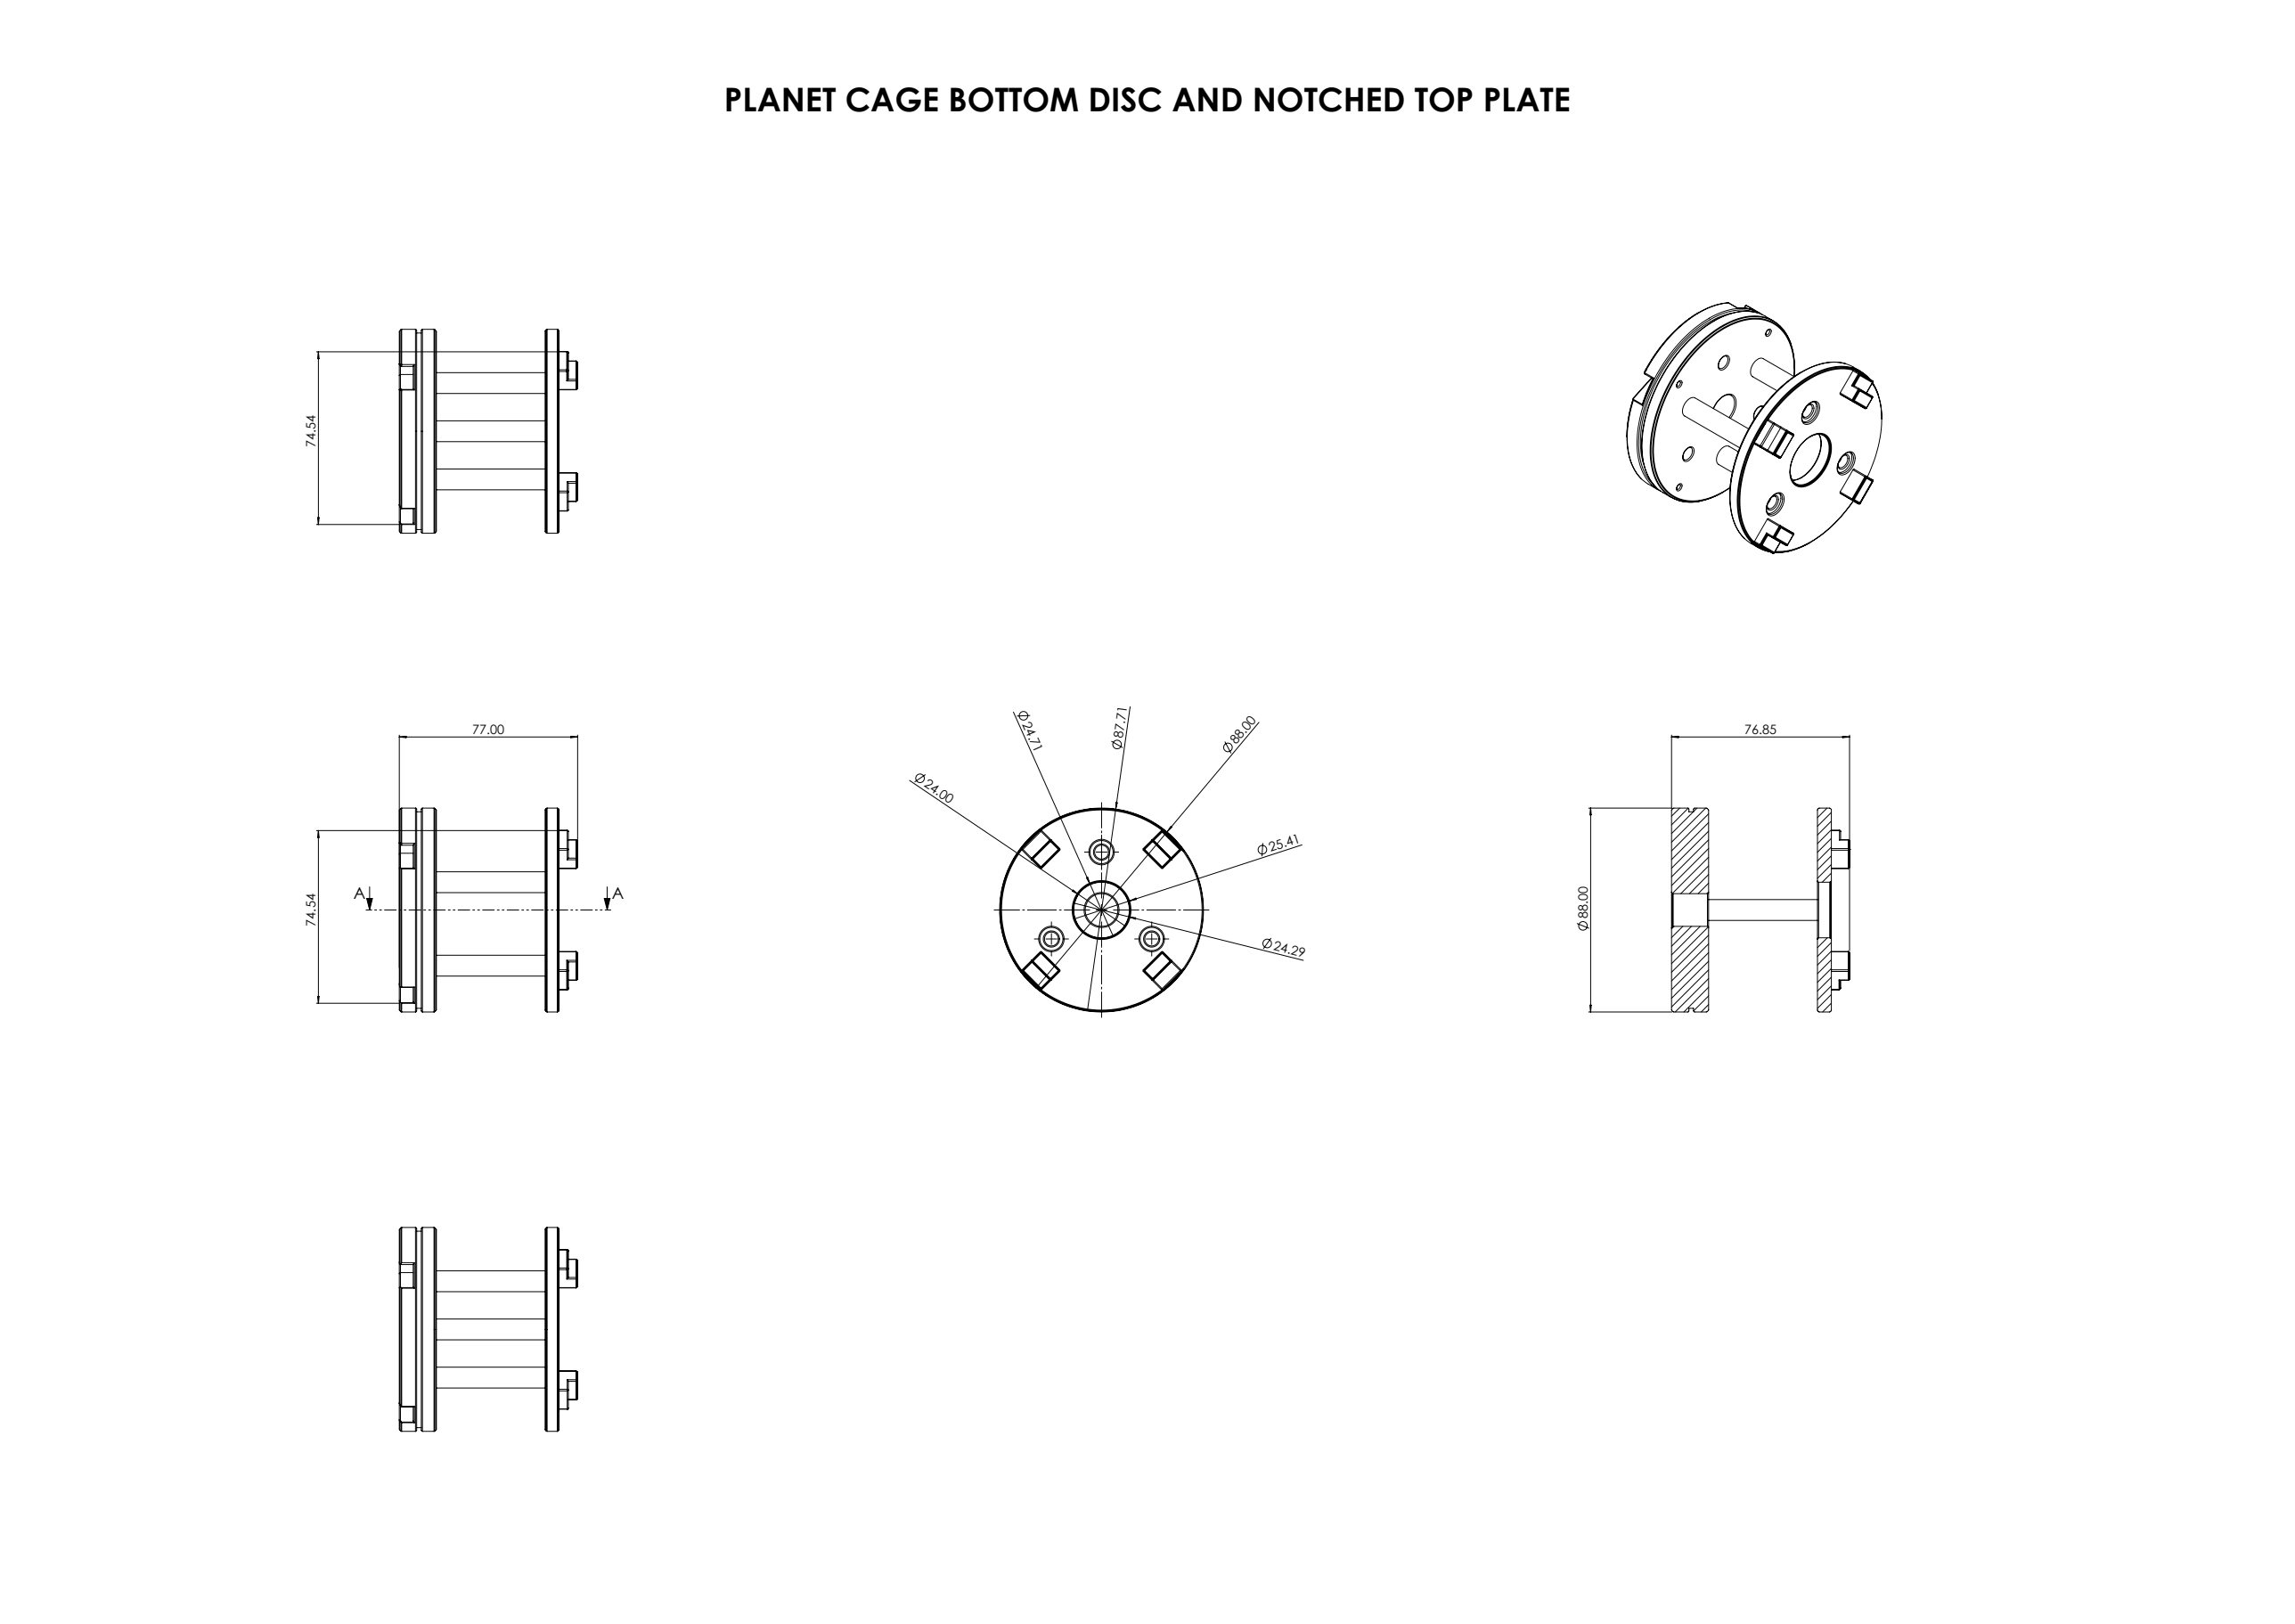
ISO-10303-21;
HEADER;
/* Generated by software containing ST-Developer
 * from STEP Tools, Inc. (www.steptools.com) 
 */

FILE_DESCRIPTION(
/* description */ (''),
/* implementation_level */ '2;1');

FILE_NAME(
/* name */ '02_Planet_Cage_Bottom_Disc_and_Notched_Top_Plate.step',
/* time_stamp */ '2026-10-11T13:00:10-07:00',
/* author */ (''),
/* organization */ (''),
/* preprocessor_version */ 'ST-DEVELOPER v20.2',
/* originating_system */ 'Autodesk Translation Framework v15.15.0.0',
/* authorisation */ '');

FILE_SCHEMA (('AUTOMOTIVE_DESIGN { 1 0 10303 214 3 1 1 }'));
ENDSEC;

DATA;
#10=MECHANICAL_DESIGN_GEOMETRIC_PRESENTATION_REPRESENTATION('',(#359),#65563);
#95=TOROIDAL_SURFACE('',#20843,43.5,0.5);
#96=TOROIDAL_SURFACE('',#20862,3.5,0.5);
#97=TOROIDAL_SURFACE('',#20886,42.9928932188135,0.5);
#98=TOROIDAL_SURFACE('',#20891,43.5,0.5);
#99=TOROIDAL_SURFACE('',#20897,3.5,0.5);
#100=TOROIDAL_SURFACE('',#20902,42.9928932188135,0.5);
#101=TOROIDAL_SURFACE('',#20905,42.9928932188135,0.5);
#102=TOROIDAL_SURFACE('',#20926,43.5,0.5);
#103=TOROIDAL_SURFACE('',#20929,43.5,0.5);
#104=TOROIDAL_SURFACE('',#20951,43.5,0.5);
#105=TOROIDAL_SURFACE('',#20956,43.5,0.5);
#106=TOROIDAL_SURFACE('',#20967,42.9928932188135,0.5);
#107=TOROIDAL_SURFACE('',#20971,3.5,0.5);
#108=TOROIDAL_SURFACE('',#20981,3.5,0.5);
#109=TOROIDAL_SURFACE('',#20985,1.75,0.5);
#110=TOROIDAL_SURFACE('',#21020,43.5,0.5);
#111=TOROIDAL_SURFACE('',#21025,1.75,0.5);
#112=TOROIDAL_SURFACE('',#21059,43.5,0.5);
#113=TOROIDAL_SURFACE('',#21069,43.5,0.5);
#114=TOROIDAL_SURFACE('',#21076,43.5,0.5);
#115=TOROIDAL_SURFACE('',#21081,43.5,0.5);
#116=TOROIDAL_SURFACE('',#21097,1.75,0.5);
#117=TOROIDAL_SURFACE('',#21103,1.75,0.5);
#118=TOROIDAL_SURFACE('',#21109,3.5,0.5);
#119=TOROIDAL_SURFACE('',#21128,3.5,0.5);
#120=TOROIDAL_SURFACE('',#21134,42.9928932188134,0.5);
#121=TOROIDAL_SURFACE('',#21136,1.75,0.5);
#122=TOROIDAL_SURFACE('',#21138,1.75,0.5);
#123=TOROIDAL_SURFACE('',#21140,3.5,0.5);
#124=TOROIDAL_SURFACE('',#21146,1.75,0.5);
#125=TOROIDAL_SURFACE('',#21148,1.75,0.5);
#126=TOROIDAL_SURFACE('',#21150,3.5,0.5);
#127=TOROIDAL_SURFACE('',#21158,3.5,0.5);
#128=TOROIDAL_SURFACE('',#21166,3.5,0.5);
#129=TOROIDAL_SURFACE('',#21183,43.5,0.5);
#130=TOROIDAL_SURFACE('',#21195,43.1928932188135,0.5);
#131=TOROIDAL_SURFACE('',#21206,3.5,0.5);
#132=TOROIDAL_SURFACE('',#21208,3.5,0.5);
#133=TOROIDAL_SURFACE('',#21210,3.5,0.5);
#134=TOROIDAL_SURFACE('',#21212,7.55,0.5);
#135=TOROIDAL_SURFACE('',#21219,7.75710678118654,0.5);
#136=TOROIDAL_SURFACE('',#21226,7.55,0.5);
#137=TOROIDAL_SURFACE('',#21228,12.5,0.5);
#138=TOROIDAL_SURFACE('',#21235,43.5,0.5);
#139=TOROIDAL_SURFACE('',#21243,43.1928932188135,0.5);
#140=TOROIDAL_SURFACE('',#21251,5.5,0.5);
#141=TOROIDAL_SURFACE('',#21261,5.5,0.5);
#142=TOROIDAL_SURFACE('',#21266,5.5,0.5);
#143=TOROIDAL_SURFACE('',#21271,12.5,0.5);
#144=TOROIDAL_SURFACE('',#21278,12.7071067811865,0.5);
#200=ELLIPSE('',#20602,0.707106781186548,0.5);
#201=ELLIPSE('',#20603,0.707106781186549,0.5);
#202=ELLIPSE('',#20642,0.707106781186549,0.5);
#203=ELLIPSE('',#20643,0.707106781186543,0.5);
#204=ELLIPSE('',#20698,0.707106781186547,0.5);
#205=ELLIPSE('',#20715,0.707106781186547,0.5);
#206=ELLIPSE('',#20745,1.08766387358053,0.5);
#207=ELLIPSE('',#20747,0.563016250305246,0.5);
#208=ELLIPSE('',#20752,0.70710678118655,0.499999999999999);
#209=ELLIPSE('',#20753,0.707106781186547,0.5);
#210=ELLIPSE('',#20756,0.707106781186549,0.5);
#211=ELLIPSE('',#20759,0.707106781186548,0.5);
#212=ELLIPSE('',#20790,0.524647623275289,0.499999999999999);
#213=ELLIPSE('',#20791,1.08766387358054,0.499999999999999);
#214=ELLIPSE('',#20799,0.541196100146196,0.5);
#215=ELLIPSE('',#20808,0.707106781186548,0.5);
#216=ELLIPSE('',#20818,0.541196100146196,0.5);
#217=ELLIPSE('',#20819,0.707106781186546,0.5);
#218=ELLIPSE('',#20822,0.999999999999998,0.499999999999999);
#219=ELLIPSE('',#20832,0.707106781186548,0.5);
#220=ELLIPSE('',#20901,0.707106781186546,0.5);
#221=ELLIPSE('',#20996,0.707106781186545,0.5);
#222=ELLIPSE('',#21001,0.563016250305243,0.5);
#223=ELLIPSE('',#21002,0.563016250305246,0.5);
#224=ELLIPSE('',#21003,0.707106781186547,0.5);
#225=ELLIPSE('',#21004,0.707106781186543,0.5);
#226=ELLIPSE('',#21007,0.563016250305245,0.499999999999997);
#227=ELLIPSE('',#21010,0.563016250305245,0.499999999999999);
#228=ELLIPSE('',#21017,0.999999999999989,0.499999999999997);
#229=ELLIPSE('',#21019,0.707106781186552,0.5);
#230=ELLIPSE('',#21057,0.707106781186546,0.5);
#231=ELLIPSE('',#21087,0.541196100146194,0.5);
#232=ELLIPSE('',#21096,0.707106781186549,0.5);
#243=SPHERICAL_SURFACE('',#20559,0.5);
#244=SPHERICAL_SURFACE('',#20569,0.5);
#245=SPHERICAL_SURFACE('',#20571,0.5);
#246=SPHERICAL_SURFACE('',#20581,0.5);
#247=SPHERICAL_SURFACE('',#20595,0.5);
#248=SPHERICAL_SURFACE('',#20605,0.5);
#249=SPHERICAL_SURFACE('',#20612,0.5);
#250=SPHERICAL_SURFACE('',#20617,0.5);
#251=SPHERICAL_SURFACE('',#20631,0.5);
#252=SPHERICAL_SURFACE('',#20637,0.5);
#253=SPHERICAL_SURFACE('',#20646,0.5);
#254=SPHERICAL_SURFACE('',#20654,0.5);
#255=SPHERICAL_SURFACE('',#20665,0.5);
#256=SPHERICAL_SURFACE('',#20674,0.5);
#257=SPHERICAL_SURFACE('',#20679,0.5);
#258=SPHERICAL_SURFACE('',#20683,0.5);
#259=SPHERICAL_SURFACE('',#20702,0.5);
#260=SPHERICAL_SURFACE('',#20708,0.5);
#261=SPHERICAL_SURFACE('',#20722,0.5);
#262=SPHERICAL_SURFACE('',#20726,0.5);
#263=SPHERICAL_SURFACE('',#20732,0.5);
#264=SPHERICAL_SURFACE('',#20737,0.5);
#265=SPHERICAL_SURFACE('',#20748,0.5);
#266=SPHERICAL_SURFACE('',#20764,0.5);
#267=SPHERICAL_SURFACE('',#20768,0.5);
#268=SPHERICAL_SURFACE('',#20784,0.5);
#269=SPHERICAL_SURFACE('',#20787,0.5);
#270=SPHERICAL_SURFACE('',#20809,0.5);
#271=SPHERICAL_SURFACE('',#20824,0.5);
#272=SPHERICAL_SURFACE('',#20827,0.5);
#273=SPHERICAL_SURFACE('',#20836,0.5);
#274=SPHERICAL_SURFACE('',#20841,0.5);
#275=SPHERICAL_SURFACE('',#20868,0.5);
#276=SPHERICAL_SURFACE('',#20871,0.5);
#277=SPHERICAL_SURFACE('',#20914,0.5);
#278=SPHERICAL_SURFACE('',#20920,0.5);
#279=SPHERICAL_SURFACE('',#20934,0.5);
#280=SPHERICAL_SURFACE('',#20936,0.5);
#281=SPHERICAL_SURFACE('',#20946,0.5);
#282=SPHERICAL_SURFACE('',#20949,0.5);
#283=SPHERICAL_SURFACE('',#20961,0.500000000000003);
#284=SPHERICAL_SURFACE('',#20975,0.5);
#285=SPHERICAL_SURFACE('',#20991,0.5);
#286=SPHERICAL_SURFACE('',#21034,0.5);
#287=SPHERICAL_SURFACE('',#21038,0.5);
#288=SPHERICAL_SURFACE('',#21042,0.5);
#289=SPHERICAL_SURFACE('',#21053,0.5);
#290=SPHERICAL_SURFACE('',#21092,0.5);
#291=SPHERICAL_SURFACE('',#21178,0.5);
#337=SHAPE_REPRESENTATION_RELATIONSHIP('SRR','None',#65615,#348);
#348=ADVANCED_BREP_SHAPE_REPRESENTATION('',(#370),#65553);
#359=STYLED_ITEM('',(#65802),#370);
#370=MANIFOLD_SOLID_BREP('Body1',#20009);
#414=CONICAL_SURFACE('',#20889,43.6,0.785398163397448);
#415=CONICAL_SURFACE('',#20908,43.6,0.785398163397448);
#416=CONICAL_SURFACE('',#20924,43.6,0.785398163397448);
#417=CONICAL_SURFACE('',#20954,43.6,0.785398163397448);
#418=CONICAL_SURFACE('',#21073,43.6,0.785398163397454);
#419=CONICAL_SURFACE('',#21189,43.7,0.785398163397452);
#420=CONICAL_SURFACE('',#21223,7.3,0.785398163397442);
#421=CONICAL_SURFACE('',#21239,43.7,0.785398163397452);
#422=CONICAL_SURFACE('',#21275,12.25,0.785398163397448);
#668=(
BOUNDED_CURVE()
B_SPLINE_CURVE(2,(#48216,#48217,#48218),.UNSPECIFIED.,.F.,.F.)
B_SPLINE_CURVE_WITH_KNOTS((3,3),(0.026389951333147,0.0542823820564139),
 .UNSPECIFIED.)
CURVE()
GEOMETRIC_REPRESENTATION_ITEM()
RATIONAL_B_SPLINE_CURVE((1.00002935554076,1.00004146705942,1.00004638738564))
REPRESENTATION_ITEM('')
);
#669=(
BOUNDED_CURVE()
B_SPLINE_CURVE(2,(#48349,#48350,#48351),.UNSPECIFIED.,.F.,.F.)
B_SPLINE_CURVE_WITH_KNOTS((3,3),(0.0263899513331846,0.0542823820564278),
 .UNSPECIFIED.)
CURVE()
GEOMETRIC_REPRESENTATION_ITEM()
RATIONAL_B_SPLINE_CURVE((1.00002935553973,1.00004146705796,1.00004638738401))
REPRESENTATION_ITEM('')
);
#670=(
BOUNDED_CURVE()
B_SPLINE_CURVE(2,(#49013,#49014,#49015),.UNSPECIFIED.,.F.,.F.)
B_SPLINE_CURVE_WITH_KNOTS((3,3),(0.355039941373883,0.455385686797418),
 .UNSPECIFIED.)
CURVE()
GEOMETRIC_REPRESENTATION_ITEM()
RATIONAL_B_SPLINE_CURVE((1.00817025780825,1.00909081812274,1.00987909016891))
REPRESENTATION_ITEM('')
);
#671=(
BOUNDED_CURVE()
B_SPLINE_CURVE(2,(#49128,#49129,#49130),.UNSPECIFIED.,.F.,.F.)
B_SPLINE_CURVE_WITH_KNOTS((3,3),(1.65125508748907,1.7516008329126),
 .UNSPECIFIED.)
CURVE()
GEOMETRIC_REPRESENTATION_ITEM()
RATIONAL_B_SPLINE_CURVE((1.00987909016891,1.00909081812274,1.00817025780825))
REPRESENTATION_ITEM('')
);
#838=B_SPLINE_SURFACE_WITH_KNOTS('',3,3,((#48066,#48067,#48068,#48069),
(#48070,#48071,#48072,#48073),(#48074,#48075,#48076,#48077),(#48078,#48079,
#48080,#48081),(#48082,#48083,#48084,#48085),(#48086,#48087,#48088,#48089),
(#48090,#48091,#48092,#48093)),.UNSPECIFIED.,.F.,.F.,.F.,(4,1,1,1,4),(4,
4),(0.,0.285714285714286,0.571428571428571,0.857142857142857,1.),(0.363335998515663,
0.499634934734419),.UNSPECIFIED.);
#839=B_SPLINE_SURFACE_WITH_KNOTS('',3,3,((#48278,#48279,#48280,#48281),
(#48282,#48283,#48284,#48285),(#48286,#48287,#48288,#48289),(#48290,#48291,
#48292,#48293),(#48294,#48295,#48296,#48297),(#48298,#48299,#48300,#48301),
(#48302,#48303,#48304,#48305)),.UNSPECIFIED.,.F.,.F.,.F.,(4,1,1,1,4),(4,
4),(0.,0.285714285714286,0.571428571428571,0.857142857142857,1.),(0.,0.136299039595008),
 .UNSPECIFIED.);
#840=B_SPLINE_SURFACE_WITH_KNOTS('',3,3,((#48415,#48416,#48417,#48418),
(#48419,#48420,#48421,#48422),(#48423,#48424,#48425,#48426),(#48427,#48428,
#48429,#48430)),.UNSPECIFIED.,.F.,.F.,.F.,(4,4),(4,4),(0.,1.),(0.,0.0923903836946144),
 .UNSPECIFIED.);
#841=B_SPLINE_SURFACE_WITH_KNOTS('',3,3,((#48482,#48483,#48484,#48485),
(#48486,#48487,#48488,#48489),(#48490,#48491,#48492,#48493),(#48494,#48495,
#48496,#48497)),.UNSPECIFIED.,.F.,.F.,.F.,(4,4),(4,4),(0.,1.),(0.,0.0923903843306348),
 .UNSPECIFIED.);
#842=B_SPLINE_SURFACE_WITH_KNOTS('',3,3,((#48548,#48549,#48550,#48551),
(#48552,#48553,#48554,#48555),(#48556,#48557,#48558,#48559),(#48560,#48561,
#48562,#48563),(#48564,#48565,#48566,#48567),(#48568,#48569,#48570,#48571),
(#48572,#48573,#48574,#48575)),.UNSPECIFIED.,.F.,.F.,.F.,(4,1,1,1,4),(4,
4),(0.,0.285714285714286,0.571428571428571,0.857142857142857,1.),(0.,0.136298877173929),
 .UNSPECIFIED.);
#893=PLANE('',#20585);
#894=PLANE('',#20588);
#895=PLANE('',#20591);
#896=PLANE('',#20597);
#897=PLANE('',#20600);
#898=PLANE('',#20607);
#899=PLANE('',#20616);
#900=PLANE('',#20633);
#901=PLANE('',#20636);
#902=PLANE('',#20640);
#903=PLANE('',#20650);
#904=PLANE('',#20651);
#905=PLANE('',#20658);
#906=PLANE('',#20669);
#907=PLANE('',#20670);
#908=PLANE('',#20687);
#909=PLANE('',#20690);
#910=PLANE('',#20693);
#911=PLANE('',#20704);
#912=PLANE('',#20707);
#913=PLANE('',#20711);
#914=PLANE('',#20727);
#915=PLANE('',#20728);
#916=PLANE('',#20736);
#917=PLANE('',#20750);
#918=PLANE('',#20754);
#919=PLANE('',#20778);
#920=PLANE('',#20794);
#921=PLANE('',#20797);
#922=PLANE('',#20802);
#923=PLANE('',#20805);
#924=PLANE('',#20813);
#925=PLANE('',#20815);
#926=PLANE('',#20816);
#927=PLANE('',#20820);
#928=PLANE('',#20831);
#929=PLANE('',#20842);
#930=PLANE('',#20858);
#931=PLANE('',#20877);
#932=PLANE('',#20907);
#933=PLANE('',#20923);
#934=PLANE('',#20928);
#935=PLANE('',#20931);
#936=PLANE('',#20940);
#937=PLANE('',#20958);
#938=PLANE('',#20977);
#939=PLANE('',#20978);
#940=PLANE('',#20997);
#941=PLANE('',#21008);
#942=PLANE('',#21015);
#943=PLANE('',#21016);
#944=PLANE('',#21022);
#945=PLANE('',#21048);
#946=PLANE('',#21055);
#947=PLANE('',#21058);
#948=PLANE('',#21067);
#949=PLANE('',#21078);
#950=PLANE('',#21083);
#951=PLANE('',#21089);
#952=PLANE('',#21094);
#953=PLANE('',#21114);
#954=PLANE('',#21156);
#955=PLANE('',#21164);
#956=PLANE('',#21172);
#957=PLANE('',#21180);
#958=PLANE('',#21198);
#959=PLANE('',#21256);
#960=PLANE('',#21280);
#961=PLANE('',#21284);
#962=PLANE('',#21285);
#963=PLANE('',#21286);
#964=PLANE('',#21287);
#965=PLANE('',#21288);
#966=PLANE('',#21289);
#967=PLANE('',#21290);
#968=PLANE('',#21291);
#969=PLANE('',#21292);
#970=PLANE('',#21293);
#1083=FACE_BOUND('',#2757,.T.);
#1084=FACE_BOUND('',#2765,.T.);
#1085=FACE_BOUND('',#2804,.T.);
#1086=FACE_BOUND('',#2834,.T.);
#1087=FACE_BOUND('',#2854,.T.);
#1088=FACE_BOUND('',#2859,.T.);
#1089=FACE_BOUND('',#2862,.T.);
#1090=FACE_BOUND('',#2876,.T.);
#1091=FACE_BOUND('',#2877,.T.);
#1092=FACE_BOUND('',#2878,.T.);
#1093=FACE_BOUND('',#2879,.T.);
#1094=FACE_BOUND('',#2880,.T.);
#1095=FACE_BOUND('',#2881,.T.);
#1096=FACE_BOUND('',#2882,.T.);
#1097=FACE_BOUND('',#2883,.T.);
#1098=FACE_BOUND('',#2884,.T.);
#1099=FACE_BOUND('',#2885,.T.);
#1100=FACE_BOUND('',#2886,.T.);
#1101=FACE_BOUND('',#2900,.T.);
#1102=FACE_BOUND('',#2904,.T.);
#1103=FACE_BOUND('',#2908,.T.);
#1104=FACE_BOUND('',#2919,.T.);
#1105=FACE_BOUND('',#2920,.T.);
#1106=FACE_BOUND('',#2921,.T.);
#1107=FACE_BOUND('',#2922,.T.);
#1108=FACE_BOUND('',#2923,.T.);
#1109=FACE_BOUND('',#2924,.T.);
#1110=FACE_BOUND('',#2925,.T.);
#1111=FACE_BOUND('',#2941,.T.);
#1112=FACE_BOUND('',#2942,.T.);
#1113=FACE_BOUND('',#2943,.T.);
#1114=FACE_BOUND('',#2944,.T.);
#1425=FACE_OUTER_BOUND('',#2612,.T.);
#1426=FACE_OUTER_BOUND('',#2613,.T.);
#1427=FACE_OUTER_BOUND('',#2614,.T.);
#1428=FACE_OUTER_BOUND('',#2615,.T.);
#1429=FACE_OUTER_BOUND('',#2616,.T.);
#1430=FACE_OUTER_BOUND('',#2617,.T.);
#1431=FACE_OUTER_BOUND('',#2618,.T.);
#1432=FACE_OUTER_BOUND('',#2619,.T.);
#1433=FACE_OUTER_BOUND('',#2620,.T.);
#1434=FACE_OUTER_BOUND('',#2621,.T.);
#1435=FACE_OUTER_BOUND('',#2622,.T.);
#1436=FACE_OUTER_BOUND('',#2623,.T.);
#1437=FACE_OUTER_BOUND('',#2624,.T.);
#1438=FACE_OUTER_BOUND('',#2625,.T.);
#1439=FACE_OUTER_BOUND('',#2626,.T.);
#1440=FACE_OUTER_BOUND('',#2627,.T.);
#1441=FACE_OUTER_BOUND('',#2628,.T.);
#1442=FACE_OUTER_BOUND('',#2629,.T.);
#1443=FACE_OUTER_BOUND('',#2630,.T.);
#1444=FACE_OUTER_BOUND('',#2631,.T.);
#1445=FACE_OUTER_BOUND('',#2632,.T.);
#1446=FACE_OUTER_BOUND('',#2633,.T.);
#1447=FACE_OUTER_BOUND('',#2634,.T.);
#1448=FACE_OUTER_BOUND('',#2635,.T.);
#1449=FACE_OUTER_BOUND('',#2636,.T.);
#1450=FACE_OUTER_BOUND('',#2637,.T.);
#1451=FACE_OUTER_BOUND('',#2638,.T.);
#1452=FACE_OUTER_BOUND('',#2639,.T.);
#1453=FACE_OUTER_BOUND('',#2640,.T.);
#1454=FACE_OUTER_BOUND('',#2641,.T.);
#1455=FACE_OUTER_BOUND('',#2642,.T.);
#1456=FACE_OUTER_BOUND('',#2643,.T.);
#1457=FACE_OUTER_BOUND('',#2644,.T.);
#1458=FACE_OUTER_BOUND('',#2645,.T.);
#1459=FACE_OUTER_BOUND('',#2646,.T.);
#1460=FACE_OUTER_BOUND('',#2647,.T.);
#1461=FACE_OUTER_BOUND('',#2648,.T.);
#1462=FACE_OUTER_BOUND('',#2649,.T.);
#1463=FACE_OUTER_BOUND('',#2650,.T.);
#1464=FACE_OUTER_BOUND('',#2651,.T.);
#1465=FACE_OUTER_BOUND('',#2652,.T.);
#1466=FACE_OUTER_BOUND('',#2653,.T.);
#1467=FACE_OUTER_BOUND('',#2654,.T.);
#1468=FACE_OUTER_BOUND('',#2655,.T.);
#1469=FACE_OUTER_BOUND('',#2656,.T.);
#1470=FACE_OUTER_BOUND('',#2657,.T.);
#1471=FACE_OUTER_BOUND('',#2658,.T.);
#1472=FACE_OUTER_BOUND('',#2659,.T.);
#1473=FACE_OUTER_BOUND('',#2660,.T.);
#1474=FACE_OUTER_BOUND('',#2661,.T.);
#1475=FACE_OUTER_BOUND('',#2662,.T.);
#1476=FACE_OUTER_BOUND('',#2663,.T.);
#1477=FACE_OUTER_BOUND('',#2664,.T.);
#1478=FACE_OUTER_BOUND('',#2665,.T.);
#1479=FACE_OUTER_BOUND('',#2666,.T.);
#1480=FACE_OUTER_BOUND('',#2667,.T.);
#1481=FACE_OUTER_BOUND('',#2668,.T.);
#1482=FACE_OUTER_BOUND('',#2669,.T.);
#1483=FACE_OUTER_BOUND('',#2670,.T.);
#1484=FACE_OUTER_BOUND('',#2671,.T.);
#1485=FACE_OUTER_BOUND('',#2672,.T.);
#1486=FACE_OUTER_BOUND('',#2673,.T.);
#1487=FACE_OUTER_BOUND('',#2674,.T.);
#1488=FACE_OUTER_BOUND('',#2675,.T.);
#1489=FACE_OUTER_BOUND('',#2676,.T.);
#1490=FACE_OUTER_BOUND('',#2677,.T.);
#1491=FACE_OUTER_BOUND('',#2678,.T.);
#1492=FACE_OUTER_BOUND('',#2679,.T.);
#1493=FACE_OUTER_BOUND('',#2680,.T.);
#1494=FACE_OUTER_BOUND('',#2681,.T.);
#1495=FACE_OUTER_BOUND('',#2682,.T.);
#1496=FACE_OUTER_BOUND('',#2683,.T.);
#1497=FACE_OUTER_BOUND('',#2684,.T.);
#1498=FACE_OUTER_BOUND('',#2685,.T.);
#1499=FACE_OUTER_BOUND('',#2686,.T.);
#1500=FACE_OUTER_BOUND('',#2687,.T.);
#1501=FACE_OUTER_BOUND('',#2688,.T.);
#1502=FACE_OUTER_BOUND('',#2689,.T.);
#1503=FACE_OUTER_BOUND('',#2690,.T.);
#1504=FACE_OUTER_BOUND('',#2691,.T.);
#1505=FACE_OUTER_BOUND('',#2692,.T.);
#1506=FACE_OUTER_BOUND('',#2693,.T.);
#1507=FACE_OUTER_BOUND('',#2694,.T.);
#1508=FACE_OUTER_BOUND('',#2695,.T.);
#1509=FACE_OUTER_BOUND('',#2696,.T.);
#1510=FACE_OUTER_BOUND('',#2697,.T.);
#1511=FACE_OUTER_BOUND('',#2698,.T.);
#1512=FACE_OUTER_BOUND('',#2699,.T.);
#1513=FACE_OUTER_BOUND('',#2700,.T.);
#1514=FACE_OUTER_BOUND('',#2701,.T.);
#1515=FACE_OUTER_BOUND('',#2702,.T.);
#1516=FACE_OUTER_BOUND('',#2703,.T.);
#1517=FACE_OUTER_BOUND('',#2704,.T.);
#1518=FACE_OUTER_BOUND('',#2705,.T.);
#1519=FACE_OUTER_BOUND('',#2706,.T.);
#1520=FACE_OUTER_BOUND('',#2707,.T.);
#1521=FACE_OUTER_BOUND('',#2708,.T.);
#1522=FACE_OUTER_BOUND('',#2709,.T.);
#1523=FACE_OUTER_BOUND('',#2710,.T.);
#1524=FACE_OUTER_BOUND('',#2711,.T.);
#1525=FACE_OUTER_BOUND('',#2712,.T.);
#1526=FACE_OUTER_BOUND('',#2713,.T.);
#1527=FACE_OUTER_BOUND('',#2714,.T.);
#1528=FACE_OUTER_BOUND('',#2715,.T.);
#1529=FACE_OUTER_BOUND('',#2716,.T.);
#1530=FACE_OUTER_BOUND('',#2717,.T.);
#1531=FACE_OUTER_BOUND('',#2718,.T.);
#1532=FACE_OUTER_BOUND('',#2719,.T.);
#1533=FACE_OUTER_BOUND('',#2720,.T.);
#1534=FACE_OUTER_BOUND('',#2721,.T.);
#1535=FACE_OUTER_BOUND('',#2722,.T.);
#1536=FACE_OUTER_BOUND('',#2723,.T.);
#1537=FACE_OUTER_BOUND('',#2724,.T.);
#1538=FACE_OUTER_BOUND('',#2725,.T.);
#1539=FACE_OUTER_BOUND('',#2726,.T.);
#1540=FACE_OUTER_BOUND('',#2727,.T.);
#1541=FACE_OUTER_BOUND('',#2728,.T.);
#1542=FACE_OUTER_BOUND('',#2729,.T.);
#1543=FACE_OUTER_BOUND('',#2730,.T.);
#1544=FACE_OUTER_BOUND('',#2731,.T.);
#1545=FACE_OUTER_BOUND('',#2732,.T.);
#1546=FACE_OUTER_BOUND('',#2733,.T.);
#1547=FACE_OUTER_BOUND('',#2734,.T.);
#1548=FACE_OUTER_BOUND('',#2735,.T.);
#1549=FACE_OUTER_BOUND('',#2736,.T.);
#1550=FACE_OUTER_BOUND('',#2737,.T.);
#1551=FACE_OUTER_BOUND('',#2738,.T.);
#1552=FACE_OUTER_BOUND('',#2739,.T.);
#1553=FACE_OUTER_BOUND('',#2740,.T.);
#1554=FACE_OUTER_BOUND('',#2741,.T.);
#1555=FACE_OUTER_BOUND('',#2742,.T.);
#1556=FACE_OUTER_BOUND('',#2743,.T.);
#1557=FACE_OUTER_BOUND('',#2744,.T.);
#1558=FACE_OUTER_BOUND('',#2745,.T.);
#1559=FACE_OUTER_BOUND('',#2746,.T.);
#1560=FACE_OUTER_BOUND('',#2747,.T.);
#1561=FACE_OUTER_BOUND('',#2748,.T.);
#1562=FACE_OUTER_BOUND('',#2749,.T.);
#1563=FACE_OUTER_BOUND('',#2750,.T.);
#1564=FACE_OUTER_BOUND('',#2751,.T.);
#1565=FACE_OUTER_BOUND('',#2752,.T.);
#1566=FACE_OUTER_BOUND('',#2753,.T.);
#1567=FACE_OUTER_BOUND('',#2754,.T.);
#1568=FACE_OUTER_BOUND('',#2755,.T.);
#1569=FACE_OUTER_BOUND('',#2756,.T.);
#1570=FACE_OUTER_BOUND('',#2758,.T.);
#1571=FACE_OUTER_BOUND('',#2759,.T.);
#1572=FACE_OUTER_BOUND('',#2760,.T.);
#1573=FACE_OUTER_BOUND('',#2761,.T.);
#1574=FACE_OUTER_BOUND('',#2762,.T.);
#1575=FACE_OUTER_BOUND('',#2763,.T.);
#1576=FACE_OUTER_BOUND('',#2764,.T.);
#1577=FACE_OUTER_BOUND('',#2766,.T.);
#1578=FACE_OUTER_BOUND('',#2767,.T.);
#1579=FACE_OUTER_BOUND('',#2768,.T.);
#1580=FACE_OUTER_BOUND('',#2769,.T.);
#1581=FACE_OUTER_BOUND('',#2770,.T.);
#1582=FACE_OUTER_BOUND('',#2771,.T.);
#1583=FACE_OUTER_BOUND('',#2772,.T.);
#1584=FACE_OUTER_BOUND('',#2773,.T.);
#1585=FACE_OUTER_BOUND('',#2774,.T.);
#1586=FACE_OUTER_BOUND('',#2775,.T.);
#1587=FACE_OUTER_BOUND('',#2776,.T.);
#1588=FACE_OUTER_BOUND('',#2777,.T.);
#1589=FACE_OUTER_BOUND('',#2778,.T.);
#1590=FACE_OUTER_BOUND('',#2779,.T.);
#1591=FACE_OUTER_BOUND('',#2780,.T.);
#1592=FACE_OUTER_BOUND('',#2781,.T.);
#1593=FACE_OUTER_BOUND('',#2782,.T.);
#1594=FACE_OUTER_BOUND('',#2783,.T.);
#1595=FACE_OUTER_BOUND('',#2784,.T.);
#1596=FACE_OUTER_BOUND('',#2785,.T.);
#1597=FACE_OUTER_BOUND('',#2786,.T.);
#1598=FACE_OUTER_BOUND('',#2787,.T.);
#1599=FACE_OUTER_BOUND('',#2788,.T.);
#1600=FACE_OUTER_BOUND('',#2789,.T.);
#1601=FACE_OUTER_BOUND('',#2790,.T.);
#1602=FACE_OUTER_BOUND('',#2791,.T.);
#1603=FACE_OUTER_BOUND('',#2792,.T.);
#1604=FACE_OUTER_BOUND('',#2793,.T.);
#1605=FACE_OUTER_BOUND('',#2794,.T.);
#1606=FACE_OUTER_BOUND('',#2795,.T.);
#1607=FACE_OUTER_BOUND('',#2796,.T.);
#1608=FACE_OUTER_BOUND('',#2797,.T.);
#1609=FACE_OUTER_BOUND('',#2798,.T.);
#1610=FACE_OUTER_BOUND('',#2799,.T.);
#1611=FACE_OUTER_BOUND('',#2800,.T.);
#1612=FACE_OUTER_BOUND('',#2801,.T.);
#1613=FACE_OUTER_BOUND('',#2802,.T.);
#1614=FACE_OUTER_BOUND('',#2803,.T.);
#1615=FACE_OUTER_BOUND('',#2805,.T.);
#1616=FACE_OUTER_BOUND('',#2806,.T.);
#1617=FACE_OUTER_BOUND('',#2807,.T.);
#1618=FACE_OUTER_BOUND('',#2808,.T.);
#1619=FACE_OUTER_BOUND('',#2809,.T.);
#1620=FACE_OUTER_BOUND('',#2810,.T.);
#1621=FACE_OUTER_BOUND('',#2811,.T.);
#1622=FACE_OUTER_BOUND('',#2812,.T.);
#1623=FACE_OUTER_BOUND('',#2813,.T.);
#1624=FACE_OUTER_BOUND('',#2814,.T.);
#1625=FACE_OUTER_BOUND('',#2815,.T.);
#1626=FACE_OUTER_BOUND('',#2816,.T.);
#1627=FACE_OUTER_BOUND('',#2817,.T.);
#1628=FACE_OUTER_BOUND('',#2818,.T.);
#1629=FACE_OUTER_BOUND('',#2819,.T.);
#1630=FACE_OUTER_BOUND('',#2820,.T.);
#1631=FACE_OUTER_BOUND('',#2821,.T.);
#1632=FACE_OUTER_BOUND('',#2822,.T.);
#1633=FACE_OUTER_BOUND('',#2823,.T.);
#1634=FACE_OUTER_BOUND('',#2824,.T.);
#1635=FACE_OUTER_BOUND('',#2825,.T.);
#1636=FACE_OUTER_BOUND('',#2826,.T.);
#1637=FACE_OUTER_BOUND('',#2827,.T.);
#1638=FACE_OUTER_BOUND('',#2828,.T.);
#1639=FACE_OUTER_BOUND('',#2829,.T.);
#1640=FACE_OUTER_BOUND('',#2830,.T.);
#1641=FACE_OUTER_BOUND('',#2831,.T.);
#1642=FACE_OUTER_BOUND('',#2832,.T.);
#1643=FACE_OUTER_BOUND('',#2833,.T.);
#1644=FACE_OUTER_BOUND('',#2835,.T.);
#1645=FACE_OUTER_BOUND('',#2836,.T.);
#1646=FACE_OUTER_BOUND('',#2837,.T.);
#1647=FACE_OUTER_BOUND('',#2838,.T.);
#1648=FACE_OUTER_BOUND('',#2839,.T.);
#1649=FACE_OUTER_BOUND('',#2840,.T.);
#1650=FACE_OUTER_BOUND('',#2841,.T.);
#1651=FACE_OUTER_BOUND('',#2842,.T.);
#1652=FACE_OUTER_BOUND('',#2843,.T.);
#1653=FACE_OUTER_BOUND('',#2844,.T.);
#1654=FACE_OUTER_BOUND('',#2845,.T.);
#1655=FACE_OUTER_BOUND('',#2846,.T.);
#1656=FACE_OUTER_BOUND('',#2847,.T.);
#1657=FACE_OUTER_BOUND('',#2848,.T.);
#1658=FACE_OUTER_BOUND('',#2849,.T.);
#1659=FACE_OUTER_BOUND('',#2850,.T.);
#1660=FACE_OUTER_BOUND('',#2851,.T.);
#1661=FACE_OUTER_BOUND('',#2852,.T.);
#1662=FACE_OUTER_BOUND('',#2853,.T.);
#1663=FACE_OUTER_BOUND('',#2855,.T.);
#1664=FACE_OUTER_BOUND('',#2856,.T.);
#1665=FACE_OUTER_BOUND('',#2857,.T.);
#1666=FACE_OUTER_BOUND('',#2858,.T.);
#1667=FACE_OUTER_BOUND('',#2860,.T.);
#1668=FACE_OUTER_BOUND('',#2861,.T.);
#1669=FACE_OUTER_BOUND('',#2863,.T.);
#1670=FACE_OUTER_BOUND('',#2864,.T.);
#1671=FACE_OUTER_BOUND('',#2865,.T.);
#1672=FACE_OUTER_BOUND('',#2866,.T.);
#1673=FACE_OUTER_BOUND('',#2867,.T.);
#1674=FACE_OUTER_BOUND('',#2868,.T.);
#1675=FACE_OUTER_BOUND('',#2869,.T.);
#1676=FACE_OUTER_BOUND('',#2870,.T.);
#1677=FACE_OUTER_BOUND('',#2871,.T.);
#1678=FACE_OUTER_BOUND('',#2872,.T.);
#1679=FACE_OUTER_BOUND('',#2873,.T.);
#1680=FACE_OUTER_BOUND('',#2874,.T.);
#1681=FACE_OUTER_BOUND('',#2875,.T.);
#1682=FACE_OUTER_BOUND('',#2887,.T.);
#1683=FACE_OUTER_BOUND('',#2888,.T.);
#1684=FACE_OUTER_BOUND('',#2889,.T.);
#1685=FACE_OUTER_BOUND('',#2890,.T.);
#1686=FACE_OUTER_BOUND('',#2891,.T.);
#1687=FACE_OUTER_BOUND('',#2892,.T.);
#1688=FACE_OUTER_BOUND('',#2893,.T.);
#1689=FACE_OUTER_BOUND('',#2894,.T.);
#1690=FACE_OUTER_BOUND('',#2895,.T.);
#1691=FACE_OUTER_BOUND('',#2896,.T.);
#1692=FACE_OUTER_BOUND('',#2897,.T.);
#1693=FACE_OUTER_BOUND('',#2898,.T.);
#1694=FACE_OUTER_BOUND('',#2899,.T.);
#1695=FACE_OUTER_BOUND('',#2901,.T.);
#1696=FACE_OUTER_BOUND('',#2902,.T.);
#1697=FACE_OUTER_BOUND('',#2903,.T.);
#1698=FACE_OUTER_BOUND('',#2905,.T.);
#1699=FACE_OUTER_BOUND('',#2906,.T.);
#1700=FACE_OUTER_BOUND('',#2907,.T.);
#1701=FACE_OUTER_BOUND('',#2909,.T.);
#1702=FACE_OUTER_BOUND('',#2910,.T.);
#1703=FACE_OUTER_BOUND('',#2911,.T.);
#1704=FACE_OUTER_BOUND('',#2912,.T.);
#1705=FACE_OUTER_BOUND('',#2913,.T.);
#1706=FACE_OUTER_BOUND('',#2914,.T.);
#1707=FACE_OUTER_BOUND('',#2915,.T.);
#1708=FACE_OUTER_BOUND('',#2916,.T.);
#1709=FACE_OUTER_BOUND('',#2917,.T.);
#1710=FACE_OUTER_BOUND('',#2918,.T.);
#1711=FACE_OUTER_BOUND('',#2926,.T.);
#1712=FACE_OUTER_BOUND('',#2927,.T.);
#1713=FACE_OUTER_BOUND('',#2928,.T.);
#1714=FACE_OUTER_BOUND('',#2929,.T.);
#1715=FACE_OUTER_BOUND('',#2930,.T.);
#1716=FACE_OUTER_BOUND('',#2931,.T.);
#1717=FACE_OUTER_BOUND('',#2932,.T.);
#1718=FACE_OUTER_BOUND('',#2933,.T.);
#1719=FACE_OUTER_BOUND('',#2934,.T.);
#1720=FACE_OUTER_BOUND('',#2935,.T.);
#1721=FACE_OUTER_BOUND('',#2936,.T.);
#1722=FACE_OUTER_BOUND('',#2937,.T.);
#1723=FACE_OUTER_BOUND('',#2938,.T.);
#1724=FACE_OUTER_BOUND('',#2939,.T.);
#1725=FACE_OUTER_BOUND('',#2940,.T.);
#1726=FACE_OUTER_BOUND('',#2945,.T.);
#1727=FACE_OUTER_BOUND('',#2946,.T.);
#1728=FACE_OUTER_BOUND('',#2947,.T.);
#1729=FACE_OUTER_BOUND('',#2948,.T.);
#1730=FACE_OUTER_BOUND('',#2949,.T.);
#1731=FACE_OUTER_BOUND('',#2950,.T.);
#1732=FACE_OUTER_BOUND('',#2951,.T.);
#1733=FACE_OUTER_BOUND('',#2952,.T.);
#1734=FACE_OUTER_BOUND('',#2953,.T.);
#1735=FACE_OUTER_BOUND('',#2954,.T.);
#1736=FACE_OUTER_BOUND('',#2955,.T.);
#1737=FACE_OUTER_BOUND('',#2956,.T.);
#1738=FACE_OUTER_BOUND('',#2957,.T.);
#1739=FACE_OUTER_BOUND('',#2958,.T.);
#1740=FACE_OUTER_BOUND('',#2959,.T.);
#1741=FACE_OUTER_BOUND('',#2960,.T.);
#1742=FACE_OUTER_BOUND('',#2961,.T.);
#1743=FACE_OUTER_BOUND('',#2962,.T.);
#1744=FACE_OUTER_BOUND('',#2963,.T.);
#1745=FACE_OUTER_BOUND('',#2964,.T.);
#1746=FACE_OUTER_BOUND('',#2965,.T.);
#1747=FACE_OUTER_BOUND('',#2966,.T.);
#1748=FACE_OUTER_BOUND('',#2967,.T.);
#1749=FACE_OUTER_BOUND('',#2968,.T.);
#1750=FACE_OUTER_BOUND('',#2969,.T.);
#1751=FACE_OUTER_BOUND('',#2970,.T.);
#2612=EDGE_LOOP('',(#13844,#13845,#13846,#13847));
#2613=EDGE_LOOP('',(#13848,#13849,#13850,#13851));
#2614=EDGE_LOOP('',(#13852,#13853,#13854,#13855));
#2615=EDGE_LOOP('',(#13856,#13857,#13858,#13859));
#2616=EDGE_LOOP('',(#13860,#13861,#13862));
#2617=EDGE_LOOP('',(#13863,#13864,#13865,#13866));
#2618=EDGE_LOOP('',(#13867,#13868,#13869,#13870));
#2619=EDGE_LOOP('',(#13871,#13872,#13873,#13874));
#2620=EDGE_LOOP('',(#13875,#13876,#13877));
#2621=EDGE_LOOP('',(#13878,#13879,#13880,#13881));
#2622=EDGE_LOOP('',(#13882,#13883,#13884,#13885));
#2623=EDGE_LOOP('',(#13886,#13887,#13888,#13889));
#2624=EDGE_LOOP('',(#13890,#13891,#13892,#13893));
#2625=EDGE_LOOP('',(#13894,#13895,#13896,#13897));
#2626=EDGE_LOOP('',(#13898,#13899,#13900,#13901));
#2627=EDGE_LOOP('',(#13902,#13903,#13904,#13905));
#2628=EDGE_LOOP('',(#13906,#13907,#13908,#13909));
#2629=EDGE_LOOP('',(#13910,#13911,#13912));
#2630=EDGE_LOOP('',(#13913,#13914,#13915,#13916));
#2631=EDGE_LOOP('',(#13917,#13918,#13919,#13920));
#2632=EDGE_LOOP('',(#13921,#13922,#13923,#13924));
#2633=EDGE_LOOP('',(#13925,#13926,#13927,#13928,#13929,#13930));
#2634=EDGE_LOOP('',(#13931,#13932,#13933,#13934));
#2635=EDGE_LOOP('',(#13935,#13936,#13937,#13938,#13939,#13940));
#2636=EDGE_LOOP('',(#13941,#13942,#13943,#13944));
#2637=EDGE_LOOP('',(#13945,#13946,#13947,#13948));
#2638=EDGE_LOOP('',(#13949,#13950,#13951,#13952));
#2639=EDGE_LOOP('',(#13953,#13954,#13955,#13956,#13957,#13958));
#2640=EDGE_LOOP('',(#13959,#13960,#13961,#13962));
#2641=EDGE_LOOP('',(#13963,#13964,#13965,#13966));
#2642=EDGE_LOOP('',(#13967,#13968,#13969,#13970,#13971));
#2643=EDGE_LOOP('',(#13972,#13973,#13974,#13975));
#2644=EDGE_LOOP('',(#13976,#13977,#13978,#13979));
#2645=EDGE_LOOP('',(#13980,#13981,#13982,#13983,#13984));
#2646=EDGE_LOOP('',(#13985,#13986,#13987));
#2647=EDGE_LOOP('',(#13988,#13989,#13990,#13991));
#2648=EDGE_LOOP('',(#13992,#13993,#13994,#13995));
#2649=EDGE_LOOP('',(#13996,#13997,#13998,#13999));
#2650=EDGE_LOOP('',(#14000,#14001,#14002));
#2651=EDGE_LOOP('',(#14003,#14004,#14005,#14006));
#2652=EDGE_LOOP('',(#14007,#14008,#14009,#14010,#14011,#14012));
#2653=EDGE_LOOP('',(#14013,#14014,#14015,#14016,#14017,#14018));
#2654=EDGE_LOOP('',(#14019,#14020,#14021,#14022,#14023));
#2655=EDGE_LOOP('',(#14024,#14025,#14026));
#2656=EDGE_LOOP('',(#14027,#14028,#14029,#14030));
#2657=EDGE_LOOP('',(#14031,#14032,#14033,#14034,#14035,#14036));
#2658=EDGE_LOOP('',(#14037,#14038,#14039,#14040));
#2659=EDGE_LOOP('',(#14041,#14042,#14043,#14044));
#2660=EDGE_LOOP('',(#14045,#14046,#14047,#14048));
#2661=EDGE_LOOP('',(#14049,#14050,#14051,#14052,#14053));
#2662=EDGE_LOOP('',(#14054,#14055,#14056,#14057));
#2663=EDGE_LOOP('',(#14058,#14059,#14060,#14061));
#2664=EDGE_LOOP('',(#14062,#14063,#14064,#14065));
#2665=EDGE_LOOP('',(#14066,#14067,#14068,#14069));
#2666=EDGE_LOOP('',(#14070,#14071,#14072,#14073));
#2667=EDGE_LOOP('',(#14074,#14075,#14076,#14077));
#2668=EDGE_LOOP('',(#14078,#14079,#14080,#14081));
#2669=EDGE_LOOP('',(#14082,#14083,#14084,#14085));
#2670=EDGE_LOOP('',(#14086,#14087,#14088,#14089));
#2671=EDGE_LOOP('',(#14090,#14091,#14092));
#2672=EDGE_LOOP('',(#14093,#14094,#14095,#14096));
#2673=EDGE_LOOP('',(#14097,#14098,#14099));
#2674=EDGE_LOOP('',(#14100,#14101,#14102,#14103));
#2675=EDGE_LOOP('',(#14104,#14105,#14106,#14107));
#2676=EDGE_LOOP('',(#14108,#14109,#14110,#14111));
#2677=EDGE_LOOP('',(#14112,#14113,#14114,#14115));
#2678=EDGE_LOOP('',(#14116,#14117,#14118,#14119));
#2679=EDGE_LOOP('',(#14120,#14121,#14122,#14123));
#2680=EDGE_LOOP('',(#14124,#14125,#14126,#14127));
#2681=EDGE_LOOP('',(#14128,#14129,#14130,#14131));
#2682=EDGE_LOOP('',(#14132,#14133,#14134,#14135,#14136));
#2683=EDGE_LOOP('',(#14137,#14138,#14139));
#2684=EDGE_LOOP('',(#14140,#14141,#14142,#14143));
#2685=EDGE_LOOP('',(#14144,#14145,#14146,#14147));
#2686=EDGE_LOOP('',(#14148,#14149,#14150,#14151,#14152,#14153));
#2687=EDGE_LOOP('',(#14154,#14155,#14156));
#2688=EDGE_LOOP('',(#14157,#14158,#14159,#14160,#14161,#14162));
#2689=EDGE_LOOP('',(#14163,#14164,#14165,#14166,#14167));
#2690=EDGE_LOOP('',(#14168,#14169,#14170,#14171));
#2691=EDGE_LOOP('',(#14172,#14173,#14174,#14175));
#2692=EDGE_LOOP('',(#14176,#14177,#14178,#14179));
#2693=EDGE_LOOP('',(#14180,#14181,#14182));
#2694=EDGE_LOOP('',(#14183,#14184,#14185,#14186));
#2695=EDGE_LOOP('',(#14187,#14188,#14189));
#2696=EDGE_LOOP('',(#14190,#14191,#14192,#14193));
#2697=EDGE_LOOP('',(#14194,#14195,#14196,#14197));
#2698=EDGE_LOOP('',(#14198,#14199,#14200,#14201));
#2699=EDGE_LOOP('',(#14202,#14203,#14204,#14205));
#2700=EDGE_LOOP('',(#14206,#14207,#14208,#14209));
#2701=EDGE_LOOP('',(#14210,#14211,#14212,#14213));
#2702=EDGE_LOOP('',(#14214,#14215,#14216,#14217,#14218,#14219));
#2703=EDGE_LOOP('',(#14220,#14221,#14222,#14223));
#2704=EDGE_LOOP('',(#14224,#14225,#14226,#14227));
#2705=EDGE_LOOP('',(#14228,#14229,#14230,#14231,#14232));
#2706=EDGE_LOOP('',(#14233,#14234,#14235,#14236,#14237));
#2707=EDGE_LOOP('',(#14238,#14239,#14240));
#2708=EDGE_LOOP('',(#14241,#14242,#14243,#14244));
#2709=EDGE_LOOP('',(#14245,#14246,#14247,#14248,#14249));
#2710=EDGE_LOOP('',(#14250,#14251,#14252,#14253));
#2711=EDGE_LOOP('',(#14254,#14255,#14256,#14257,#14258));
#2712=EDGE_LOOP('',(#14259,#14260,#14261,#14262,#14263,#14264));
#2713=EDGE_LOOP('',(#14265,#14266,#14267,#14268));
#2714=EDGE_LOOP('',(#14269,#14270,#14271,#14272));
#2715=EDGE_LOOP('',(#14273,#14274,#14275,#14276));
#2716=EDGE_LOOP('',(#14277,#14278,#14279,#14280));
#2717=EDGE_LOOP('',(#14281,#14282,#14283,#14284));
#2718=EDGE_LOOP('',(#14285,#14286,#14287,#14288));
#2719=EDGE_LOOP('',(#14289,#14290,#14291,#14292));
#2720=EDGE_LOOP('',(#14293,#14294,#14295,#14296));
#2721=EDGE_LOOP('',(#14297,#14298,#14299,#14300));
#2722=EDGE_LOOP('',(#14301,#14302,#14303));
#2723=EDGE_LOOP('',(#14304,#14305,#14306));
#2724=EDGE_LOOP('',(#14307,#14308,#14309,#14310,#14311));
#2725=EDGE_LOOP('',(#14312,#14313,#14314,#14315));
#2726=EDGE_LOOP('',(#14316,#14317,#14318,#14319));
#2727=EDGE_LOOP('',(#14320,#14321,#14322,#14323));
#2728=EDGE_LOOP('',(#14324,#14325,#14326,#14327));
#2729=EDGE_LOOP('',(#14328,#14329,#14330));
#2730=EDGE_LOOP('',(#14331,#14332,#14333,#14334,#14335));
#2731=EDGE_LOOP('',(#14336,#14337,#14338,#14339));
#2732=EDGE_LOOP('',(#14340,#14341,#14342,#14343));
#2733=EDGE_LOOP('',(#14344,#14345,#14346,#14347));
#2734=EDGE_LOOP('',(#14348,#14349,#14350,#14351,#14352));
#2735=EDGE_LOOP('',(#14353,#14354,#14355));
#2736=EDGE_LOOP('',(#14356,#14357,#14358,#14359));
#2737=EDGE_LOOP('',(#14360,#14361,#14362,#14363,#14364,#14365));
#2738=EDGE_LOOP('',(#14366,#14367,#14368,#14369,#14370,#14371));
#2739=EDGE_LOOP('',(#14372,#14373,#14374,#14375,#14376));
#2740=EDGE_LOOP('',(#14377,#14378,#14379,#14380));
#2741=EDGE_LOOP('',(#14381,#14382,#14383,#14384,#14385,#14386));
#2742=EDGE_LOOP('',(#14387,#14388,#14389,#14390,#14391,#14392));
#2743=EDGE_LOOP('',(#14393,#14394,#14395));
#2744=EDGE_LOOP('',(#14396,#14397,#14398,#14399,#14400,#14401));
#2745=EDGE_LOOP('',(#14402,#14403,#14404));
#2746=EDGE_LOOP('',(#14405,#14406,#14407,#14408,#14409));
#2747=EDGE_LOOP('',(#14410,#14411,#14412,#14413));
#2748=EDGE_LOOP('',(#14414,#14415,#14416,#14417));
#2749=EDGE_LOOP('',(#14418,#14419,#14420,#14421));
#2750=EDGE_LOOP('',(#14422,#14423,#14424,#14425,#14426,#14427));
#2751=EDGE_LOOP('',(#14428,#14429,#14430,#14431));
#2752=EDGE_LOOP('',(#14432,#14433,#14434));
#2753=EDGE_LOOP('',(#14435,#14436,#14437,#14438));
#2754=EDGE_LOOP('',(#14439,#14440,#14441,#14442,#14443));
#2755=EDGE_LOOP('',(#14444,#14445,#14446,#14447,#14448,#14449,#14450,#14451,
#14452,#14453,#14454,#14455,#14456,#14457,#14458,#14459,#14460,#14461,#14462,
#14463,#14464));
#2756=EDGE_LOOP('',(#14465));
#2757=EDGE_LOOP('',(#14466));
#2758=EDGE_LOOP('',(#14467,#14468,#14469,#14470,#14471));
#2759=EDGE_LOOP('',(#14472,#14473,#14474,#14475));
#2760=EDGE_LOOP('',(#14476,#14477,#14478,#14479));
#2761=EDGE_LOOP('',(#14480,#14481,#14482));
#2762=EDGE_LOOP('',(#14483,#14484,#14485,#14486,#14487,#14488));
#2763=EDGE_LOOP('',(#14489,#14490,#14491,#14492));
#2764=EDGE_LOOP('',(#14493,#14494,#14495,#14496,#14497,#14498,#14499,#14500,
#14501,#14502,#14503,#14504,#14505,#14506,#14507,#14508));
#2765=EDGE_LOOP('',(#14509));
#2766=EDGE_LOOP('',(#14510,#14511,#14512,#14513));
#2767=EDGE_LOOP('',(#14514,#14515,#14516,#14517));
#2768=EDGE_LOOP('',(#14518,#14519,#14520,#14521));
#2769=EDGE_LOOP('',(#14522,#14523,#14524,#14525,#14526,#14527));
#2770=EDGE_LOOP('',(#14528,#14529,#14530,#14531,#14532));
#2771=EDGE_LOOP('',(#14533,#14534,#14535,#14536));
#2772=EDGE_LOOP('',(#14537,#14538,#14539,#14540,#14541));
#2773=EDGE_LOOP('',(#14542,#14543,#14544,#14545));
#2774=EDGE_LOOP('',(#14546,#14547,#14548,#14549,#14550));
#2775=EDGE_LOOP('',(#14551,#14552,#14553,#14554,#14555,#14556,#14557));
#2776=EDGE_LOOP('',(#14558,#14559,#14560,#14561,#14562));
#2777=EDGE_LOOP('',(#14563,#14564,#14565,#14566,#14567,#14568,#14569,#14570));
#2778=EDGE_LOOP('',(#14571,#14572,#14573,#14574));
#2779=EDGE_LOOP('',(#14575,#14576,#14577));
#2780=EDGE_LOOP('',(#14578,#14579,#14580,#14581,#14582,#14583));
#2781=EDGE_LOOP('',(#14584,#14585,#14586,#14587,#14588,#14589));
#2782=EDGE_LOOP('',(#14590,#14591,#14592,#14593,#14594,#14595,#14596));
#2783=EDGE_LOOP('',(#14597,#14598,#14599,#14600,#14601));
#2784=EDGE_LOOP('',(#14602,#14603,#14604,#14605,#14606,#14607));
#2785=EDGE_LOOP('',(#14608,#14609,#14610,#14611));
#2786=EDGE_LOOP('',(#14612,#14613,#14614,#14615));
#2787=EDGE_LOOP('',(#14616,#14617,#14618,#14619,#14620));
#2788=EDGE_LOOP('',(#14621,#14622,#14623,#14624));
#2789=EDGE_LOOP('',(#14625,#14626,#14627,#14628,#14629));
#2790=EDGE_LOOP('',(#14630,#14631,#14632,#14633));
#2791=EDGE_LOOP('',(#14634,#14635,#14636));
#2792=EDGE_LOOP('',(#14637,#14638,#14639));
#2793=EDGE_LOOP('',(#14640,#14641,#14642,#14643));
#2794=EDGE_LOOP('',(#14644,#14645,#14646,#14647,#14648,#14649));
#2795=EDGE_LOOP('',(#14650,#14651,#14652,#14653));
#2796=EDGE_LOOP('',(#14654,#14655,#14656,#14657));
#2797=EDGE_LOOP('',(#14658,#14659,#14660,#14661));
#2798=EDGE_LOOP('',(#14662,#14663,#14664));
#2799=EDGE_LOOP('',(#14665,#14666,#14667));
#2800=EDGE_LOOP('',(#14668,#14669,#14670,#14671));
#2801=EDGE_LOOP('',(#14672,#14673,#14674,#14675));
#2802=EDGE_LOOP('',(#14676,#14677,#14678,#14679,#14680));
#2803=EDGE_LOOP('',(#14681,#14682,#14683,#14684,#14685));
#2804=EDGE_LOOP('',(#14686));
#2805=EDGE_LOOP('',(#14687,#14688,#14689));
#2806=EDGE_LOOP('',(#14690,#14691,#14692,#14693));
#2807=EDGE_LOOP('',(#14694,#14695,#14696,#14697,#14698));
#2808=EDGE_LOOP('',(#14699,#14700,#14701,#14702));
#2809=EDGE_LOOP('',(#14703,#14704,#14705,#14706));
#2810=EDGE_LOOP('',(#14707,#14708,#14709,#14710));
#2811=EDGE_LOOP('',(#14711,#14712,#14713,#14714));
#2812=EDGE_LOOP('',(#14715,#14716,#14717));
#2813=EDGE_LOOP('',(#14718,#14719,#14720,#14721,#14722,#14723));
#2814=EDGE_LOOP('',(#14724,#14725,#14726,#14727,#14728));
#2815=EDGE_LOOP('',(#14729,#14730,#14731,#14732));
#2816=EDGE_LOOP('',(#14733,#14734,#14735,#14736));
#2817=EDGE_LOOP('',(#14737,#14738,#14739,#14740));
#2818=EDGE_LOOP('',(#14741,#14742,#14743,#14744));
#2819=EDGE_LOOP('',(#14745,#14746,#14747,#14748,#14749));
#2820=EDGE_LOOP('',(#14750,#14751,#14752));
#2821=EDGE_LOOP('',(#14753,#14754,#14755,#14756));
#2822=EDGE_LOOP('',(#14757,#14758,#14759,#14760,#14761,#14762));
#2823=EDGE_LOOP('',(#14763,#14764,#14765,#14766));
#2824=EDGE_LOOP('',(#14767,#14768,#14769,#14770,#14771,#14772));
#2825=EDGE_LOOP('',(#14773,#14774,#14775,#14776,#14777));
#2826=EDGE_LOOP('',(#14778,#14779,#14780,#14781));
#2827=EDGE_LOOP('',(#14782,#14783,#14784,#14785,#14786));
#2828=EDGE_LOOP('',(#14787,#14788,#14789,#14790));
#2829=EDGE_LOOP('',(#14791,#14792,#14793,#14794));
#2830=EDGE_LOOP('',(#14795,#14796,#14797,#14798));
#2831=EDGE_LOOP('',(#14799,#14800,#14801,#14802,#14803,#14804));
#2832=EDGE_LOOP('',(#14805,#14806,#14807,#14808,#14809));
#2833=EDGE_LOOP('',(#14810,#14811,#14812,#14813,#14814));
#2834=EDGE_LOOP('',(#14815));
#2835=EDGE_LOOP('',(#14816,#14817,#14818,#14819));
#2836=EDGE_LOOP('',(#14820,#14821,#14822,#14823,#14824));
#2837=EDGE_LOOP('',(#14825,#14826,#14827,#14828));
#2838=EDGE_LOOP('',(#14829,#14830,#14831,#14832));
#2839=EDGE_LOOP('',(#14833,#14834,#14835,#14836));
#2840=EDGE_LOOP('',(#14837,#14838,#14839,#14840));
#2841=EDGE_LOOP('',(#14841,#14842,#14843,#14844));
#2842=EDGE_LOOP('',(#14845,#14846,#14847,#14848));
#2843=EDGE_LOOP('',(#14849,#14850,#14851,#14852));
#2844=EDGE_LOOP('',(#14853,#14854,#14855,#14856));
#2845=EDGE_LOOP('',(#14857,#14858,#14859,#14860,#14861));
#2846=EDGE_LOOP('',(#14862,#14863,#14864,#14865));
#2847=EDGE_LOOP('',(#14866,#14867,#14868));
#2848=EDGE_LOOP('',(#14869,#14870,#14871,#14872));
#2849=EDGE_LOOP('',(#14873,#14874,#14875,#14876,#14877));
#2850=EDGE_LOOP('',(#14878,#14879,#14880,#14881));
#2851=EDGE_LOOP('',(#14882,#14883,#14884,#14885,#14886));
#2852=EDGE_LOOP('',(#14887,#14888,#14889,#14890,#14891,#14892));
#2853=EDGE_LOOP('',(#14893));
#2854=EDGE_LOOP('',(#14894));
#2855=EDGE_LOOP('',(#14895,#14896,#14897,#14898,#14899,#14900));
#2856=EDGE_LOOP('',(#14901,#14902,#14903,#14904,#14905,#14906));
#2857=EDGE_LOOP('',(#14907,#14908,#14909,#14910,#14911));
#2858=EDGE_LOOP('',(#14912,#14913,#14914,#14915,#14916));
#2859=EDGE_LOOP('',(#14917));
#2860=EDGE_LOOP('',(#14918,#14919,#14920,#14921,#14922));
#2861=EDGE_LOOP('',(#14923,#14924,#14925,#14926,#14927));
#2862=EDGE_LOOP('',(#14928));
#2863=EDGE_LOOP('',(#14929,#14930,#14931,#14932,#14933,#14934));
#2864=EDGE_LOOP('',(#14935,#14936,#14937,#14938));
#2865=EDGE_LOOP('',(#14939,#14940,#14941,#14942));
#2866=EDGE_LOOP('',(#14943,#14944,#14945,#14946));
#2867=EDGE_LOOP('',(#14947,#14948,#14949));
#2868=EDGE_LOOP('',(#14950,#14951,#14952,#14953,#14954,#14955));
#2869=EDGE_LOOP('',(#14956,#14957,#14958,#14959));
#2870=EDGE_LOOP('',(#14960,#14961,#14962,#14963));
#2871=EDGE_LOOP('',(#14964,#14965,#14966,#14967,#14968));
#2872=EDGE_LOOP('',(#14969,#14970,#14971,#14972));
#2873=EDGE_LOOP('',(#14973,#14974,#14975,#14976,#14977));
#2874=EDGE_LOOP('',(#14978,#14979,#14980,#14981,#14982));
#2875=EDGE_LOOP('',(#14983));
#2876=EDGE_LOOP('',(#14984));
#2877=EDGE_LOOP('',(#14985));
#2878=EDGE_LOOP('',(#14986));
#2879=EDGE_LOOP('',(#14987));
#2880=EDGE_LOOP('',(#14988));
#2881=EDGE_LOOP('',(#14989));
#2882=EDGE_LOOP('',(#14990));
#2883=EDGE_LOOP('',(#14991));
#2884=EDGE_LOOP('',(#14992));
#2885=EDGE_LOOP('',(#14993));
#2886=EDGE_LOOP('',(#14994));
#2887=EDGE_LOOP('',(#14995,#14996,#14997,#14998,#14999));
#2888=EDGE_LOOP('',(#15000,#15001,#15002,#15003,#15004));
#2889=EDGE_LOOP('',(#15005,#15006,#15007,#15008,#15009));
#2890=EDGE_LOOP('',(#15010,#15011,#15012,#15013,#15014));
#2891=EDGE_LOOP('',(#15015,#15016,#15017,#15018,#15019));
#2892=EDGE_LOOP('',(#15020,#15021,#15022,#15023,#15024));
#2893=EDGE_LOOP('',(#15025,#15026,#15027,#15028,#15029));
#2894=EDGE_LOOP('',(#15030,#15031,#15032,#15033,#15034));
#2895=EDGE_LOOP('',(#15035,#15036,#15037,#15038,#15039));
#2896=EDGE_LOOP('',(#15040,#15041,#15042,#15043,#15044));
#2897=EDGE_LOOP('',(#15045,#15046,#15047,#15048));
#2898=EDGE_LOOP('',(#15049,#15050,#15051,#15052));
#2899=EDGE_LOOP('',(#15053));
#2900=EDGE_LOOP('',(#15054));
#2901=EDGE_LOOP('',(#15055,#15056,#15057,#15058));
#2902=EDGE_LOOP('',(#15059,#15060,#15061,#15062));
#2903=EDGE_LOOP('',(#15063));
#2904=EDGE_LOOP('',(#15064));
#2905=EDGE_LOOP('',(#15065,#15066,#15067,#15068));
#2906=EDGE_LOOP('',(#15069,#15070,#15071,#15072));
#2907=EDGE_LOOP('',(#15073));
#2908=EDGE_LOOP('',(#15074));
#2909=EDGE_LOOP('',(#15075,#15076,#15077,#15078));
#2910=EDGE_LOOP('',(#15079,#15080,#15081,#15082));
#2911=EDGE_LOOP('',(#15083,#15084,#15085));
#2912=EDGE_LOOP('',(#15086,#15087,#15088,#15089,#15090,#15091,#15092,#15093));
#2913=EDGE_LOOP('',(#15094,#15095,#15096,#15097,#15098));
#2914=EDGE_LOOP('',(#15099,#15100,#15101,#15102,#15103,#15104));
#2915=EDGE_LOOP('',(#15105,#15106,#15107,#15108,#15109,#15110));
#2916=EDGE_LOOP('',(#15111,#15112,#15113,#15114,#15115,#15116));
#2917=EDGE_LOOP('',(#15117,#15118,#15119,#15120,#15121));
#2918=EDGE_LOOP('',(#15122));
#2919=EDGE_LOOP('',(#15123));
#2920=EDGE_LOOP('',(#15124));
#2921=EDGE_LOOP('',(#15125));
#2922=EDGE_LOOP('',(#15126));
#2923=EDGE_LOOP('',(#15127));
#2924=EDGE_LOOP('',(#15128));
#2925=EDGE_LOOP('',(#15129));
#2926=EDGE_LOOP('',(#15130,#15131,#15132,#15133));
#2927=EDGE_LOOP('',(#15134,#15135,#15136,#15137));
#2928=EDGE_LOOP('',(#15138,#15139,#15140,#15141));
#2929=EDGE_LOOP('',(#15142,#15143,#15144,#15145,#15146));
#2930=EDGE_LOOP('',(#15147,#15148,#15149,#15150,#15151,#15152));
#2931=EDGE_LOOP('',(#15153,#15154,#15155,#15156,#15157));
#2932=EDGE_LOOP('',(#15158,#15159,#15160,#15161,#15162,#15163));
#2933=EDGE_LOOP('',(#15164,#15165,#15166,#15167,#15168,#15169));
#2934=EDGE_LOOP('',(#15170,#15171,#15172,#15173,#15174));
#2935=EDGE_LOOP('',(#15175,#15176,#15177,#15178,#15179,#15180));
#2936=EDGE_LOOP('',(#15181,#15182,#15183,#15184,#15185,#15186));
#2937=EDGE_LOOP('',(#15187,#15188,#15189,#15190,#15191,#15192,#15193,#15194,
#15195));
#2938=EDGE_LOOP('',(#15196,#15197,#15198,#15199,#15200,#15201,#15202,#15203,
#15204,#15205,#15206,#15207,#15208,#15209,#15210,#15211,#15212,#15213,#15214,
#15215,#15216,#15217,#15218));
#2939=EDGE_LOOP('',(#15219,#15220,#15221,#15222,#15223));
#2940=EDGE_LOOP('',(#15224,#15225,#15226,#15227,#15228,#15229,#15230,#15231,
#15232,#15233,#15234,#15235,#15236,#15237,#15238,#15239,#15240,#15241,#15242,
#15243,#15244,#15245,#15246,#15247,#15248,#15249,#15250,#15251,#15252,#15253,
#15254,#15255,#15256,#15257));
#2941=EDGE_LOOP('',(#15258));
#2942=EDGE_LOOP('',(#15259));
#2943=EDGE_LOOP('',(#15260));
#2944=EDGE_LOOP('',(#15261));
#2945=EDGE_LOOP('',(#15262,#15263,#15264,#15265,#15266));
#2946=EDGE_LOOP('',(#15267,#15268,#15269,#15270,#15271));
#2947=EDGE_LOOP('',(#15272,#15273,#15274,#15275,#15276));
#2948=EDGE_LOOP('',(#15277,#15278,#15279,#15280,#15281));
#2949=EDGE_LOOP('',(#15282,#15283,#15284,#15285,#15286));
#2950=EDGE_LOOP('',(#15287,#15288,#15289,#15290,#15291,#15292));
#2951=EDGE_LOOP('',(#15293,#15294,#15295,#15296,#15297,#15298));
#2952=EDGE_LOOP('',(#15299,#15300,#15301,#15302,#15303));
#2953=EDGE_LOOP('',(#15304,#15305,#15306,#15307,#15308));
#2954=EDGE_LOOP('',(#15309,#15310,#15311,#15312));
#2955=EDGE_LOOP('',(#15313,#15314,#15315,#15316));
#2956=EDGE_LOOP('',(#15317,#15318,#15319,#15320));
#2957=EDGE_LOOP('',(#15321));
#2958=EDGE_LOOP('',(#15322));
#2959=EDGE_LOOP('',(#15323));
#2960=EDGE_LOOP('',(#15324,#15325,#15326,#15327,#15328,#15329,#15330,#15331));
#2961=EDGE_LOOP('',(#15332,#15333));
#2962=EDGE_LOOP('',(#15334,#15335));
#2963=EDGE_LOOP('',(#15336,#15337));
#2964=EDGE_LOOP('',(#15338,#15339,#15340,#15341));
#2965=EDGE_LOOP('',(#15342,#15343));
#2966=EDGE_LOOP('',(#15344,#15345,#15346,#15347));
#2967=EDGE_LOOP('',(#15348,#15349,#15350,#15351));
#2968=EDGE_LOOP('',(#15352,#15353,#15354,#15355));
#2969=EDGE_LOOP('',(#15356,#15357,#15358,#15359));
#2970=EDGE_LOOP('',(#15360,#15361,#15362,#15363));
#3689=CIRCLE('',#20557,0.499999999999999);
#3690=CIRCLE('',#20558,0.500000000000002);
#3691=CIRCLE('',#20560,0.499999999999999);
#3692=CIRCLE('',#20561,0.499999999999998);
#3693=CIRCLE('',#20562,0.499999999999997);
#3694=CIRCLE('',#20564,0.499999999999999);
#3695=CIRCLE('',#20565,0.499999999999998);
#3696=CIRCLE('',#20567,0.499999999999997);
#3697=CIRCLE('',#20568,0.5);
#3698=CIRCLE('',#20570,0.500000000000001);
#3699=CIRCLE('',#20572,0.500000000000001);
#3700=CIRCLE('',#20573,0.499999999999999);
#3701=CIRCLE('',#20574,0.499999999999999);
#3702=CIRCLE('',#20575,0.5);
#3703=CIRCLE('',#20577,0.499999999999998);
#3704=CIRCLE('',#20579,0.499999999999999);
#3705=CIRCLE('',#20580,0.499999999999999);
#3706=CIRCLE('',#20582,0.499999999999999);
#3707=CIRCLE('',#20584,0.499999999999998);
#3708=CIRCLE('',#20587,0.5);
#3709=CIRCLE('',#20590,0.499999999999999);
#3710=CIRCLE('',#20594,0.499999999999999);
#3711=CIRCLE('',#20596,0.5);
#3712=CIRCLE('',#20599,0.5);
#3713=CIRCLE('',#20604,0.499999999999999);
#3714=CIRCLE('',#20606,0.500000000000001);
#3715=CIRCLE('',#20608,0.5);
#3716=CIRCLE('',#20609,0.5);
#3717=CIRCLE('',#20611,0.499999999999999);
#3718=CIRCLE('',#20613,0.5);
#3719=CIRCLE('',#20615,0.5);
#3720=CIRCLE('',#20618,0.500000000000001);
#3721=CIRCLE('',#20619,0.499999999999998);
#3722=CIRCLE('',#20620,0.499999999999999);
#3723=CIRCLE('',#20621,0.499999999999998);
#3724=CIRCLE('',#20624,0.5);
#3725=CIRCLE('',#20626,0.499999999999999);
#3726=CIRCLE('',#20628,0.499999999999997);
#3727=CIRCLE('',#20630,0.499999999999999);
#3728=CIRCLE('',#20632,0.499999999999998);
#3729=CIRCLE('',#20635,0.500000000000001);
#3730=CIRCLE('',#20639,0.5);
#3731=CIRCLE('',#20645,0.500000000000002);
#3732=CIRCLE('',#20647,0.500000000000002);
#3733=CIRCLE('',#20649,0.499999999999999);
#3734=CIRCLE('',#20653,0.499999999999996);
#3735=CIRCLE('',#20655,0.499999999999998);
#3736=CIRCLE('',#20657,0.5);
#3737=CIRCLE('',#20660,0.499999999999999);
#3738=CIRCLE('',#20661,0.5);
#3739=CIRCLE('',#20663,0.499999999999995);
#3740=CIRCLE('',#20664,0.499999999999999);
#3741=CIRCLE('',#20666,0.500000000000001);
#3742=CIRCLE('',#20667,0.499999999999998);
#3743=CIRCLE('',#20668,0.499999999999998);
#3744=CIRCLE('',#20672,0.499999999999999);
#3745=CIRCLE('',#20673,0.499999999999998);
#3746=CIRCLE('',#20675,0.500000000000001);
#3747=CIRCLE('',#20677,0.499999999999999);
#3748=CIRCLE('',#20678,0.5);
#3749=CIRCLE('',#20680,0.499999999999999);
#3750=CIRCLE('',#20682,0.499999999999999);
#3751=CIRCLE('',#20684,0.500000000000001);
#3752=CIRCLE('',#20686,0.499999999999998);
#3753=CIRCLE('',#20689,0.499999999999999);
#3754=CIRCLE('',#20692,0.5);
#3755=CIRCLE('',#20695,0.500000000000005);
#3756=CIRCLE('',#20697,0.499999999999999);
#3757=CIRCLE('',#20700,0.499999999999993);
#3758=CIRCLE('',#20701,0.5);
#3759=CIRCLE('',#20703,0.499999999999999);
#3760=CIRCLE('',#20706,0.499999999999999);
#3761=CIRCLE('',#20709,0.499999999999998);
#3762=CIRCLE('',#20710,0.499999999999999);
#3763=CIRCLE('',#20713,0.5);
#3764=CIRCLE('',#20717,0.499999999999998);
#3765=CIRCLE('',#20718,0.499999999999998);
#3766=CIRCLE('',#20720,0.499999999999997);
#3767=CIRCLE('',#20721,0.5);
#3768=CIRCLE('',#20723,0.499999999999998);
#3769=CIRCLE('',#20725,0.5);
#3770=CIRCLE('',#20731,0.499999999999993);
#3771=CIRCLE('',#20733,0.499999999999999);
#3772=CIRCLE('',#20735,0.499999999999999);
#3773=CIRCLE('',#20738,0.5);
#3774=CIRCLE('',#20740,0.5);
#3775=CIRCLE('',#20742,0.499999999999999);
#3776=CIRCLE('',#20743,0.5);
#3777=CIRCLE('',#20746,0.499999999999995);
#3778=CIRCLE('',#20749,0.5);
#3779=CIRCLE('',#20757,0.499999999999999);
#3780=CIRCLE('',#20760,0.5);
#3781=CIRCLE('',#20762,0.499999999999999);
#3782=CIRCLE('',#20763,0.499999999999999);
#3783=CIRCLE('',#20765,0.500000000000001);
#3784=CIRCLE('',#20766,0.5);
#3785=CIRCLE('',#20767,0.5);
#3786=CIRCLE('',#20769,0.500000000000001);
#3787=CIRCLE('',#20770,0.5);
#3788=CIRCLE('',#20771,0.499999999999999);
#3789=CIRCLE('',#20773,0.5);
#3790=CIRCLE('',#20775,0.500000000000001);
#3791=CIRCLE('',#20777,0.499999999999998);
#3792=CIRCLE('',#20780,0.500000000000005);
#3793=CIRCLE('',#20782,0.499999999999999);
#3794=CIRCLE('',#20783,0.5);
#3795=CIRCLE('',#20785,0.499999999999999);
#3796=CIRCLE('',#20786,0.500000000000001);
#3797=CIRCLE('',#20788,0.5);
#3798=CIRCLE('',#20793,0.5);
#3799=CIRCLE('',#20796,0.499999999999998);
#3800=CIRCLE('',#20800,0.499999999999997);
#3801=CIRCLE('',#20804,0.5);
#3802=CIRCLE('',#20807,0.499999999999999);
#3803=CIRCLE('',#20810,0.499999999999996);
#3804=CIRCLE('',#20812,0.499999999999996);
#3805=CIRCLE('',#20814,0.5);
#3806=CIRCLE('',#20823,0.499999999999999);
#3807=CIRCLE('',#20825,0.499999999999998);
#3808=CIRCLE('',#20828,0.5);
#3809=CIRCLE('',#20830,0.5);
#3810=CIRCLE('',#20834,0.499999999999998);
#3811=CIRCLE('',#20835,0.499999999999998);
#3812=CIRCLE('',#20837,0.499999999999999);
#3813=CIRCLE('',#20840,0.5);
#3814=CIRCLE('',#20844,44.);
#3815=CIRCLE('',#20845,0.5);
#3816=CIRCLE('',#20846,43.5);
#3817=CIRCLE('',#20847,44.);
#3818=CIRCLE('',#20849,44.);
#3819=CIRCLE('',#20850,44.);
#3820=CIRCLE('',#20851,44.);
#3821=CIRCLE('',#20852,44.);
#3822=CIRCLE('',#20853,44.);
#3823=CIRCLE('',#20854,44.);
#3824=CIRCLE('',#20855,44.);
#3825=CIRCLE('',#20856,44.);
#3826=CIRCLE('',#20857,44.);
#3827=CIRCLE('',#20859,42.4);
#3828=CIRCLE('',#20861,0.499999999999997);
#3829=CIRCLE('',#20863,0.499999999999997);
#3830=CIRCLE('',#20864,3.5);
#3831=CIRCLE('',#20865,3.);
#3832=CIRCLE('',#20867,0.500000000000001);
#3833=CIRCLE('',#20869,0.499999999999997);
#3834=CIRCLE('',#20870,0.5);
#3835=CIRCLE('',#20872,0.499999999999997);
#3836=CIRCLE('',#20873,0.5);
#3837=CIRCLE('',#20874,0.500000000000001);
#3838=CIRCLE('',#20875,0.5);
#3839=CIRCLE('',#20876,0.5);
#3840=CIRCLE('',#20878,42.9928932188135);
#3841=CIRCLE('',#20879,3.5);
#3842=CIRCLE('',#20880,42.9928932188135);
#3843=CIRCLE('',#20881,3.5);
#3844=CIRCLE('',#20882,42.9928932188135);
#3845=CIRCLE('',#20883,3.5);
#3846=CIRCLE('',#20884,42.9928932188135);
#3847=CIRCLE('',#20885,7.75710678118654);
#3848=CIRCLE('',#20887,43.3464466094067);
#3849=CIRCLE('',#20888,0.500000000000002);
#3850=CIRCLE('',#20890,43.8535533905933);
#3851=CIRCLE('',#20892,0.499999999999987);
#3852=CIRCLE('',#20894,0.5);
#3853=CIRCLE('',#20896,0.499999999999997);
#3854=CIRCLE('',#20898,0.499999999999995);
#3855=CIRCLE('',#20899,3.);
#3856=CIRCLE('',#20903,0.500000000000007);
#3857=CIRCLE('',#20904,43.3464466094067);
#3858=CIRCLE('',#20906,43.3464466094068);
#3859=CIRCLE('',#20909,43.8535533905933);
#3860=CIRCLE('',#20911,0.5);
#3861=CIRCLE('',#20912,0.500000000000001);
#3862=CIRCLE('',#20913,0.500000000000001);
#3863=CIRCLE('',#20915,0.5);
#3864=CIRCLE('',#20917,0.500000000000001);
#3865=CIRCLE('',#20918,0.500000000000001);
#3866=CIRCLE('',#20919,0.5);
#3867=CIRCLE('',#20921,0.5);
#3868=CIRCLE('',#20922,0.500000000000002);
#3869=CIRCLE('',#20925,43.8535533905933);
#3870=CIRCLE('',#20932,0.499999999999999);
#3871=CIRCLE('',#20933,0.499999999999997);
#3872=CIRCLE('',#20935,0.499999999999997);
#3873=CIRCLE('',#20937,0.499999999999999);
#3874=CIRCLE('',#20939,0.499999999999997);
#3875=CIRCLE('',#20943,0.499999999999991);
#3876=CIRCLE('',#20944,0.499999999999999);
#3877=CIRCLE('',#20945,0.500000000000004);
#3878=CIRCLE('',#20947,0.499999999999995);
#3879=CIRCLE('',#20948,0.5);
#3880=CIRCLE('',#20950,0.5);
#3881=CIRCLE('',#20952,43.8535533905933);
#3882=CIRCLE('',#20953,0.5);
#3883=CIRCLE('',#20955,43.3464466094067);
#3884=CIRCLE('',#20957,43.5);
#3885=CIRCLE('',#20959,3.);
#3886=CIRCLE('',#20960,1.75);
#3887=CIRCLE('',#20962,0.500000000000003);
#3888=CIRCLE('',#20963,0.500000000000004);
#3889=CIRCLE('',#20964,0.499999999999997);
#3890=CIRCLE('',#20966,0.5);
#3891=CIRCLE('',#20968,0.500000000000007);
#3892=CIRCLE('',#20970,0.499999999999997);
#3893=CIRCLE('',#20972,0.499999999999997);
#3894=CIRCLE('',#20973,3.);
#3895=CIRCLE('',#20976,0.499999999999995);
#3896=CIRCLE('',#20980,0.500000000000001);
#3897=CIRCLE('',#20982,3.);
#3898=CIRCLE('',#20984,3.);
#3899=CIRCLE('',#20986,0.5);
#3900=CIRCLE('',#20987,1.25);
#3901=CIRCLE('',#20989,1.25);
#3902=CIRCLE('',#20990,1.25);
#3903=CIRCLE('',#20992,0.499999999999996);
#3904=CIRCLE('',#20993,0.499999999999999);
#3905=CIRCLE('',#20994,0.499999999999998);
#3906=CIRCLE('',#20999,0.5);
#3907=CIRCLE('',#21006,0.499999999999999);
#3908=CIRCLE('',#21011,0.499999999999998);
#3909=CIRCLE('',#21013,0.499999999999997);
#3910=CIRCLE('',#21014,0.499999999999999);
#3911=CIRCLE('',#21021,43.5);
#3912=CIRCLE('',#21023,3.);
#3913=CIRCLE('',#21024,1.75);
#3914=CIRCLE('',#21026,0.5);
#3915=CIRCLE('',#21027,1.25);
#3916=CIRCLE('',#21029,1.25);
#3917=CIRCLE('',#21030,1.25);
#3918=CIRCLE('',#21032,0.499999999999997);
#3919=CIRCLE('',#21033,0.5);
#3920=CIRCLE('',#21035,0.5);
#3921=CIRCLE('',#21037,0.499999999999996);
#3922=CIRCLE('',#21039,0.500000000000003);
#3923=CIRCLE('',#21041,0.499999999999999);
#3924=CIRCLE('',#21043,0.500000000000003);
#3925=CIRCLE('',#21044,0.499999999999999);
#3926=CIRCLE('',#21045,0.5);
#3927=CIRCLE('',#21047,0.5);
#3928=CIRCLE('',#21050,0.499999999999997);
#3929=CIRCLE('',#21052,0.500000000000002);
#3930=CIRCLE('',#21054,0.500000000000001);
#3931=CIRCLE('',#21060,44.);
#3932=CIRCLE('',#21061,0.5);
#3933=CIRCLE('',#21062,43.5);
#3934=CIRCLE('',#21063,44.);
#3935=CIRCLE('',#21065,44.);
#3936=CIRCLE('',#21066,44.);
#3937=CIRCLE('',#21068,42.4);
#3938=CIRCLE('',#21070,43.8535533905933);
#3939=CIRCLE('',#21071,43.8535533905933);
#3940=CIRCLE('',#21072,0.5);
#3941=CIRCLE('',#21074,43.3464466094067);
#3942=CIRCLE('',#21075,43.3464466094067);
#3943=CIRCLE('',#21077,43.5);
#3944=CIRCLE('',#21079,3.);
#3945=CIRCLE('',#21080,1.75);
#3946=CIRCLE('',#21082,43.5);
#3947=CIRCLE('',#21084,1.75);
#3948=CIRCLE('',#21086,0.499999999999999);
#3949=CIRCLE('',#21091,0.499999999999999);
#3950=CIRCLE('',#21093,0.499999999999998);
#3951=CIRCLE('',#21098,0.5);
#3952=CIRCLE('',#21099,1.25);
#3953=CIRCLE('',#21101,1.25);
#3954=CIRCLE('',#21102,1.25);
#3955=CIRCLE('',#21104,0.5);
#3956=CIRCLE('',#21105,1.25);
#3957=CIRCLE('',#21107,1.25);
#3958=CIRCLE('',#21108,1.25);
#3959=CIRCLE('',#21110,3.5);
#3960=CIRCLE('',#21111,0.5);
#3961=CIRCLE('',#21112,3.);
#3962=CIRCLE('',#21113,3.);
#3963=CIRCLE('',#21115,42.9928932188134);
#3964=CIRCLE('',#21116,3.5);
#3965=CIRCLE('',#21117,1.75);
#3966=CIRCLE('',#21118,3.5);
#3967=CIRCLE('',#21119,1.75);
#3968=CIRCLE('',#21120,4.5);
#3969=CIRCLE('',#21121,4.5);
#3970=CIRCLE('',#21122,4.5);
#3971=CIRCLE('',#21123,7.55);
#3972=CIRCLE('',#21124,1.75);
#3973=CIRCLE('',#21125,1.75);
#3974=CIRCLE('',#21127,3.);
#3975=CIRCLE('',#21129,0.5);
#3976=CIRCLE('',#21130,3.);
#3977=CIRCLE('',#21131,3.);
#3978=CIRCLE('',#21133,3.);
#3979=CIRCLE('',#21135,0.5);
#3980=CIRCLE('',#21137,0.5);
#3981=CIRCLE('',#21139,0.5);
#3982=CIRCLE('',#21141,0.5);
#3983=CIRCLE('',#21142,3.);
#3984=CIRCLE('',#21143,3.);
#3985=CIRCLE('',#21145,3.);
#3986=CIRCLE('',#21147,0.5);
#3987=CIRCLE('',#21149,0.5);
#3988=CIRCLE('',#21151,3.);
#3989=CIRCLE('',#21152,0.5);
#3990=CIRCLE('',#21153,3.5);
#3991=CIRCLE('',#21155,3.);
#3992=CIRCLE('',#21157,5.);
#3993=CIRCLE('',#21159,3.);
#3994=CIRCLE('',#21160,0.5);
#3995=CIRCLE('',#21161,3.5);
#3996=CIRCLE('',#21163,3.);
#3997=CIRCLE('',#21165,5.);
#3998=CIRCLE('',#21167,3.);
#3999=CIRCLE('',#21168,0.5);
#4000=CIRCLE('',#21169,3.5);
#4001=CIRCLE('',#21171,3.);
#4002=CIRCLE('',#21173,5.);
#4003=CIRCLE('',#21175,0.499999999999999);
#4004=CIRCLE('',#21177,0.499999999999999);
#4005=CIRCLE('',#21179,0.499999999999998);
#4006=CIRCLE('',#21182,0.5);
#4007=CIRCLE('',#21184,44.);
#4008=CIRCLE('',#21185,44.);
#4009=CIRCLE('',#21186,0.5);
#4010=CIRCLE('',#21187,43.8535533905933);
#4011=CIRCLE('',#21188,43.8535533905933);
#4012=CIRCLE('',#21190,43.5464466094067);
#4013=CIRCLE('',#21191,43.5464466094067);
#4014=CIRCLE('',#21193,44.);
#4015=CIRCLE('',#21194,44.);
#4016=CIRCLE('',#21196,0.5);
#4017=CIRCLE('',#21197,43.1928932188135);
#4018=CIRCLE('',#21199,3.5);
#4019=CIRCLE('',#21200,3.5);
#4020=CIRCLE('',#21201,4.5);
#4021=CIRCLE('',#21202,4.5);
#4022=CIRCLE('',#21203,4.5);
#4023=CIRCLE('',#21204,12.5);
#4024=CIRCLE('',#21205,3.5);
#4025=CIRCLE('',#21207,0.5);
#4026=CIRCLE('',#21209,0.5);
#4027=CIRCLE('',#21211,0.5);
#4028=CIRCLE('',#21213,7.05);
#4029=CIRCLE('',#21214,7.05);
#4030=CIRCLE('',#21215,0.5);
#4031=CIRCLE('',#21217,7.05);
#4032=CIRCLE('',#21218,7.05);
#4033=CIRCLE('',#21220,7.40355339059327);
#4034=CIRCLE('',#21221,0.5);
#4035=CIRCLE('',#21222,7.40355339059327);
#4036=CIRCLE('',#21224,7.19644660940673);
#4037=CIRCLE('',#21225,7.19644660940673);
#4038=CIRCLE('',#21227,0.5);
#4039=CIRCLE('',#21229,0.5);
#4040=CIRCLE('',#21230,12.);
#4041=CIRCLE('',#21231,12.);
#4042=CIRCLE('',#21233,12.);
#4043=CIRCLE('',#21234,12.);
#4044=CIRCLE('',#21236,43.8535533905933);
#4045=CIRCLE('',#21237,43.8535533905933);
#4046=CIRCLE('',#21238,0.5);
#4047=CIRCLE('',#21240,43.5464466094067);
#4048=CIRCLE('',#21241,43.5464466094067);
#4049=CIRCLE('',#21242,43.4);
#4050=CIRCLE('',#21244,43.1928932188135);
#4051=CIRCLE('',#21245,43.1928932188135);
#4052=CIRCLE('',#21246,43.1928932188135);
#4053=CIRCLE('',#21247,43.1928932188135);
#4054=CIRCLE('',#21248,43.1928932188135);
#4055=CIRCLE('',#21249,43.1928932188135);
#4056=CIRCLE('',#21250,43.1928932188135);
#4057=CIRCLE('',#21252,5.5);
#4058=CIRCLE('',#21253,0.5);
#4059=CIRCLE('',#21254,5.);
#4060=CIRCLE('',#21255,5.);
#4061=CIRCLE('',#21257,5.5);
#4062=CIRCLE('',#21258,12.7071067811865);
#4063=CIRCLE('',#21259,5.5);
#4064=CIRCLE('',#21262,0.5);
#4065=CIRCLE('',#21263,5.);
#4066=CIRCLE('',#21264,5.);
#4067=CIRCLE('',#21267,0.5);
#4068=CIRCLE('',#21268,5.);
#4069=CIRCLE('',#21269,5.);
#4070=CIRCLE('',#21272,12.1464466094067);
#4071=CIRCLE('',#21273,0.5);
#4072=CIRCLE('',#21274,12.1464466094067);
#4073=CIRCLE('',#21276,12.3535533905933);
#4074=CIRCLE('',#21277,12.3535533905933);
#4075=CIRCLE('',#21279,0.5);
#5088=B_SPLINE_CURVE_WITH_KNOTS('',3,(#47337,#47338,#47339,#47340,#47341,
#47342),.UNSPECIFIED.,.F.,.F.,(4,2,4),(0.30198667152271,0.315892269007964,
0.319082038667528),.UNSPECIFIED.);
#5089=B_SPLINE_CURVE_WITH_KNOTS('',3,(#47393,#47394,#47395,#47396,#47397,
#47398,#47399,#47400,#47401,#47402,#47403),.UNSPECIFIED.,.F.,.F.,(4,2,2,
3,4),(-0.0419712710900813,-0.0313437335457433,-0.0138874725471006,0.,0.00645492300733996),
 .UNSPECIFIED.);
#5090=B_SPLINE_CURVE_WITH_KNOTS('',3,(#47454,#47455,#47456,#47457,#47458,
#47459),.UNSPECIFIED.,.F.,.F.,(4,2,4),(0.471466566294365,0.474656335953928,
0.488561933439089),.UNSPECIFIED.);
#5091=B_SPLINE_CURVE_WITH_KNOTS('',3,(#47474,#47475,#47476,#47477),
 .UNSPECIFIED.,.F.,.F.,(4,4),(0.964631000010127,1.09925463072705),
 .UNSPECIFIED.);
#5092=B_SPLINE_CURVE_WITH_KNOTS('',3,(#47480,#47481,#47482,#47483),
 .UNSPECIFIED.,.F.,.F.,(4,4),(1.86383746795727,1.99846109867419),
 .UNSPECIFIED.);
#5093=B_SPLINE_CURVE_WITH_KNOTS('',3,(#47493,#47494,#47495,#47496,#47497,
#47498,#47499,#47500,#47501,#47502,#47503),.UNSPECIFIED.,.F.,.F.,(4,3,2,
2,4),(-0.00645830092897804,0.,0.0122190666797987,0.0290968711311065,0.0419019462529983),
 .UNSPECIFIED.);
#5094=B_SPLINE_CURVE_WITH_KNOTS('',3,(#47602,#47603,#47604,#47605,#47606,
#47607,#47608,#47609,#47610,#47611,#47612),.UNSPECIFIED.,.F.,.F.,(4,3,2,
2,4),(-0.00645830092897708,0.,0.012219066679791,0.0290968711310762,0.041901946252941),
 .UNSPECIFIED.);
#5095=B_SPLINE_CURVE_WITH_KNOTS('',3,(#47633,#47634,#47635,#47636),
 .UNSPECIFIED.,.F.,.F.,(4,4),(0.964631000010129,1.09925463072705),
 .UNSPECIFIED.);
#5096=B_SPLINE_CURVE_WITH_KNOTS('',3,(#47640,#47641,#47642,#47643),
 .UNSPECIFIED.,.F.,.F.,(4,4),(1.86383746795727,1.99846109867419),
 .UNSPECIFIED.);
#5097=B_SPLINE_CURVE_WITH_KNOTS('',3,(#47654,#47655,#47656,#47657,#47658,
#47659,#47660,#47661,#47662,#47663,#47664),.UNSPECIFIED.,.F.,.F.,(4,2,2,
3,4),(-0.0419712710901671,-0.031343733545801,-0.0138874725471113,0.,0.00645492300734379),
 .UNSPECIFIED.);
#5098=B_SPLINE_CURVE_WITH_KNOTS('',3,(#47717,#47718,#47719,#47720,#47721,
#47722,#47723,#47724),.UNSPECIFIED.,.F.,.F.,(4,2,2,4),(0.169835657785507,
0.171492731661375,0.184845562376643,0.187089348107769),.UNSPECIFIED.);
#5099=B_SPLINE_CURVE_WITH_KNOTS('',3,(#47913,#47914,#47915,#47916),
 .UNSPECIFIED.,.F.,.F.,(4,4),(0.0456172479668645,0.054374780828201),
 .UNSPECIFIED.);
#5100=B_SPLINE_CURVE_WITH_KNOTS('',3,(#47923,#47924,#47925,#47926,#47927,
#47928,#47929,#47930),.UNSPECIFIED.,.F.,.F.,(4,2,2,4),(0.339943055200166,
0.342186840931291,0.35553967164656,0.357196745522428),.UNSPECIFIED.);
#5101=B_SPLINE_CURVE_WITH_KNOTS('',3,(#47937,#47938,#47939,#47940,#47941,
#47942,#47943,#47944,#47945,#47946,#47947),.UNSPECIFIED.,.F.,.F.,(4,2,2,
3,4),(-0.0419712710900602,-0.0313437335457316,-0.0138874725471015,0.,0.0064549230073403),
 .UNSPECIFIED.);
#5102=B_SPLINE_CURVE_WITH_KNOTS('',3,(#48014,#48015,#48016,#48017,#48018,
#48019,#48020,#48021,#48022,#48023),.UNSPECIFIED.,.F.,.F.,(4,2,2,2,4),(0.23372232720254,
0.240645165240831,0.255490442096141,0.27033571895145,0.287205208370036),
 .UNSPECIFIED.);
#5103=B_SPLINE_CURVE_WITH_KNOTS('',3,(#48030,#48031,#48032,#48033,#48034,
#48035,#48036,#48037,#48038,#48039),.UNSPECIFIED.,.F.,.F.,(4,2,2,2,4),(-0.0417111144051926,
-0.0413742569498193,-0.0219183984840148,-0.00139787181587547,-0.000254064777074337),
 .UNSPECIFIED.);
#5104=B_SPLINE_CURVE_WITH_KNOTS('',3,(#48094,#48095,#48096,#48097),
 .UNSPECIFIED.,.F.,.F.,(4,4),(0.363335998515663,0.499634934734419),
 .UNSPECIFIED.);
#5105=B_SPLINE_CURVE_WITH_KNOTS('',3,(#48098,#48099,#48100,#48101),
 .UNSPECIFIED.,.F.,.F.,(4,4),(-0.499634934734419,-0.363335998515663),
 .UNSPECIFIED.);
#5106=B_SPLINE_CURVE_WITH_KNOTS('',3,(#48137,#48138,#48139,#48140),
 .UNSPECIFIED.,.F.,.F.,(4,4),(-0.0923903836946144,0.),.UNSPECIFIED.);
#5107=B_SPLINE_CURVE_WITH_KNOTS('',3,(#48148,#48149,#48150,#48151,#48152,
#48153,#48154,#48155,#48156,#48157,#48158,#48159,#48160,#48161),
 .UNSPECIFIED.,.F.,.F.,(4,2,2,2,2,2,4),(-0.224987174815843,-0.22451346339712,
-0.196761712223143,-0.16971876072295,-0.144143929728093,-0.124672759657506,
-0.107525143255139),.UNSPECIFIED.);
#5108=B_SPLINE_CURVE_WITH_KNOTS('',3,(#48165,#48166,#48167,#48168,#48169,
#48170,#48171,#48172,#48173,#48174),.UNSPECIFIED.,.F.,.F.,(4,2,2,2,4),(0.233722327202539,
0.24064516524083,0.255490442096139,0.270335718951448,0.287205208370034),
 .UNSPECIFIED.);
#5109=B_SPLINE_CURVE_WITH_KNOTS('',3,(#48178,#48179,#48180,#48181,#48182,
#48183,#48184,#48185,#48186,#48187),.UNSPECIFIED.,.F.,.F.,(4,2,2,2,4),(-0.0417109259698474,
-0.0413740649215941,-0.021971461689753,-0.00144737185821615,-0.000254064846037182),
 .UNSPECIFIED.);
#5110=B_SPLINE_CURVE_WITH_KNOTS('',3,(#48194,#48195,#48196,#48197,#48198,
#48199),.UNSPECIFIED.,.F.,.F.,(4,2,4),(-0.190951927958331,0.,0.00159258460364357),
 .UNSPECIFIED.);
#5111=B_SPLINE_CURVE_WITH_KNOTS('',3,(#48209,#48210,#48211,#48212),
 .UNSPECIFIED.,.F.,.F.,(4,4),(0.112297946941942,0.113633052740004),
 .UNSPECIFIED.);
#5112=B_SPLINE_CURVE_WITH_KNOTS('',3,(#48220,#48221,#48222,#48223),
 .UNSPECIFIED.,.F.,.F.,(4,4),(0.0372440833740091,0.041304702596258),
 .UNSPECIFIED.);
#5113=B_SPLINE_CURVE_WITH_KNOTS('',3,(#48227,#48228,#48229,#48230,#48231,
#48232),.UNSPECIFIED.,.F.,.F.,(4,2,4),(0.0372440833834408,0.0623721844208971,
0.0947431788431503),.UNSPECIFIED.);
#5114=B_SPLINE_CURVE_WITH_KNOTS('',3,(#48238,#48239,#48240,#48241,#48242,
#48243,#48244,#48245,#48246,#48247),.UNSPECIFIED.,.F.,.F.,(4,2,2,2,4),(0.133960440718842,
0.134063881015114,0.159415678018092,0.18476747502107,0.205333050889553),
 .UNSPECIFIED.);
#5115=B_SPLINE_CURVE_WITH_KNOTS('',3,(#48254,#48255,#48256,#48257,#48258,
#48259,#48260,#48261,#48262,#48263,#48264,#48265,#48266,#48267),
 .UNSPECIFIED.,.F.,.F.,(4,2,2,2,2,2,4),(-0.224987174750142,-0.224513463331962,
-0.196761712162241,-0.169718760666431,-0.144143929682433,-0.124672759619459,
-0.107525143228149),.UNSPECIFIED.);
#5116=B_SPLINE_CURVE_WITH_KNOTS('',3,(#48268,#48269,#48270,#48271,#48272,
#48273,#48274,#48275,#48276,#48277),.UNSPECIFIED.,.F.,.F.,(4,2,2,2,4),(-0.0530664398487118,
-0.0526203138668234,-0.0265376315324865,-0.00211254843584519,-0.000314678867370228),
 .UNSPECIFIED.);
#5117=B_SPLINE_CURVE_WITH_KNOTS('',3,(#48309,#48310,#48311,#48312),
 .UNSPECIFIED.,.F.,.F.,(4,4),(-0.136299039595008,0.),.UNSPECIFIED.);
#5118=B_SPLINE_CURVE_WITH_KNOTS('',3,(#48315,#48316,#48317,#48318),
 .UNSPECIFIED.,.F.,.F.,(4,4),(0.,0.136299039595008),.UNSPECIFIED.);
#5119=B_SPLINE_CURVE_WITH_KNOTS('',3,(#48323,#48324,#48325,#48326,#48327,
#48328,#48329,#48330,#48331,#48332,#48333,#48334,#48335,#48336),
 .UNSPECIFIED.,.F.,.F.,(4,2,2,2,2,2,4),(-0.224987174736304,-0.224513463317212,
-0.196761712147415,-0.169718760651608,-0.144143929670733,-0.124672759609814,
-0.107525143222326),.UNSPECIFIED.);
#5120=B_SPLINE_CURVE_WITH_KNOTS('',3,(#48353,#48354,#48355,#48356),
 .UNSPECIFIED.,.F.,.F.,(4,4),(0.0372440833740096,0.0413047025962583),
 .UNSPECIFIED.);
#5121=B_SPLINE_CURVE_WITH_KNOTS('',3,(#48360,#48361,#48362,#48363,#48364,
#48365),.UNSPECIFIED.,.F.,.F.,(4,2,4),(0.0372440833834404,0.0623721844208965,
0.0947431788431497),.UNSPECIFIED.);
#5122=B_SPLINE_CURVE_WITH_KNOTS('',3,(#48372,#48373,#48374,#48375,#48376,
#48377,#48378,#48379),.UNSPECIFIED.,.F.,.F.,(4,2,2,4),(-0.000448465708050994,
0.,0.0249528266048236,0.0484519800048465),.UNSPECIFIED.);
#5123=B_SPLINE_CURVE_WITH_KNOTS('',3,(#48381,#48382,#48383,#48384,#48385,
#48386,#48387,#48388),.UNSPECIFIED.,.F.,.F.,(4,2,2,4),(-0.0487006899272012,
-0.0286121652027313,0.,0.000200219383804073),.UNSPECIFIED.);
#5124=B_SPLINE_CURVE_WITH_KNOTS('',3,(#48394,#48395,#48396,#48397,#48398,
#48399,#48400,#48401),.UNSPECIFIED.,.F.,.F.,(4,2,2,4),(-0.00044846570820805,
0.,0.0249528266047917,0.0484519800048519),.UNSPECIFIED.);
#5125=B_SPLINE_CURVE_WITH_KNOTS('',3,(#48403,#48404,#48405,#48406,#48407,
#48408,#48409,#48410),.UNSPECIFIED.,.F.,.F.,(4,2,2,4),(-0.0487006899269451,
-0.028612165202599,0.,0.000200219383555375),.UNSPECIFIED.);
#5126=B_SPLINE_CURVE_WITH_KNOTS('',3,(#48435,#48436,#48437,#48438),
 .UNSPECIFIED.,.F.,.F.,(4,4),(0.,0.0923903836946144),.UNSPECIFIED.);
#5127=B_SPLINE_CURVE_WITH_KNOTS('',3,(#48451,#48452,#48453,#48454,#48455,
#48456),.UNSPECIFIED.,.F.,.F.,(4,2,4),(0.0372440833834417,0.0623721844208971,
0.0947431788431506),.UNSPECIFIED.);
#5128=B_SPLINE_CURVE_WITH_KNOTS('',3,(#48461,#48462,#48463,#48464,#48465,
#48466,#48467,#48468),.UNSPECIFIED.,.F.,.F.,(4,2,2,4),(-0.0487006899272249,
-0.0286121652027421,0.,0.000200219383468989),.UNSPECIFIED.);
#5129=B_SPLINE_CURVE_WITH_KNOTS('',3,(#48473,#48474,#48475,#48476,#48477,
#48478,#48479,#48480),.UNSPECIFIED.,.F.,.F.,(4,2,2,4),(-0.0487006899264554,
-0.0286121652025119,0.,0.000200219383993128),.UNSPECIFIED.);
#5130=B_SPLINE_CURVE_WITH_KNOTS('',3,(#48502,#48503,#48504,#48505),
 .UNSPECIFIED.,.F.,.F.,(4,4),(-0.0923903843306348,0.),.UNSPECIFIED.);
#5131=B_SPLINE_CURVE_WITH_KNOTS('',3,(#48507,#48508,#48509,#48510),
 .UNSPECIFIED.,.F.,.F.,(4,4),(0.,0.0923903843306348),.UNSPECIFIED.);
#5132=B_SPLINE_CURVE_WITH_KNOTS('',3,(#48523,#48524,#48525,#48526),
 .UNSPECIFIED.,.F.,.F.,(4,4),(-0.136298877173929,0.),.UNSPECIFIED.);
#5133=B_SPLINE_CURVE_WITH_KNOTS('',3,(#48530,#48531,#48532,#48533,#48534,
#48535),.UNSPECIFIED.,.F.,.F.,(4,2,4),(0.0372440833834397,0.0623721844208972,
0.0947431788431508),.UNSPECIFIED.);
#5134=B_SPLINE_CURVE_WITH_KNOTS('',3,(#48578,#48579,#48580,#48581),
 .UNSPECIFIED.,.F.,.F.,(4,4),(0.,0.136298877173929),.UNSPECIFIED.);
#5135=B_SPLINE_CURVE_WITH_KNOTS('',3,(#48584,#48585,#48586,#48587,#48588,
#48589,#48590,#48591,#48592,#48593,#48594,#48595,#48596,#48597),
 .UNSPECIFIED.,.F.,.F.,(4,2,2,2,2,2,4),(-0.224987174812291,-0.224513463393476,
-0.196761712220003,-0.169718760720331,-0.144143929725999,-0.124672759655815,
-0.107525143253847),.UNSPECIFIED.);
#5136=B_SPLINE_CURVE_WITH_KNOTS('',3,(#48717,#48718,#48719,#48720,#48721,
#48722),.UNSPECIFIED.,.F.,.F.,(4,2,4),(0.435389141045337,0.443174934764026,
0.444151928712643),.UNSPECIFIED.);
#5137=B_SPLINE_CURVE_WITH_KNOTS('',3,(#48998,#48999,#49000,#49001),
 .UNSPECIFIED.,.F.,.F.,(4,4),(0.964631000010116,1.09925463072705),
 .UNSPECIFIED.);
#5138=B_SPLINE_CURVE_WITH_KNOTS('',3,(#49005,#49006,#49007,#49008,#49009,
#49010,#49011,#49012),.UNSPECIFIED.,.F.,.F.,(4,2,2,4),(1.86383746795725,
2.02276765578846,2.10223274970406,2.12738029118256),.UNSPECIFIED.);
#5139=B_SPLINE_CURVE_WITH_KNOTS('',3,(#49019,#49020,#49021,#49022,#49023,
#49024,#49025,#49026,#49027,#49028,#49029),.UNSPECIFIED.,.F.,.F.,(4,3,2,
2,4),(-0.00645830092897787,0.,0.0122190666797978,0.0290968711310892,0.0419019462529432),
 .UNSPECIFIED.);
#5140=B_SPLINE_CURVE_WITH_KNOTS('',3,(#49139,#49140,#49141,#49142),
 .UNSPECIFIED.,.F.,.F.,(4,4),(1.86383746795727,1.99846109867419),
 .UNSPECIFIED.);
#5141=B_SPLINE_CURVE_WITH_KNOTS('',3,(#49145,#49146,#49147,#49148,#49149,
#49150,#49151,#49152),.UNSPECIFIED.,.F.,.F.,(4,2,2,4),(0.835711807501242,
0.860859348980241,0.940324442895844,1.09925463072705),.UNSPECIFIED.);
#5644=LINE('',#47245,#6536);
#5645=LINE('',#47248,#6537);
#5646=LINE('',#47259,#6538);
#5647=LINE('',#47262,#6539);
#5648=LINE('',#47268,#6540);
#5649=LINE('',#47270,#6541);
#5650=LINE('',#47286,#6542);
#5651=LINE('',#47287,#6543);
#5652=LINE('',#47292,#6544);
#5653=LINE('',#47294,#6545);
#5654=LINE('',#47299,#6546);
#5655=LINE('',#47302,#6547);
#5656=LINE('',#47304,#6548);
#5657=LINE('',#47307,#6549);
#5658=LINE('',#47311,#6550);
#5659=LINE('',#47312,#6551);
#5660=LINE('',#47315,#6552);
#5661=LINE('',#47318,#6553);
#5662=LINE('',#47320,#6554);
#5663=LINE('',#47321,#6555);
#5664=LINE('',#47324,#6556);
#5665=LINE('',#47329,#6557);
#5666=LINE('',#47333,#6558);
#5667=LINE('',#47348,#6559);
#5668=LINE('',#47350,#6560);
#5669=LINE('',#47355,#6561);
#5670=LINE('',#47359,#6562);
#5671=LINE('',#47363,#6563);
#5672=LINE('',#47369,#6564);
#5673=LINE('',#47372,#6565);
#5674=LINE('',#47375,#6566);
#5675=LINE('',#47377,#6567);
#5676=LINE('',#47378,#6568);
#5677=LINE('',#47388,#6569);
#5678=LINE('',#47391,#6570);
#5679=LINE('',#47407,#6571);
#5680=LINE('',#47410,#6572);
#5681=LINE('',#47413,#6573);
#5682=LINE('',#47416,#6574);
#5683=LINE('',#47420,#6575);
#5684=LINE('',#47421,#6576);
#5685=LINE('',#47426,#6577);
#5686=LINE('',#47427,#6578);
#5687=LINE('',#47430,#6579);
#5688=LINE('',#47433,#6580);
#5689=LINE('',#47437,#6581);
#5690=LINE('',#47440,#6582);
#5691=LINE('',#47443,#6583);
#5692=LINE('',#47445,#6584);
#5693=LINE('',#47447,#6585);
#5694=LINE('',#47448,#6586);
#5695=LINE('',#47463,#6587);
#5696=LINE('',#47469,#6588);
#5697=LINE('',#47472,#6589);
#5698=LINE('',#47479,#6590);
#5699=LINE('',#47487,#6591);
#5700=LINE('',#47510,#6592);
#5701=LINE('',#47513,#6593);
#5702=LINE('',#47518,#6594);
#5703=LINE('',#47521,#6595);
#5704=LINE('',#47530,#6596);
#5705=LINE('',#47532,#6597);
#5706=LINE('',#47533,#6598);
#5707=LINE('',#47536,#6599);
#5708=LINE('',#47538,#6600);
#5709=LINE('',#47539,#6601);
#5710=LINE('',#47545,#6602);
#5711=LINE('',#47552,#6603);
#5712=LINE('',#47558,#6604);
#5713=LINE('',#47564,#6605);
#5714=LINE('',#47568,#6606);
#5715=LINE('',#47569,#6607);
#5716=LINE('',#47572,#6608);
#5717=LINE('',#47576,#6609);
#5718=LINE('',#47577,#6610);
#5719=LINE('',#47580,#6611);
#5720=LINE('',#47584,#6612);
#5721=LINE('',#47585,#6613);
#5722=LINE('',#47588,#6614);
#5723=LINE('',#47595,#6615);
#5724=LINE('',#47598,#6616);
#5725=LINE('',#47614,#6617);
#5726=LINE('',#47617,#6618);
#5727=LINE('',#47623,#6619);
#5728=LINE('',#47625,#6620);
#5729=LINE('',#47626,#6621);
#5730=LINE('',#47629,#6622);
#5731=LINE('',#47638,#6623);
#5732=LINE('',#47644,#6624);
#5733=LINE('',#47650,#6625);
#5734=LINE('',#47651,#6626);
#5735=LINE('',#47667,#6627);
#5736=LINE('',#47670,#6628);
#5737=LINE('',#47677,#6629);
#5738=LINE('',#47682,#6630);
#5739=LINE('',#47688,#6631);
#5740=LINE('',#47691,#6632);
#5741=LINE('',#47693,#6633);
#5742=LINE('',#47694,#6634);
#5743=LINE('',#47699,#6635);
#5744=LINE('',#47704,#6636);
#5745=LINE('',#47708,#6637);
#5746=LINE('',#47709,#6638);
#5747=LINE('',#47726,#6639);
#5748=LINE('',#47730,#6640);
#5749=LINE('',#47737,#6641);
#5750=LINE('',#47740,#6642);
#5751=LINE('',#47746,#6643);
#5752=LINE('',#47748,#6644);
#5753=LINE('',#47749,#6645);
#5754=LINE('',#47752,#6646);
#5755=LINE('',#47758,#6647);
#5756=LINE('',#47759,#6648);
#5757=LINE('',#47764,#6649);
#5758=LINE('',#47770,#6650);
#5759=LINE('',#47773,#6651);
#5760=LINE('',#47779,#6652);
#5761=LINE('',#47782,#6653);
#5762=LINE('',#47797,#6654);
#5763=LINE('',#47800,#6655);
#5764=LINE('',#47803,#6656);
#5765=LINE('',#47806,#6657);
#5766=LINE('',#47809,#6658);
#5767=LINE('',#47812,#6659);
#5768=LINE('',#47815,#6660);
#5769=LINE('',#47816,#6661);
#5770=LINE('',#47819,#6662);
#5771=LINE('',#47826,#6663);
#5772=LINE('',#47828,#6664);
#5773=LINE('',#47839,#6665);
#5774=LINE('',#47841,#6666);
#5775=LINE('',#47845,#6667);
#5776=LINE('',#47849,#6668);
#5777=LINE('',#47850,#6669);
#5778=LINE('',#47853,#6670);
#5779=LINE('',#47857,#6671);
#5780=LINE('',#47858,#6672);
#5781=LINE('',#47864,#6673);
#5782=LINE('',#47865,#6674);
#5783=LINE('',#47869,#6675);
#5784=LINE('',#47872,#6676);
#5785=LINE('',#47874,#6677);
#5786=LINE('',#47879,#6678);
#5787=LINE('',#47881,#6679);
#5788=LINE('',#47886,#6680);
#5789=LINE('',#47891,#6681);
#5790=LINE('',#47893,#6682);
#5791=LINE('',#47894,#6683);
#5792=LINE('',#47901,#6684);
#5793=LINE('',#47904,#6685);
#5794=LINE('',#47906,#6686);
#5795=LINE('',#47908,#6687);
#5796=LINE('',#47909,#6688);
#5797=LINE('',#47922,#6689);
#5798=LINE('',#47935,#6690);
#5799=LINE('',#47955,#6691);
#5800=LINE('',#47961,#6692);
#5801=LINE('',#47974,#6693);
#5802=LINE('',#47978,#6694);
#5803=LINE('',#47982,#6695);
#5804=LINE('',#47986,#6696);
#5805=LINE('',#47990,#6697);
#5806=LINE('',#47994,#6698);
#5807=LINE('',#47998,#6699);
#5808=LINE('',#48002,#6700);
#5809=LINE('',#48006,#6701);
#5810=LINE('',#48025,#6702);
#5811=LINE('',#48029,#6703);
#5812=LINE('',#48050,#6704);
#5813=LINE('',#48051,#6705);
#5814=LINE('',#48106,#6706);
#5815=LINE('',#48110,#6707);
#5816=LINE('',#48114,#6708);
#5817=LINE('',#48118,#6709);
#5818=LINE('',#48122,#6710);
#5819=LINE('',#48126,#6711);
#5820=LINE('',#48145,#6712);
#5821=LINE('',#48176,#6713);
#5822=LINE('',#48201,#6714);
#5823=LINE('',#48225,#6715);
#5824=LINE('',#48234,#6716);
#5825=LINE('',#48235,#6717);
#5826=LINE('',#48251,#6718);
#5827=LINE('',#48341,#6719);
#5828=LINE('',#48358,#6720);
#5829=LINE('',#48367,#6721);
#5830=LINE('',#48368,#6722);
#5831=LINE('',#48391,#6723);
#5832=LINE('',#48392,#6724);
#5833=LINE('',#48413,#6725);
#5834=LINE('',#48414,#6726);
#5835=LINE('',#48445,#6727);
#5836=LINE('',#48449,#6728);
#5837=LINE('',#48458,#6729);
#5838=LINE('',#48459,#6730);
#5839=LINE('',#48481,#6731);
#5840=LINE('',#48538,#6732);
#5841=LINE('',#48541,#6733);
#5842=LINE('',#48599,#6734);
#5843=LINE('',#48605,#6735);
#5844=LINE('',#48612,#6736);
#5845=LINE('',#48616,#6737);
#5846=LINE('',#48619,#6738);
#5847=LINE('',#48621,#6739);
#5848=LINE('',#48622,#6740);
#5849=LINE('',#48635,#6741);
#5850=LINE('',#48650,#6742);
#5851=LINE('',#48651,#6743);
#5852=LINE('',#48654,#6744);
#5853=LINE('',#48656,#6745);
#5854=LINE('',#48658,#6746);
#5855=LINE('',#48660,#6747);
#5856=LINE('',#48661,#6748);
#5857=LINE('',#48664,#6749);
#5858=LINE('',#48671,#6750);
#5859=LINE('',#48677,#6751);
#5860=LINE('',#48681,#6752);
#5861=LINE('',#48685,#6753);
#5862=LINE('',#48689,#6754);
#5863=LINE('',#48690,#6755);
#5864=LINE('',#48695,#6756);
#5865=LINE('',#48702,#6757);
#5866=LINE('',#48704,#6758);
#5867=LINE('',#48705,#6759);
#5868=LINE('',#48708,#6760);
#5869=LINE('',#48711,#6761);
#5870=LINE('',#48714,#6762);
#5871=LINE('',#48735,#6763);
#5872=LINE('',#48744,#6764);
#5873=LINE('',#48750,#6765);
#5874=LINE('',#48755,#6766);
#5875=LINE('',#48765,#6767);
#5876=LINE('',#48768,#6768);
#5877=LINE('',#48770,#6769);
#5878=LINE('',#48774,#6770);
#5879=LINE('',#48777,#6771);
#5880=LINE('',#48782,#6772);
#5881=LINE('',#48785,#6773);
#5882=LINE('',#48789,#6774);
#5883=LINE('',#48790,#6775);
#5884=LINE('',#48803,#6776);
#5885=LINE('',#48818,#6777);
#5886=LINE('',#48836,#6778);
#5887=LINE('',#48839,#6779);
#5888=LINE('',#48840,#6780);
#5889=LINE('',#48843,#6781);
#5890=LINE('',#48849,#6782);
#5891=LINE('',#48851,#6783);
#5892=LINE('',#48853,#6784);
#5893=LINE('',#48854,#6785);
#5894=LINE('',#48863,#6786);
#5895=LINE('',#48873,#6787);
#5896=LINE('',#48911,#6788);
#5897=LINE('',#48921,#6789);
#5898=LINE('',#48937,#6790);
#5899=LINE('',#48951,#6791);
#5900=LINE('',#48964,#6792);
#5901=LINE('',#48977,#6793);
#5902=LINE('',#48983,#6794);
#5903=LINE('',#48986,#6795);
#5904=LINE('',#48989,#6796);
#5905=LINE('',#48994,#6797);
#5906=LINE('',#48996,#6798);
#5907=LINE('',#49003,#6799);
#5908=LINE('',#49042,#6800);
#5909=LINE('',#49050,#6801);
#5910=LINE('',#49085,#6802);
#5911=LINE('',#49097,#6803);
#5912=LINE('',#49113,#6804);
#5913=LINE('',#49124,#6805);
#5914=LINE('',#49163,#6806);
#5915=LINE('',#49164,#6807);
#5916=LINE('',#49172,#6808);
#5917=LINE('',#49180,#6809);
#5918=LINE('',#49188,#6810);
#5919=LINE('',#49197,#6811);
#5920=LINE('',#49204,#6812);
#5921=LINE('',#49212,#6813);
#5922=LINE('',#49220,#6814);
#5923=LINE('',#49222,#6815);
#5924=LINE('',#49224,#6816);
#5925=LINE('',#49226,#6817);
#6536=VECTOR('',#23439,10.);
#6537=VECTOR('',#23442,10.);
#6538=VECTOR('',#23455,10.);
#6539=VECTOR('',#23458,10.);
#6540=VECTOR('',#23463,10.);
#6541=VECTOR('',#23466,10.);
#6542=VECTOR('',#23485,10.);
#6543=VECTOR('',#23486,10.);
#6544=VECTOR('',#23491,10.);
#6545=VECTOR('',#23494,10.);
#6546=VECTOR('',#23501,10.);
#6547=VECTOR('',#23504,10.);
#6548=VECTOR('',#23507,10.);
#6549=VECTOR('',#23510,10.);
#6550=VECTOR('',#23515,10.);
#6551=VECTOR('',#23516,10.);
#6552=VECTOR('',#23519,10.);
#6553=VECTOR('',#23524,10.);
#6554=VECTOR('',#23527,10.);
#6555=VECTOR('',#23528,10.);
#6556=VECTOR('',#23531,10.);
#6557=VECTOR('',#23540,10.);
#6558=VECTOR('',#23547,10.);
#6559=VECTOR('',#23554,10.);
#6560=VECTOR('',#23557,10.);
#6561=VECTOR('',#23564,10.);
#6562=VECTOR('',#23567,10.);
#6563=VECTOR('',#23572,10.);
#6564=VECTOR('',#23581,10.);
#6565=VECTOR('',#23584,10.);
#6566=VECTOR('',#23587,10.);
#6567=VECTOR('',#23588,10.);
#6568=VECTOR('',#23589,10.);
#6569=VECTOR('',#23602,10.);
#6570=VECTOR('',#23605,10.);
#6571=VECTOR('',#23610,10.);
#6572=VECTOR('',#23613,10.);
#6573=VECTOR('',#23616,10.);
#6574=VECTOR('',#23619,10.);
#6575=VECTOR('',#23624,10.);
#6576=VECTOR('',#23625,10.);
#6577=VECTOR('',#23632,10.);
#6578=VECTOR('',#23633,10.);
#6579=VECTOR('',#23636,10.);
#6580=VECTOR('',#23641,10.);
#6581=VECTOR('',#23646,10.);
#6582=VECTOR('',#23649,10.);
#6583=VECTOR('',#23652,10.);
#6584=VECTOR('',#23653,10.);
#6585=VECTOR('',#23654,10.);
#6586=VECTOR('',#23655,10.);
#6587=VECTOR('',#23666,10.);
#6588=VECTOR('',#23675,10.);
#6589=VECTOR('',#23678,10.);
#6590=VECTOR('',#23679,10.);
#6591=VECTOR('',#23686,10.);
#6592=VECTOR('',#23701,10.);
#6593=VECTOR('',#23704,10.);
#6594=VECTOR('',#23709,10.);
#6595=VECTOR('',#23712,10.);
#6596=VECTOR('',#23723,10.);
#6597=VECTOR('',#23724,10.);
#6598=VECTOR('',#23725,10.);
#6599=VECTOR('',#23728,10.);
#6600=VECTOR('',#23729,10.);
#6601=VECTOR('',#23730,10.);
#6602=VECTOR('',#23737,10.);
#6603=VECTOR('',#23746,10.);
#6604=VECTOR('',#23755,10.);
#6605=VECTOR('',#23764,10.);
#6606=VECTOR('',#23769,10.);
#6607=VECTOR('',#23770,10.);
#6608=VECTOR('',#23773,10.);
#6609=VECTOR('',#23778,10.);
#6610=VECTOR('',#23779,10.);
#6611=VECTOR('',#23782,10.);
#6612=VECTOR('',#23787,10.);
#6613=VECTOR('',#23788,10.);
#6614=VECTOR('',#23791,10.);
#6615=VECTOR('',#23798,10.);
#6616=VECTOR('',#23801,10.);
#6617=VECTOR('',#23804,10.);
#6618=VECTOR('',#23807,10.);
#6619=VECTOR('',#23816,10.);
#6620=VECTOR('',#23817,10.);
#6621=VECTOR('',#23818,10.);
#6622=VECTOR('',#23821,10.);
#6623=VECTOR('',#23826,10.);
#6624=VECTOR('',#23827,10.);
#6625=VECTOR('',#23836,10.);
#6626=VECTOR('',#23837,10.);
#6627=VECTOR('',#23842,10.);
#6628=VECTOR('',#23845,10.);
#6629=VECTOR('',#23854,10.);
#6630=VECTOR('',#23861,10.);
#6631=VECTOR('',#23870,10.);
#6632=VECTOR('',#23875,10.);
#6633=VECTOR('',#23878,10.);
#6634=VECTOR('',#23879,10.);
#6635=VECTOR('',#23886,10.);
#6636=VECTOR('',#23893,10.);
#6637=VECTOR('',#23898,10.);
#6638=VECTOR('',#23899,10.);
#6639=VECTOR('',#23910,10.);
#6640=VECTOR('',#23913,10.);
#6641=VECTOR('',#23920,10.);
#6642=VECTOR('',#23923,10.);
#6643=VECTOR('',#23932,10.);
#6644=VECTOR('',#23933,10.);
#6645=VECTOR('',#23934,10.);
#6646=VECTOR('',#23937,10.);
#6647=VECTOR('',#23944,10.);
#6648=VECTOR('',#23945,0.5);
#6649=VECTOR('',#23950,10.);
#6650=VECTOR('',#23957,10.);
#6651=VECTOR('',#23960,10.);
#6652=VECTOR('',#23965,10.);
#6653=VECTOR('',#23968,10.);
#6654=VECTOR('',#23987,10.);
#6655=VECTOR('',#23990,10.);
#6656=VECTOR('',#23993,10.);
#6657=VECTOR('',#23996,10.);
#6658=VECTOR('',#23999,10.);
#6659=VECTOR('',#24002,10.);
#6660=VECTOR('',#24005,10.);
#6661=VECTOR('',#24006,10.);
#6662=VECTOR('',#24009,10.);
#6663=VECTOR('',#24016,10.);
#6664=VECTOR('',#24019,10.);
#6665=VECTOR('',#24034,0.5);
#6666=VECTOR('',#24035,0.5);
#6667=VECTOR('',#24040,10.);
#6668=VECTOR('',#24045,10.);
#6669=VECTOR('',#24046,10.);
#6670=VECTOR('',#24049,10.);
#6671=VECTOR('',#24054,10.);
#6672=VECTOR('',#24055,10.);
#6673=VECTOR('',#24064,10.);
#6674=VECTOR('',#24065,10.);
#6675=VECTOR('',#24070,10.);
#6676=VECTOR('',#24073,10.);
#6677=VECTOR('',#24076,10.);
#6678=VECTOR('',#24081,10.);
#6679=VECTOR('',#24084,10.);
#6680=VECTOR('',#24091,10.);
#6681=VECTOR('',#24098,10.);
#6682=VECTOR('',#24101,10.);
#6683=VECTOR('',#24102,10.);
#6684=VECTOR('',#24109,10.);
#6685=VECTOR('',#24112,10.);
#6686=VECTOR('',#24115,10.);
#6687=VECTOR('',#24116,10.);
#6688=VECTOR('',#24117,10.);
#6689=VECTOR('',#24130,10.);
#6690=VECTOR('',#24137,10.);
#6691=VECTOR('',#24150,10.);
#6692=VECTOR('',#24161,10.);
#6693=VECTOR('',#24178,44.);
#6694=VECTOR('',#24181,10.);
#6695=VECTOR('',#24184,10.);
#6696=VECTOR('',#24187,10.);
#6697=VECTOR('',#24190,10.);
#6698=VECTOR('',#24193,10.);
#6699=VECTOR('',#24196,10.);
#6700=VECTOR('',#24199,10.);
#6701=VECTOR('',#24202,10.);
#6702=VECTOR('',#24211,10.);
#6703=VECTOR('',#24214,10.);
#6704=VECTOR('',#24227,10.);
#6705=VECTOR('',#24228,10.);
#6706=VECTOR('',#24251,10.);
#6707=VECTOR('',#24254,10.);
#6708=VECTOR('',#24257,10.);
#6709=VECTOR('',#24260,10.);
#6710=VECTOR('',#24263,10.);
#6711=VECTOR('',#24266,10.);
#6712=VECTOR('',#24287,10.);
#6713=VECTOR('',#24292,10.);
#6714=VECTOR('',#24303,10.);
#6715=VECTOR('',#24318,10.);
#6716=VECTOR('',#24319,10.);
#6717=VECTOR('',#24320,10.);
#6718=VECTOR('',#24327,10.);
#6719=VECTOR('',#24344,10.);
#6720=VECTOR('',#24355,10.);
#6721=VECTOR('',#24356,10.);
#6722=VECTOR('',#24357,10.);
#6723=VECTOR('',#24368,10.);
#6724=VECTOR('',#24369,10.);
#6725=VECTOR('',#24376,10.);
#6726=VECTOR('',#24377,10.);
#6727=VECTOR('',#24392,10.);
#6728=VECTOR('',#24397,10.);
#6729=VECTOR('',#24398,10.);
#6730=VECTOR('',#24399,10.);
#6731=VECTOR('',#24406,10.);
#6732=VECTOR('',#24437,10.);
#6733=VECTOR('',#24440,10.);
#6734=VECTOR('',#24453,10.);
#6735=VECTOR('',#24462,10.);
#6736=VECTOR('',#24473,10.);
#6737=VECTOR('',#24480,10.);
#6738=VECTOR('',#24483,10.);
#6739=VECTOR('',#24484,10.);
#6740=VECTOR('',#24485,10.);
#6741=VECTOR('',#24506,1.25);
#6742=VECTOR('',#24523,10.);
#6743=VECTOR('',#24524,10.);
#6744=VECTOR('',#24527,10.);
#6745=VECTOR('',#24528,10.);
#6746=VECTOR('',#24529,10.);
#6747=VECTOR('',#24530,10.);
#6748=VECTOR('',#24531,10.);
#6749=VECTOR('',#24534,10.);
#6750=VECTOR('',#24541,10.);
#6751=VECTOR('',#24546,10.);
#6752=VECTOR('',#24551,0.5);
#6753=VECTOR('',#24554,0.5);
#6754=VECTOR('',#24559,0.5);
#6755=VECTOR('',#24560,10.);
#6756=VECTOR('',#24565,0.5);
#6757=VECTOR('',#24576,10.);
#6758=VECTOR('',#24577,10.);
#6759=VECTOR('',#24578,10.);
#6760=VECTOR('',#24581,10.);
#6761=VECTOR('',#24584,10.);
#6762=VECTOR('',#24587,10.);
#6763=VECTOR('',#24608,1.25);
#6764=VECTOR('',#24619,10.);
#6765=VECTOR('',#24628,10.);
#6766=VECTOR('',#24635,10.);
#6767=VECTOR('',#24648,10.);
#6768=VECTOR('',#24651,10.);
#6769=VECTOR('',#24654,10.);
#6770=VECTOR('',#24659,10.);
#6771=VECTOR('',#24662,10.);
#6772=VECTOR('',#24671,10.);
#6773=VECTOR('',#24674,10.);
#6774=VECTOR('',#24679,10.);
#6775=VECTOR('',#24680,0.5);
#6776=VECTOR('',#24695,44.);
#6777=VECTOR('',#24714,43.6);
#6778=VECTOR('',#24743,10.);
#6779=VECTOR('',#24746,10.);
#6780=VECTOR('',#24747,10.);
#6781=VECTOR('',#24750,10.);
#6782=VECTOR('',#24759,10.);
#6783=VECTOR('',#24760,10.);
#6784=VECTOR('',#24761,10.);
#6785=VECTOR('',#24762,10.);
#6786=VECTOR('',#24775,1.25);
#6787=VECTOR('',#24788,1.25);
#6788=VECTOR('',#24831,3.);
#6789=VECTOR('',#24844,3.);
#6790=VECTOR('',#24869,3.);
#6791=VECTOR('',#24890,3.);
#6792=VECTOR('',#24907,3.);
#6793=VECTOR('',#24924,3.);
#6794=VECTOR('',#24931,10.);
#6795=VECTOR('',#24934,10.);
#6796=VECTOR('',#24939,10.);
#6797=VECTOR('',#24946,10.);
#6798=VECTOR('',#24947,10.);
#6799=VECTOR('',#24948,10.);
#6800=VECTOR('',#24967,43.7);
#6801=VECTOR('',#24976,44.);
#6802=VECTOR('',#25023,7.05);
#6803=VECTOR('',#25038,7.3);
#6804=VECTOR('',#25059,12.);
#6805=VECTOR('',#25074,43.7);
#6806=VECTOR('',#25107,10.);
#6807=VECTOR('',#25108,10.);
#6808=VECTOR('',#25117,5.);
#6809=VECTOR('',#25128,5.);
#6810=VECTOR('',#25139,5.);
#6811=VECTOR('',#25150,12.25);
#6812=VECTOR('',#25161,10.);
#6813=VECTOR('',#25176,10.);
#6814=VECTOR('',#25191,42.4);
#6815=VECTOR('',#25194,4.5);
#6816=VECTOR('',#25197,4.5);
#6817=VECTOR('',#25200,4.5);
#7756=VERTEX_POINT('',#47241);
#7757=VERTEX_POINT('',#47242);
#7758=VERTEX_POINT('',#47244);
#7759=VERTEX_POINT('',#47246);
#7760=VERTEX_POINT('',#47250);
#7761=VERTEX_POINT('',#47251);
#7762=VERTEX_POINT('',#47256);
#7763=VERTEX_POINT('',#47257);
#7764=VERTEX_POINT('',#47260);
#7765=VERTEX_POINT('',#47264);
#7766=VERTEX_POINT('',#47265);
#7767=VERTEX_POINT('',#47267);
#7768=VERTEX_POINT('',#47274);
#7769=VERTEX_POINT('',#47275);
#7770=VERTEX_POINT('',#47277);
#7771=VERTEX_POINT('',#47279);
#7772=VERTEX_POINT('',#47283);
#7773=VERTEX_POINT('',#47284);
#7774=VERTEX_POINT('',#47289);
#7775=VERTEX_POINT('',#47291);
#7776=VERTEX_POINT('',#47298);
#7777=VERTEX_POINT('',#47300);
#7778=VERTEX_POINT('',#47306);
#7779=VERTEX_POINT('',#47310);
#7780=VERTEX_POINT('',#47314);
#7781=VERTEX_POINT('',#47323);
#7782=VERTEX_POINT('',#47335);
#7783=VERTEX_POINT('',#47336);
#7784=VERTEX_POINT('',#47343);
#7785=VERTEX_POINT('',#47345);
#7786=VERTEX_POINT('',#47347);
#7787=VERTEX_POINT('',#47354);
#7788=VERTEX_POINT('',#47356);
#7789=VERTEX_POINT('',#47358);
#7790=VERTEX_POINT('',#47362);
#7791=VERTEX_POINT('',#47368);
#7792=VERTEX_POINT('',#47370);
#7793=VERTEX_POINT('',#47374);
#7794=VERTEX_POINT('',#47376);
#7795=VERTEX_POINT('',#47380);
#7796=VERTEX_POINT('',#47381);
#7797=VERTEX_POINT('',#47384);
#7798=VERTEX_POINT('',#47390);
#7799=VERTEX_POINT('',#47392);
#7800=VERTEX_POINT('',#47406);
#7801=VERTEX_POINT('',#47408);
#7802=VERTEX_POINT('',#47412);
#7803=VERTEX_POINT('',#47414);
#7804=VERTEX_POINT('',#47418);
#7805=VERTEX_POINT('',#47425);
#7806=VERTEX_POINT('',#47429);
#7807=VERTEX_POINT('',#47436);
#7808=VERTEX_POINT('',#47438);
#7809=VERTEX_POINT('',#47442);
#7810=VERTEX_POINT('',#47444);
#7811=VERTEX_POINT('',#47446);
#7812=VERTEX_POINT('',#47450);
#7813=VERTEX_POINT('',#47452);
#7814=VERTEX_POINT('',#47461);
#7815=VERTEX_POINT('',#47467);
#7816=VERTEX_POINT('',#47471);
#7817=VERTEX_POINT('',#47473);
#7818=VERTEX_POINT('',#47478);
#7819=VERTEX_POINT('',#47491);
#7820=VERTEX_POINT('',#47506);
#7821=VERTEX_POINT('',#47507);
#7822=VERTEX_POINT('',#47509);
#7823=VERTEX_POINT('',#47511);
#7824=VERTEX_POINT('',#47515);
#7825=VERTEX_POINT('',#47517);
#7826=VERTEX_POINT('',#47519);
#7827=VERTEX_POINT('',#47523);
#7828=VERTEX_POINT('',#47524);
#7829=VERTEX_POINT('',#47529);
#7830=VERTEX_POINT('',#47531);
#7831=VERTEX_POINT('',#47535);
#7832=VERTEX_POINT('',#47537);
#7833=VERTEX_POINT('',#47541);
#7834=VERTEX_POINT('',#47543);
#7835=VERTEX_POINT('',#47549);
#7836=VERTEX_POINT('',#47551);
#7837=VERTEX_POINT('',#47557);
#7838=VERTEX_POINT('',#47563);
#7839=VERTEX_POINT('',#47567);
#7840=VERTEX_POINT('',#47571);
#7841=VERTEX_POINT('',#47575);
#7842=VERTEX_POINT('',#47579);
#7843=VERTEX_POINT('',#47583);
#7844=VERTEX_POINT('',#47587);
#7845=VERTEX_POINT('',#47591);
#7846=VERTEX_POINT('',#47592);
#7847=VERTEX_POINT('',#47594);
#7848=VERTEX_POINT('',#47596);
#7849=VERTEX_POINT('',#47600);
#7850=VERTEX_POINT('',#47601);
#7851=VERTEX_POINT('',#47613);
#7852=VERTEX_POINT('',#47616);
#7853=VERTEX_POINT('',#47622);
#7854=VERTEX_POINT('',#47624);
#7855=VERTEX_POINT('',#47628);
#7856=VERTEX_POINT('',#47632);
#7857=VERTEX_POINT('',#47637);
#7858=VERTEX_POINT('',#47639);
#7859=VERTEX_POINT('',#47646);
#7860=VERTEX_POINT('',#47653);
#7861=VERTEX_POINT('',#47665);
#7862=VERTEX_POINT('',#47669);
#7863=VERTEX_POINT('',#47673);
#7864=VERTEX_POINT('',#47675);
#7865=VERTEX_POINT('',#47679);
#7866=VERTEX_POINT('',#47686);
#7867=VERTEX_POINT('',#47697);
#7868=VERTEX_POINT('',#47703);
#7869=VERTEX_POINT('',#47707);
#7870=VERTEX_POINT('',#47715);
#7871=VERTEX_POINT('',#47716);
#7872=VERTEX_POINT('',#47725);
#7873=VERTEX_POINT('',#47727);
#7874=VERTEX_POINT('',#47729);
#7875=VERTEX_POINT('',#47733);
#7876=VERTEX_POINT('',#47734);
#7877=VERTEX_POINT('',#47736);
#7878=VERTEX_POINT('',#47739);
#7879=VERTEX_POINT('',#47745);
#7880=VERTEX_POINT('',#47747);
#7881=VERTEX_POINT('',#47751);
#7882=VERTEX_POINT('',#47753);
#7883=VERTEX_POINT('',#47757);
#7884=VERTEX_POINT('',#47761);
#7885=VERTEX_POINT('',#47763);
#7886=VERTEX_POINT('',#47767);
#7887=VERTEX_POINT('',#47769);
#7888=VERTEX_POINT('',#47771);
#7889=VERTEX_POINT('',#47775);
#7890=VERTEX_POINT('',#47776);
#7891=VERTEX_POINT('',#47778);
#7892=VERTEX_POINT('',#47780);
#7893=VERTEX_POINT('',#47784);
#7894=VERTEX_POINT('',#47785);
#7895=VERTEX_POINT('',#47790);
#7896=VERTEX_POINT('',#47791);
#7897=VERTEX_POINT('',#47796);
#7898=VERTEX_POINT('',#47798);
#7899=VERTEX_POINT('',#47802);
#7900=VERTEX_POINT('',#47804);
#7901=VERTEX_POINT('',#47808);
#7902=VERTEX_POINT('',#47810);
#7903=VERTEX_POINT('',#47814);
#7904=VERTEX_POINT('',#47818);
#7905=VERTEX_POINT('',#47822);
#7906=VERTEX_POINT('',#47823);
#7907=VERTEX_POINT('',#47825);
#7908=VERTEX_POINT('',#47830);
#7909=VERTEX_POINT('',#47836);
#7910=VERTEX_POINT('',#47837);
#7911=VERTEX_POINT('',#47840);
#7912=VERTEX_POINT('',#47844);
#7913=VERTEX_POINT('',#47848);
#7914=VERTEX_POINT('',#47852);
#7915=VERTEX_POINT('',#47856);
#7916=VERTEX_POINT('',#47860);
#7917=VERTEX_POINT('',#47868);
#7918=VERTEX_POINT('',#47870);
#7919=VERTEX_POINT('',#47876);
#7920=VERTEX_POINT('',#47878);
#7921=VERTEX_POINT('',#47885);
#7922=VERTEX_POINT('',#47889);
#7923=VERTEX_POINT('',#47897);
#7924=VERTEX_POINT('',#47898);
#7925=VERTEX_POINT('',#47900);
#7926=VERTEX_POINT('',#47902);
#7927=VERTEX_POINT('',#47907);
#7928=VERTEX_POINT('',#47911);
#7929=VERTEX_POINT('',#47921);
#7930=VERTEX_POINT('',#47934);
#7931=VERTEX_POINT('',#47936);
#7932=VERTEX_POINT('',#47952);
#7933=VERTEX_POINT('',#47965);
#7934=VERTEX_POINT('',#47966);
#7935=VERTEX_POINT('',#47968);
#7936=VERTEX_POINT('',#47973);
#7937=VERTEX_POINT('',#47975);
#7938=VERTEX_POINT('',#47977);
#7939=VERTEX_POINT('',#47979);
#7940=VERTEX_POINT('',#47981);
#7941=VERTEX_POINT('',#47983);
#7942=VERTEX_POINT('',#47985);
#7943=VERTEX_POINT('',#47987);
#7944=VERTEX_POINT('',#47989);
#7945=VERTEX_POINT('',#47991);
#7946=VERTEX_POINT('',#47993);
#7947=VERTEX_POINT('',#47995);
#7948=VERTEX_POINT('',#47997);
#7949=VERTEX_POINT('',#47999);
#7950=VERTEX_POINT('',#48001);
#7951=VERTEX_POINT('',#48003);
#7952=VERTEX_POINT('',#48005);
#7953=VERTEX_POINT('',#48009);
#7954=VERTEX_POINT('',#48012);
#7955=VERTEX_POINT('',#48013);
#7956=VERTEX_POINT('',#48024);
#7957=VERTEX_POINT('',#48026);
#7958=VERTEX_POINT('',#48028);
#7959=VERTEX_POINT('',#48041);
#7960=VERTEX_POINT('',#48042);
#7961=VERTEX_POINT('',#48047);
#7962=VERTEX_POINT('',#48048);
#7963=VERTEX_POINT('',#48053);
#7964=VERTEX_POINT('',#48057);
#7965=VERTEX_POINT('',#48058);
#7966=VERTEX_POINT('',#48060);
#7967=VERTEX_POINT('',#48062);
#7968=VERTEX_POINT('',#48103);
#7969=VERTEX_POINT('',#48105);
#7970=VERTEX_POINT('',#48107);
#7971=VERTEX_POINT('',#48109);
#7972=VERTEX_POINT('',#48111);
#7973=VERTEX_POINT('',#48113);
#7974=VERTEX_POINT('',#48115);
#7975=VERTEX_POINT('',#48117);
#7976=VERTEX_POINT('',#48119);
#7977=VERTEX_POINT('',#48121);
#7978=VERTEX_POINT('',#48123);
#7979=VERTEX_POINT('',#48125);
#7980=VERTEX_POINT('',#48128);
#7981=VERTEX_POINT('',#48131);
#7982=VERTEX_POINT('',#48135);
#7983=VERTEX_POINT('',#48144);
#7984=VERTEX_POINT('',#48146);
#7985=VERTEX_POINT('',#48163);
#7986=VERTEX_POINT('',#48164);
#7987=VERTEX_POINT('',#48175);
#7988=VERTEX_POINT('',#48189);
#7989=VERTEX_POINT('',#48193);
#7990=VERTEX_POINT('',#48200);
#7991=VERTEX_POINT('',#48204);
#7992=VERTEX_POINT('',#48208);
#7993=VERTEX_POINT('',#48215);
#7994=VERTEX_POINT('',#48219);
#7995=VERTEX_POINT('',#48224);
#7996=VERTEX_POINT('',#48226);
#7997=VERTEX_POINT('',#48233);
#7998=VERTEX_POINT('',#48237);
#7999=VERTEX_POINT('',#48250);
#8000=VERTEX_POINT('',#48252);
#8001=VERTEX_POINT('',#48306);
#8002=VERTEX_POINT('',#48307);
#8003=VERTEX_POINT('',#48313);
#8004=VERTEX_POINT('',#48322);
#8005=VERTEX_POINT('',#48337);
#8006=VERTEX_POINT('',#48340);
#8007=VERTEX_POINT('',#48345);
#8008=VERTEX_POINT('',#48348);
#8009=VERTEX_POINT('',#48352);
#8010=VERTEX_POINT('',#48357);
#8011=VERTEX_POINT('',#48359);
#8012=VERTEX_POINT('',#48366);
#8013=VERTEX_POINT('',#48390);
#8014=VERTEX_POINT('',#48412);
#8015=VERTEX_POINT('',#48431);
#8016=VERTEX_POINT('',#48433);
#8017=VERTEX_POINT('',#48444);
#8018=VERTEX_POINT('',#48448);
#8019=VERTEX_POINT('',#48450);
#8020=VERTEX_POINT('',#48457);
#8021=VERTEX_POINT('',#48470);
#8022=VERTEX_POINT('',#48472);
#8023=VERTEX_POINT('',#48498);
#8024=VERTEX_POINT('',#48499);
#8025=VERTEX_POINT('',#48501);
#8026=VERTEX_POINT('',#48517);
#8027=VERTEX_POINT('',#48521);
#8028=VERTEX_POINT('',#48528);
#8029=VERTEX_POINT('',#48537);
#8030=VERTEX_POINT('',#48539);
#8031=VERTEX_POINT('',#48542);
#8032=VERTEX_POINT('',#48545);
#8033=VERTEX_POINT('',#48576);
#8034=VERTEX_POINT('',#48583);
#8035=VERTEX_POINT('',#48598);
#8036=VERTEX_POINT('',#48604);
#8037=VERTEX_POINT('',#48608);
#8038=VERTEX_POINT('',#48618);
#8039=VERTEX_POINT('',#48620);
#8040=VERTEX_POINT('',#48630);
#8041=VERTEX_POINT('',#48634);
#8042=VERTEX_POINT('',#48636);
#8043=VERTEX_POINT('',#48640);
#8044=VERTEX_POINT('',#48641);
#8045=VERTEX_POINT('',#48643);
#8046=VERTEX_POINT('',#48647);
#8047=VERTEX_POINT('',#48648);
#8048=VERTEX_POINT('',#48653);
#8049=VERTEX_POINT('',#48655);
#8050=VERTEX_POINT('',#48657);
#8051=VERTEX_POINT('',#48659);
#8052=VERTEX_POINT('',#48663);
#8053=VERTEX_POINT('',#48667);
#8054=VERTEX_POINT('',#48668);
#8055=VERTEX_POINT('',#48670);
#8056=VERTEX_POINT('',#48672);
#8057=VERTEX_POINT('',#48674);
#8058=VERTEX_POINT('',#48676);
#8059=VERTEX_POINT('',#48680);
#8060=VERTEX_POINT('',#48682);
#8061=VERTEX_POINT('',#48684);
#8062=VERTEX_POINT('',#48688);
#8063=VERTEX_POINT('',#48692);
#8064=VERTEX_POINT('',#48694);
#8065=VERTEX_POINT('',#48701);
#8066=VERTEX_POINT('',#48703);
#8067=VERTEX_POINT('',#48707);
#8068=VERTEX_POINT('',#48709);
#8069=VERTEX_POINT('',#48713);
#8070=VERTEX_POINT('',#48715);
#8071=VERTEX_POINT('',#48727);
#8072=VERTEX_POINT('',#48730);
#8073=VERTEX_POINT('',#48734);
#8074=VERTEX_POINT('',#48736);
#8075=VERTEX_POINT('',#48740);
#8076=VERTEX_POINT('',#48742);
#8077=VERTEX_POINT('',#48748);
#8078=VERTEX_POINT('',#48754);
#8079=VERTEX_POINT('',#48758);
#8080=VERTEX_POINT('',#48759);
#8081=VERTEX_POINT('',#48764);
#8082=VERTEX_POINT('',#48766);
#8083=VERTEX_POINT('',#48772);
#8084=VERTEX_POINT('',#48776);
#8085=VERTEX_POINT('',#48784);
#8086=VERTEX_POINT('',#48788);
#8087=VERTEX_POINT('',#48792);
#8088=VERTEX_POINT('',#48793);
#8089=VERTEX_POINT('',#48795);
#8090=VERTEX_POINT('',#48800);
#8091=VERTEX_POINT('',#48801);
#8092=VERTEX_POINT('',#48806);
#8093=VERTEX_POINT('',#48809);
#8094=VERTEX_POINT('',#48810);
#8095=VERTEX_POINT('',#48815);
#8096=VERTEX_POINT('',#48816);
#8097=VERTEX_POINT('',#48824);
#8098=VERTEX_POINT('',#48829);
#8099=VERTEX_POINT('',#48832);
#8100=VERTEX_POINT('',#48838);
#8101=VERTEX_POINT('',#48842);
#8102=VERTEX_POINT('',#48848);
#8103=VERTEX_POINT('',#48850);
#8104=VERTEX_POINT('',#48852);
#8105=VERTEX_POINT('',#48858);
#8106=VERTEX_POINT('',#48862);
#8107=VERTEX_POINT('',#48864);
#8108=VERTEX_POINT('',#48868);
#8109=VERTEX_POINT('',#48872);
#8110=VERTEX_POINT('',#48874);
#8111=VERTEX_POINT('',#48878);
#8112=VERTEX_POINT('',#48880);
#8113=VERTEX_POINT('',#48882);
#8114=VERTEX_POINT('',#48886);
#8115=VERTEX_POINT('',#48888);
#8116=VERTEX_POINT('',#48890);
#8117=VERTEX_POINT('',#48892);
#8118=VERTEX_POINT('',#48894);
#8119=VERTEX_POINT('',#48896);
#8120=VERTEX_POINT('',#48898);
#8121=VERTEX_POINT('',#48900);
#8122=VERTEX_POINT('',#48902);
#8123=VERTEX_POINT('',#48904);
#8124=VERTEX_POINT('',#48906);
#8125=VERTEX_POINT('',#48909);
#8126=VERTEX_POINT('',#48913);
#8127=VERTEX_POINT('',#48915);
#8128=VERTEX_POINT('',#48919);
#8129=VERTEX_POINT('',#48929);
#8130=VERTEX_POINT('',#48931);
#8131=VERTEX_POINT('',#48935);
#8132=VERTEX_POINT('',#48943);
#8133=VERTEX_POINT('',#48945);
#8134=VERTEX_POINT('',#48949);
#8135=VERTEX_POINT('',#48953);
#8136=VERTEX_POINT('',#48956);
#8137=VERTEX_POINT('',#48958);
#8138=VERTEX_POINT('',#48962);
#8139=VERTEX_POINT('',#48966);
#8140=VERTEX_POINT('',#48969);
#8141=VERTEX_POINT('',#48971);
#8142=VERTEX_POINT('',#48975);
#8143=VERTEX_POINT('',#48979);
#8144=VERTEX_POINT('',#48982);
#8145=VERTEX_POINT('',#48984);
#8146=VERTEX_POINT('',#48993);
#8147=VERTEX_POINT('',#48995);
#8148=VERTEX_POINT('',#48997);
#8149=VERTEX_POINT('',#49002);
#8150=VERTEX_POINT('',#49004);
#8151=VERTEX_POINT('',#49017);
#8152=VERTEX_POINT('',#49031);
#8153=VERTEX_POINT('',#49032);
#8154=VERTEX_POINT('',#49035);
#8155=VERTEX_POINT('',#49037);
#8156=VERTEX_POINT('',#49041);
#8157=VERTEX_POINT('',#49043);
#8158=VERTEX_POINT('',#49047);
#8159=VERTEX_POINT('',#49048);
#8160=VERTEX_POINT('',#49053);
#8161=VERTEX_POINT('',#49057);
#8162=VERTEX_POINT('',#49059);
#8163=VERTEX_POINT('',#49061);
#8164=VERTEX_POINT('',#49063);
#8165=VERTEX_POINT('',#49065);
#8166=VERTEX_POINT('',#49067);
#8167=VERTEX_POINT('',#49069);
#8168=VERTEX_POINT('',#49078);
#8169=VERTEX_POINT('',#49079);
#8170=VERTEX_POINT('',#49084);
#8171=VERTEX_POINT('',#49086);
#8172=VERTEX_POINT('',#49090);
#8173=VERTEX_POINT('',#49091);
#8174=VERTEX_POINT('',#49096);
#8175=VERTEX_POINT('',#49098);
#8176=VERTEX_POINT('',#49104);
#8177=VERTEX_POINT('',#49106);
#8178=VERTEX_POINT('',#49110);
#8179=VERTEX_POINT('',#49111);
#8180=VERTEX_POINT('',#49116);
#8181=VERTEX_POINT('',#49117);
#8182=VERTEX_POINT('',#49122);
#8183=VERTEX_POINT('',#49125);
#8184=VERTEX_POINT('',#49127);
#8185=VERTEX_POINT('',#49138);
#8186=VERTEX_POINT('',#49143);
#8187=VERTEX_POINT('',#49155);
#8188=VERTEX_POINT('',#49157);
#8189=VERTEX_POINT('',#49159);
#8190=VERTEX_POINT('',#49165);
#8191=VERTEX_POINT('',#49167);
#8192=VERTEX_POINT('',#49169);
#8193=VERTEX_POINT('',#49174);
#8194=VERTEX_POINT('',#49176);
#8195=VERTEX_POINT('',#49182);
#8196=VERTEX_POINT('',#49184);
#8197=VERTEX_POINT('',#49190);
#8198=VERTEX_POINT('',#49191);
#8199=VERTEX_POINT('',#49196);
#8200=VERTEX_POINT('',#49198);
#9955=EDGE_CURVE('',#7756,#7757,#3689,.T.);
#9956=EDGE_CURVE('',#7757,#7758,#5644,.T.);
#9957=EDGE_CURVE('',#7758,#7759,#3690,.T.);
#9958=EDGE_CURVE('',#7759,#7756,#5645,.T.);
#9959=EDGE_CURVE('',#7760,#7761,#3691,.T.);
#9960=EDGE_CURVE('',#7761,#7759,#3692,.T.);
#9961=EDGE_CURVE('',#7758,#7760,#3693,.T.);
#9962=EDGE_CURVE('',#7762,#7763,#3694,.T.);
#9963=EDGE_CURVE('',#7763,#7757,#5646,.T.);
#9964=EDGE_CURVE('',#7764,#7757,#3695,.T.);
#9965=EDGE_CURVE('',#7764,#7762,#5647,.T.);
#9966=EDGE_CURVE('',#7765,#7766,#3696,.T.);
#9967=EDGE_CURVE('',#7766,#7767,#5648,.T.);
#9968=EDGE_CURVE('',#7767,#7762,#3697,.T.);
#9969=EDGE_CURVE('',#7762,#7765,#5649,.T.);
#9970=EDGE_CURVE('',#7767,#7763,#3698,.T.);
#9971=EDGE_CURVE('',#7768,#7769,#3699,.T.);
#9972=EDGE_CURVE('',#7768,#7770,#3700,.T.);
#9973=EDGE_CURVE('',#7770,#7771,#3701,.T.);
#9974=EDGE_CURVE('',#7771,#7769,#3702,.T.);
#9975=EDGE_CURVE('',#7772,#7773,#3703,.T.);
#9976=EDGE_CURVE('',#7773,#7771,#5650,.T.);
#9977=EDGE_CURVE('',#7770,#7772,#5651,.T.);
#9978=EDGE_CURVE('',#7774,#7765,#3704,.T.);
#9979=EDGE_CURVE('',#7765,#7775,#5652,.T.);
#9980=EDGE_CURVE('',#7772,#7775,#3705,.T.);
#9981=EDGE_CURVE('',#7772,#7774,#5653,.T.);
#9982=EDGE_CURVE('',#7774,#7766,#3706,.T.);
#9983=EDGE_CURVE('',#7758,#7776,#5654,.T.);
#9984=EDGE_CURVE('',#7776,#7777,#3707,.T.);
#9985=EDGE_CURVE('',#7777,#7760,#5655,.T.);
#9986=EDGE_CURVE('',#7776,#7763,#5656,.T.);
#9987=EDGE_CURVE('',#7767,#7778,#5657,.T.);
#9988=EDGE_CURVE('',#7778,#7776,#3708,.T.);
#9989=EDGE_CURVE('',#7779,#7766,#5658,.T.);
#9990=EDGE_CURVE('',#7778,#7779,#5659,.T.);
#9991=EDGE_CURVE('',#7774,#7780,#5660,.T.);
#9992=EDGE_CURVE('',#7779,#7780,#3709,.T.);
#9993=EDGE_CURVE('',#7780,#7770,#5661,.T.);
#9994=EDGE_CURVE('',#7760,#7768,#5662,.T.);
#9995=EDGE_CURVE('',#7769,#7761,#5663,.T.);
#9996=EDGE_CURVE('',#7768,#7781,#5664,.T.);
#9997=EDGE_CURVE('',#7781,#7780,#3710,.T.);
#9998=EDGE_CURVE('',#7778,#7777,#3711,.T.);
#9999=EDGE_CURVE('',#7781,#7777,#5665,.T.);
#10000=EDGE_CURVE('',#7779,#7781,#3712,.T.);
#10001=EDGE_CURVE('',#7775,#7764,#5666,.T.);
#10002=EDGE_CURVE('',#7782,#7783,#5088,.F.);
#10003=EDGE_CURVE('',#7784,#7783,#200,.T.);
#10004=EDGE_CURVE('',#7785,#7784,#201,.T.);
#10005=EDGE_CURVE('',#7785,#7786,#5667,.T.);
#10006=EDGE_CURVE('',#7786,#7756,#3713,.T.);
#10007=EDGE_CURVE('',#7756,#7782,#5668,.T.);
#10008=EDGE_CURVE('',#7786,#7764,#3714,.T.);
#10009=EDGE_CURVE('',#7787,#7759,#5669,.T.);
#10010=EDGE_CURVE('',#7788,#7787,#3715,.F.);
#10011=EDGE_CURVE('',#7788,#7789,#5670,.T.);
#10012=EDGE_CURVE('',#7782,#7789,#3716,.F.);
#10013=EDGE_CURVE('',#7786,#7790,#5671,.T.);
#10014=EDGE_CURVE('',#7790,#7775,#3717,.T.);
#10015=EDGE_CURVE('',#7790,#7773,#3718,.T.);
#10016=EDGE_CURVE('',#7790,#7791,#5672,.T.);
#10017=EDGE_CURVE('',#7791,#7792,#3719,.F.);
#10018=EDGE_CURVE('',#7792,#7773,#5673,.T.);
#10019=EDGE_CURVE('',#7793,#7785,#5674,.T.);
#10020=EDGE_CURVE('',#7794,#7793,#5675,.T.);
#10021=EDGE_CURVE('',#7791,#7794,#5676,.T.);
#10022=EDGE_CURVE('',#7795,#7796,#3720,.T.);
#10023=EDGE_CURVE('',#7796,#7793,#3721,.T.);
#10024=EDGE_CURVE('',#7793,#7797,#3722,.T.);
#10025=EDGE_CURVE('',#7797,#7795,#3723,.T.);
#10026=EDGE_CURVE('',#7784,#7797,#5677,.F.);
#10027=EDGE_CURVE('',#7796,#7798,#5678,.T.);
#10028=EDGE_CURVE('',#7798,#7799,#5089,.F.);
#10029=EDGE_CURVE('',#7799,#7794,#3724,.F.);
#10030=EDGE_CURVE('',#7795,#7800,#5679,.T.);
#10031=EDGE_CURVE('',#7800,#7801,#3725,.T.);
#10032=EDGE_CURVE('',#7801,#7796,#5680,.T.);
#10033=EDGE_CURVE('',#7797,#7802,#5681,.T.);
#10034=EDGE_CURVE('',#7802,#7803,#3726,.T.);
#10035=EDGE_CURVE('',#7803,#7795,#5682,.T.);
#10036=EDGE_CURVE('',#7804,#7802,#3727,.T.);
#10037=EDGE_CURVE('',#7802,#7783,#5683,.T.);
#10038=EDGE_CURVE('',#7789,#7804,#5684,.T.);
#10039=EDGE_CURVE('',#7804,#7803,#3728,.T.);
#10040=EDGE_CURVE('',#7805,#7803,#5685,.T.);
#10041=EDGE_CURVE('',#7800,#7805,#5686,.T.);
#10042=EDGE_CURVE('',#7804,#7806,#5687,.T.);
#10043=EDGE_CURVE('',#7805,#7806,#3729,.T.);
#10044=EDGE_CURVE('',#7806,#7788,#5688,.T.);
#10045=EDGE_CURVE('',#7771,#7807,#5689,.T.);
#10046=EDGE_CURVE('',#7807,#7808,#3730,.F.);
#10047=EDGE_CURVE('',#7808,#7769,#5690,.T.);
#10048=EDGE_CURVE('',#7809,#7808,#5691,.T.);
#10049=EDGE_CURVE('',#7810,#7809,#5692,.T.);
#10050=EDGE_CURVE('',#7811,#7810,#5693,.T.);
#10051=EDGE_CURVE('',#7761,#7811,#5694,.T.);
#10052=EDGE_CURVE('',#7811,#7812,#202,.F.);
#10053=EDGE_CURVE('',#7812,#7813,#203,.F.);
#10054=EDGE_CURVE('',#7787,#7813,#5090,.T.);
#10055=EDGE_CURVE('',#7814,#7806,#3731,.T.);
#10056=EDGE_CURVE('',#7813,#7814,#5695,.F.);
#10057=EDGE_CURVE('',#7814,#7805,#3732,.T.);
#10058=EDGE_CURVE('',#7800,#7815,#3733,.T.);
#10059=EDGE_CURVE('',#7814,#7815,#5696,.T.);
#10060=EDGE_CURVE('',#7816,#7801,#5697,.T.);
#10061=EDGE_CURVE('',#7817,#7816,#5091,.F.);
#10062=EDGE_CURVE('',#7818,#7817,#5698,.T.);
#10063=EDGE_CURVE('',#7818,#7798,#5092,.T.);
#10064=EDGE_CURVE('',#7810,#7815,#3734,.T.);
#10065=EDGE_CURVE('',#7815,#7812,#5699,.T.);
#10066=EDGE_CURVE('',#7810,#7801,#3735,.T.);
#10067=EDGE_CURVE('',#7819,#7809,#3736,.T.);
#10068=EDGE_CURVE('',#7816,#7819,#5093,.T.);
#10069=EDGE_CURVE('',#7820,#7821,#3737,.T.);
#10070=EDGE_CURVE('',#7821,#7822,#5700,.T.);
#10071=EDGE_CURVE('',#7822,#7823,#3738,.F.);
#10072=EDGE_CURVE('',#7823,#7820,#5701,.T.);
#10073=EDGE_CURVE('',#7824,#7820,#3739,.T.);
#10074=EDGE_CURVE('',#7820,#7825,#5702,.T.);
#10075=EDGE_CURVE('',#7825,#7826,#3740,.T.);
#10076=EDGE_CURVE('',#7826,#7824,#5703,.T.);
#10077=EDGE_CURVE('',#7827,#7828,#3741,.T.);
#10078=EDGE_CURVE('',#7827,#7826,#3742,.T.);
#10079=EDGE_CURVE('',#7825,#7828,#3743,.T.);
#10080=EDGE_CURVE('',#7829,#7821,#5704,.T.);
#10081=EDGE_CURVE('',#7830,#7829,#5705,.T.);
#10082=EDGE_CURVE('',#7822,#7830,#5706,.T.);
#10083=EDGE_CURVE('',#7831,#7826,#5707,.T.);
#10084=EDGE_CURVE('',#7832,#7831,#5708,.T.);
#10085=EDGE_CURVE('',#7824,#7832,#5709,.T.);
#10086=EDGE_CURVE('',#7833,#7824,#3744,.T.);
#10087=EDGE_CURVE('',#7832,#7834,#3745,.T.);
#10088=EDGE_CURVE('',#7834,#7833,#5710,.T.);
#10089=EDGE_CURVE('',#7833,#7821,#3746,.T.);
#10090=EDGE_CURVE('',#7831,#7835,#3747,.T.);
#10091=EDGE_CURVE('',#7835,#7836,#5711,.T.);
#10092=EDGE_CURVE('',#7836,#7832,#3748,.T.);
#10093=EDGE_CURVE('',#7836,#7834,#3749,.T.);
#10094=EDGE_CURVE('',#7827,#7837,#5712,.T.);
#10095=EDGE_CURVE('',#7837,#7831,#3750,.T.);
#10096=EDGE_CURVE('',#7837,#7835,#3751,.T.);
#10097=EDGE_CURVE('',#7833,#7838,#5713,.T.);
#10098=EDGE_CURVE('',#7838,#7829,#3752,.T.);
#10099=EDGE_CURVE('',#7839,#7834,#5714,.T.);
#10100=EDGE_CURVE('',#7838,#7839,#5715,.T.);
#10101=EDGE_CURVE('',#7836,#7840,#5716,.T.);
#10102=EDGE_CURVE('',#7839,#7840,#3753,.T.);
#10103=EDGE_CURVE('',#7841,#7835,#5717,.T.);
#10104=EDGE_CURVE('',#7840,#7841,#5718,.T.);
#10105=EDGE_CURVE('',#7837,#7842,#5719,.T.);
#10106=EDGE_CURVE('',#7841,#7842,#3754,.T.);
#10107=EDGE_CURVE('',#7843,#7827,#5720,.T.);
#10108=EDGE_CURVE('',#7842,#7843,#5721,.T.);
#10109=EDGE_CURVE('',#7828,#7844,#5722,.T.);
#10110=EDGE_CURVE('',#7844,#7843,#3755,.T.);
#10111=EDGE_CURVE('',#7845,#7846,#3756,.T.);
#10112=EDGE_CURVE('',#7846,#7847,#5723,.T.);
#10113=EDGE_CURVE('',#7847,#7848,#204,.F.);
#10114=EDGE_CURVE('',#7848,#7845,#5724,.T.);
#10115=EDGE_CURVE('',#7849,#7850,#5094,.T.);
#10116=EDGE_CURVE('',#7849,#7851,#5725,.T.);
#10117=EDGE_CURVE('',#7851,#7845,#3757,.T.);
#10118=EDGE_CURVE('',#7845,#7852,#5726,.T.);
#10119=EDGE_CURVE('',#7850,#7852,#3758,.T.);
#10120=EDGE_CURVE('',#7851,#7846,#3759,.T.);
#10121=EDGE_CURVE('',#7853,#7846,#5727,.T.);
#10122=EDGE_CURVE('',#7854,#7853,#5728,.T.);
#10123=EDGE_CURVE('',#7847,#7854,#5729,.T.);
#10124=EDGE_CURVE('',#7851,#7855,#5730,.T.);
#10125=EDGE_CURVE('',#7855,#7853,#3760,.T.);
#10126=EDGE_CURVE('',#7856,#7849,#5095,.F.);
#10127=EDGE_CURVE('',#7857,#7856,#5731,.T.);
#10128=EDGE_CURVE('',#7857,#7858,#5096,.T.);
#10129=EDGE_CURVE('',#7855,#7858,#5732,.T.);
#10130=EDGE_CURVE('',#7855,#7859,#3761,.T.);
#10131=EDGE_CURVE('',#7859,#7853,#3762,.T.);
#10132=EDGE_CURVE('',#7852,#7823,#5733,.T.);
#10133=EDGE_CURVE('',#7825,#7848,#5734,.T.);
#10134=EDGE_CURVE('',#7858,#7860,#5097,.F.);
#10135=EDGE_CURVE('',#7860,#7861,#3763,.F.);
#10136=EDGE_CURVE('',#7861,#7859,#5735,.T.);
#10137=EDGE_CURVE('',#7859,#7862,#5736,.T.);
#10138=EDGE_CURVE('',#7862,#7854,#205,.F.);
#10139=EDGE_CURVE('',#7863,#7842,#3764,.T.);
#10140=EDGE_CURVE('',#7864,#7843,#3765,.T.);
#10141=EDGE_CURVE('',#7864,#7863,#5737,.T.);
#10142=EDGE_CURVE('',#7865,#7840,#3766,.T.);
#10143=EDGE_CURVE('',#7841,#7863,#3767,.T.);
#10144=EDGE_CURVE('',#7863,#7865,#5738,.T.);
#10145=EDGE_CURVE('',#7865,#7839,#3768,.T.);
#10146=EDGE_CURVE('',#7866,#7838,#3769,.T.);
#10147=EDGE_CURVE('',#7865,#7866,#5739,.T.);
#10148=EDGE_CURVE('',#7866,#7864,#5740,.T.);
#10149=EDGE_CURVE('',#7847,#7828,#5741,.T.);
#10150=EDGE_CURVE('',#7844,#7854,#5742,.T.);
#10151=EDGE_CURVE('',#7867,#7844,#3770,.T.);
#10152=EDGE_CURVE('',#7862,#7867,#5743,.T.);
#10153=EDGE_CURVE('',#7867,#7864,#3771,.T.);
#10154=EDGE_CURVE('',#7867,#7868,#5744,.T.);
#10155=EDGE_CURVE('',#7868,#7866,#3772,.T.);
#10156=EDGE_CURVE('',#7869,#7861,#5745,.T.);
#10157=EDGE_CURVE('',#7868,#7869,#5746,.T.);
#10158=EDGE_CURVE('',#7868,#7829,#3773,.T.);
#10159=EDGE_CURVE('',#7869,#7830,#3774,.F.);
#10160=EDGE_CURVE('',#7870,#7871,#5098,.T.);
#10161=EDGE_CURVE('',#7870,#7872,#5747,.T.);
#10162=EDGE_CURVE('',#7872,#7873,#3775,.T.);
#10163=EDGE_CURVE('',#7873,#7874,#5748,.T.);
#10164=EDGE_CURVE('',#7871,#7874,#3776,.T.);
#10165=EDGE_CURVE('',#7875,#7876,#206,.T.);
#10166=EDGE_CURVE('',#7876,#7877,#5749,.T.);
#10167=EDGE_CURVE('',#7877,#7872,#3777,.T.);
#10168=EDGE_CURVE('',#7872,#7878,#5750,.T.);
#10169=EDGE_CURVE('',#7878,#7875,#207,.T.);
#10170=EDGE_CURVE('',#7877,#7873,#3778,.T.);
#10171=EDGE_CURVE('',#7879,#7873,#5751,.T.);
#10172=EDGE_CURVE('',#7880,#7879,#5752,.T.);
#10173=EDGE_CURVE('',#7874,#7880,#5753,.T.);
#10174=EDGE_CURVE('',#7877,#7881,#5754,.T.);
#10175=EDGE_CURVE('',#7882,#7881,#208,.T.);
#10176=EDGE_CURVE('',#7879,#7882,#209,.T.);
#10177=EDGE_CURVE('',#7883,#7876,#5755,.T.);
#10178=EDGE_CURVE('',#7881,#7883,#5756,.T.);
#10179=EDGE_CURVE('',#7884,#7875,#210,.T.);
#10180=EDGE_CURVE('',#7884,#7885,#5757,.T.);
#10181=EDGE_CURVE('',#7885,#7883,#3779,.T.);
#10182=EDGE_CURVE('',#7878,#7886,#211,.T.);
#10183=EDGE_CURVE('',#7886,#7887,#5758,.T.);
#10184=EDGE_CURVE('',#7888,#7887,#3780,.T.);
#10185=EDGE_CURVE('',#7888,#7884,#5759,.T.);
#10186=EDGE_CURVE('',#7889,#7890,#3781,.T.);
#10187=EDGE_CURVE('',#7890,#7891,#5760,.T.);
#10188=EDGE_CURVE('',#7891,#7892,#3782,.T.);
#10189=EDGE_CURVE('',#7892,#7889,#5761,.T.);
#10190=EDGE_CURVE('',#7893,#7894,#3783,.T.);
#10191=EDGE_CURVE('',#7893,#7892,#3784,.T.);
#10192=EDGE_CURVE('',#7891,#7894,#3785,.T.);
#10193=EDGE_CURVE('',#7895,#7896,#3786,.T.);
#10194=EDGE_CURVE('',#7896,#7890,#3787,.T.);
#10195=EDGE_CURVE('',#7889,#7895,#3788,.T.);
#10196=EDGE_CURVE('',#7896,#7897,#5762,.T.);
#10197=EDGE_CURVE('',#7897,#7898,#3789,.F.);
#10198=EDGE_CURVE('',#7898,#7890,#5763,.T.);
#10199=EDGE_CURVE('',#7895,#7899,#5764,.T.);
#10200=EDGE_CURVE('',#7900,#7899,#3790,.T.);
#10201=EDGE_CURVE('',#7900,#7896,#5765,.T.);
#10202=EDGE_CURVE('',#7889,#7901,#5766,.T.);
#10203=EDGE_CURVE('',#7901,#7902,#3791,.T.);
#10204=EDGE_CURVE('',#7902,#7895,#5767,.T.);
#10205=EDGE_CURVE('',#7903,#7892,#5768,.T.);
#10206=EDGE_CURVE('',#7901,#7903,#5769,.T.);
#10207=EDGE_CURVE('',#7893,#7904,#5770,.T.);
#10208=EDGE_CURVE('',#7904,#7903,#3792,.T.);
#10209=EDGE_CURVE('',#7905,#7906,#3793,.T.);
#10210=EDGE_CURVE('',#7906,#7907,#5771,.T.);
#10211=EDGE_CURVE('',#7907,#7904,#3794,.T.);
#10212=EDGE_CURVE('',#7904,#7905,#5772,.T.);
#10213=EDGE_CURVE('',#7905,#7908,#3795,.T.);
#10214=EDGE_CURVE('',#7908,#7906,#3796,.T.);
#10215=EDGE_CURVE('',#7907,#7903,#3797,.T.);
#10216=EDGE_CURVE('',#7909,#7910,#212,.T.);
#10217=EDGE_CURVE('',#7910,#7908,#5773,.T.);
#10218=EDGE_CURVE('',#7905,#7911,#5774,.T.);
#10219=EDGE_CURVE('',#7911,#7909,#213,.T.);
#10220=EDGE_CURVE('',#7907,#7912,#5775,.T.);
#10221=EDGE_CURVE('',#7912,#7901,#3798,.T.);
#10222=EDGE_CURVE('',#7913,#7906,#5776,.T.);
#10223=EDGE_CURVE('',#7912,#7913,#5777,.T.);
#10224=EDGE_CURVE('',#7908,#7914,#5778,.T.);
#10225=EDGE_CURVE('',#7913,#7914,#3799,.T.);
#10226=EDGE_CURVE('',#7915,#7910,#5779,.T.);
#10227=EDGE_CURVE('',#7914,#7915,#5780,.T.);
#10228=EDGE_CURVE('',#7916,#7909,#214,.T.);
#10229=EDGE_CURVE('',#7910,#7916,#3800,.T.);
#10230=EDGE_CURVE('',#7894,#7916,#5781,.T.);
#10231=EDGE_CURVE('',#7911,#7893,#5782,.T.);
#10232=EDGE_CURVE('',#7891,#7917,#5783,.T.);
#10233=EDGE_CURVE('',#7917,#7918,#3801,.F.);
#10234=EDGE_CURVE('',#7918,#7894,#5784,.T.);
#10235=EDGE_CURVE('',#7917,#7898,#5785,.T.);
#10236=EDGE_CURVE('',#7919,#7916,#3802,.T.);
#10237=EDGE_CURVE('',#7916,#7920,#5786,.T.);
#10238=EDGE_CURVE('',#7920,#7870,#215,.F.);
#10239=EDGE_CURVE('',#7871,#7919,#5787,.T.);
#10240=EDGE_CURVE('',#7919,#7910,#3803,.T.);
#10241=EDGE_CURVE('',#7919,#7921,#5788,.T.);
#10242=EDGE_CURVE('',#7915,#7921,#3804,.T.);
#10243=EDGE_CURVE('',#7922,#7880,#3805,.F.);
#10244=EDGE_CURVE('',#7921,#7922,#5789,.T.);
#10245=EDGE_CURVE('',#7887,#7918,#5790,.T.);
#10246=EDGE_CURVE('',#7920,#7886,#5791,.T.);
#10247=EDGE_CURVE('',#7923,#7924,#216,.T.);
#10248=EDGE_CURVE('',#7924,#7925,#5792,.T.);
#10249=EDGE_CURVE('',#7925,#7926,#217,.F.);
#10250=EDGE_CURVE('',#7926,#7923,#5793,.T.);
#10251=EDGE_CURVE('',#7925,#7900,#5794,.T.);
#10252=EDGE_CURVE('',#7927,#7924,#5795,.T.);
#10253=EDGE_CURVE('',#7897,#7927,#5796,.T.);
#10254=EDGE_CURVE('',#7923,#7928,#218,.T.);
#10255=EDGE_CURVE('',#7928,#7882,#5099,.T.);
#10256=EDGE_CURVE('',#7924,#7883,#3806,.T.);
#10257=EDGE_CURVE('',#7885,#7924,#3807,.T.);
#10258=EDGE_CURVE('',#7928,#7929,#5797,.T.);
#10259=EDGE_CURVE('',#7929,#7922,#5100,.F.);
#10260=EDGE_CURVE('',#7912,#7902,#3808,.T.);
#10261=EDGE_CURVE('',#7885,#7930,#5798,.T.);
#10262=EDGE_CURVE('',#7930,#7931,#5101,.F.);
#10263=EDGE_CURVE('',#7931,#7927,#3809,.F.);
#10264=EDGE_CURVE('',#7929,#7926,#219,.F.);
#10265=EDGE_CURVE('',#7932,#7914,#3810,.T.);
#10266=EDGE_CURVE('',#7915,#7899,#3811,.T.);
#10267=EDGE_CURVE('',#7899,#7932,#5799,.T.);
#10268=EDGE_CURVE('',#7921,#7900,#3812,.T.);
#10269=EDGE_CURVE('',#7913,#7932,#3813,.T.);
#10270=EDGE_CURVE('',#7932,#7902,#5800,.T.);
#10271=EDGE_CURVE('',#7933,#7934,#3814,.T.);
#10272=EDGE_CURVE('',#7934,#7935,#3815,.T.);
#10273=EDGE_CURVE('',#7935,#7935,#3816,.T.);
#10274=EDGE_CURVE('',#7934,#7933,#3817,.T.);
#10275=EDGE_CURVE('',#7933,#7936,#5801,.T.);
#10276=EDGE_CURVE('',#7937,#7936,#3818,.T.);
#10277=EDGE_CURVE('',#7938,#7937,#5802,.T.);
#10278=EDGE_CURVE('',#7938,#7939,#3819,.T.);
#10279=EDGE_CURVE('',#7940,#7939,#5803,.T.);
#10280=EDGE_CURVE('',#7941,#7940,#3820,.T.);
#10281=EDGE_CURVE('',#7942,#7941,#5804,.T.);
#10282=EDGE_CURVE('',#7942,#7943,#3821,.T.);
#10283=EDGE_CURVE('',#7944,#7943,#5805,.T.);
#10284=EDGE_CURVE('',#7945,#7944,#3822,.T.);
#10285=EDGE_CURVE('',#7946,#7945,#5806,.T.);
#10286=EDGE_CURVE('',#7946,#7947,#3823,.T.);
#10287=EDGE_CURVE('',#7948,#7947,#5807,.T.);
#10288=EDGE_CURVE('',#7949,#7948,#3824,.T.);
#10289=EDGE_CURVE('',#7950,#7949,#5808,.T.);
#10290=EDGE_CURVE('',#7950,#7951,#3825,.T.);
#10291=EDGE_CURVE('',#7952,#7951,#5809,.T.);
#10292=EDGE_CURVE('',#7936,#7952,#3826,.T.);
#10293=EDGE_CURVE('',#7953,#7953,#3827,.T.);
#10294=EDGE_CURVE('',#7954,#7955,#5102,.T.);
#10295=EDGE_CURVE('',#7955,#7956,#5810,.T.);
#10296=EDGE_CURVE('',#7956,#7957,#3828,.T.);
#10297=EDGE_CURVE('',#7957,#7958,#5811,.T.);
#10298=EDGE_CURVE('',#7958,#7954,#5103,.T.);
#10299=EDGE_CURVE('',#7959,#7960,#3829,.T.);
#10300=EDGE_CURVE('',#7960,#7957,#3830,.T.);
#10301=EDGE_CURVE('',#7956,#7959,#3831,.T.);
#10302=EDGE_CURVE('',#7961,#7962,#3832,.T.);
#10303=EDGE_CURVE('',#7962,#7960,#5812,.T.);
#10304=EDGE_CURVE('',#7959,#7961,#5813,.T.);
#10305=EDGE_CURVE('',#7961,#7963,#3833,.T.);
#10306=EDGE_CURVE('',#7963,#7962,#3834,.T.);
#10307=EDGE_CURVE('',#7964,#7965,#3835,.T.);
#10308=EDGE_CURVE('',#7965,#7966,#3836,.T.);
#10309=EDGE_CURVE('',#7967,#7966,#3837,.T.);
#10310=EDGE_CURVE('',#7966,#7945,#3838,.T.);
#10311=EDGE_CURVE('',#7945,#7964,#3839,.T.);
#10312=EDGE_CURVE('',#7964,#7963,#5104,.T.);
#10313=EDGE_CURVE('',#7961,#7965,#5105,.T.);
#10314=EDGE_CURVE('',#7968,#7962,#3840,.T.);
#10315=EDGE_CURVE('',#7969,#7968,#5814,.T.);
#10316=EDGE_CURVE('',#7970,#7969,#3841,.T.);
#10317=EDGE_CURVE('',#7971,#7970,#5815,.T.);
#10318=EDGE_CURVE('',#7972,#7971,#3842,.T.);
#10319=EDGE_CURVE('',#7973,#7972,#5816,.T.);
#10320=EDGE_CURVE('',#7974,#7973,#3843,.T.);
#10321=EDGE_CURVE('',#7975,#7974,#5817,.T.);
#10322=EDGE_CURVE('',#7976,#7975,#3844,.T.);
#10323=EDGE_CURVE('',#7977,#7976,#5818,.T.);
#10324=EDGE_CURVE('',#7978,#7977,#3845,.T.);
#10325=EDGE_CURVE('',#7979,#7978,#5819,.T.);
#10326=EDGE_CURVE('',#7958,#7979,#3846,.T.);
#10327=EDGE_CURVE('',#7980,#7980,#3847,.T.);
#10328=EDGE_CURVE('',#7963,#7981,#3848,.T.);
#10329=EDGE_CURVE('',#7981,#7968,#3849,.T.);
#10330=EDGE_CURVE('',#7982,#7964,#3850,.T.);
#10331=EDGE_CURVE('',#7981,#7982,#5106,.T.);
#10332=EDGE_CURVE('',#7944,#7982,#3851,.T.);
#10333=EDGE_CURVE('',#7965,#7983,#5820,.T.);
#10334=EDGE_CURVE('',#7984,#7983,#3852,.T.);
#10335=EDGE_CURVE('',#7946,#7984,#5107,.T.);
#10336=EDGE_CURVE('',#7985,#7986,#5108,.T.);
#10337=EDGE_CURVE('',#7986,#7987,#5821,.T.);
#10338=EDGE_CURVE('',#7987,#7977,#3853,.T.);
#10339=EDGE_CURVE('',#7976,#7985,#5109,.T.);
#10340=EDGE_CURVE('',#7988,#7978,#3854,.T.);
#10341=EDGE_CURVE('',#7987,#7988,#3855,.T.);
#10342=EDGE_CURVE('',#7989,#7979,#5110,.T.);
#10343=EDGE_CURVE('',#7988,#7990,#5822,.T.);
#10344=EDGE_CURVE('',#7990,#7989,#220,.T.);
#10345=EDGE_CURVE('',#7975,#7991,#3856,.T.);
#10346=EDGE_CURVE('',#7991,#7985,#3857,.T.);
#10347=EDGE_CURVE('',#7989,#7992,#5111,.T.);
#10348=EDGE_CURVE('',#7992,#7954,#3858,.T.);
#10349=EDGE_CURVE('',#7993,#7955,#668,.T.);
#10350=EDGE_CURVE('',#7994,#7993,#5112,.T.);
#10351=EDGE_CURVE('',#7995,#7994,#5823,.T.);
#10352=EDGE_CURVE('',#7996,#7995,#5113,.F.);
#10353=EDGE_CURVE('',#7996,#7997,#5824,.T.);
#10354=EDGE_CURVE('',#7956,#7997,#5825,.T.);
#10355=EDGE_CURVE('',#7998,#7992,#5114,.T.);
#10356=EDGE_CURVE('',#7993,#7998,#3859,.T.);
#10357=EDGE_CURVE('',#7990,#7999,#5826,.T.);
#10358=EDGE_CURVE('',#8000,#7999,#3860,.T.);
#10359=EDGE_CURVE('',#7950,#8000,#5115,.T.);
#10360=EDGE_CURVE('',#7949,#7998,#5116,.T.);
#10361=EDGE_CURVE('',#8001,#8002,#3861,.T.);
#10362=EDGE_CURVE('',#8002,#7991,#5117,.T.);
#10363=EDGE_CURVE('',#7991,#8003,#3862,.T.);
#10364=EDGE_CURVE('',#8003,#8001,#5118,.T.);
#10365=EDGE_CURVE('',#7975,#8003,#3863,.T.);
#10366=EDGE_CURVE('',#7938,#8004,#5119,.T.);
#10367=EDGE_CURVE('',#7937,#8005,#3864,.T.);
#10368=EDGE_CURVE('',#8005,#8001,#3865,.T.);
#10369=EDGE_CURVE('',#8001,#8006,#5827,.T.);
#10370=EDGE_CURVE('',#8004,#8006,#3866,.T.);
#10371=EDGE_CURVE('',#7937,#8002,#3867,.T.);
#10372=EDGE_CURVE('',#8005,#8007,#3868,.T.);
#10373=EDGE_CURVE('',#8008,#7986,#669,.T.);
#10374=EDGE_CURVE('',#8009,#8008,#5120,.T.);
#10375=EDGE_CURVE('',#8010,#8009,#5828,.T.);
#10376=EDGE_CURVE('',#8011,#8010,#5121,.F.);
#10377=EDGE_CURVE('',#8011,#8012,#5829,.T.);
#10378=EDGE_CURVE('',#7987,#8012,#5830,.T.);
#10379=EDGE_CURVE('',#8008,#8002,#3869,.T.);
#10380=EDGE_CURVE('',#7952,#8009,#5122,.T.);
#10381=EDGE_CURVE('',#7951,#8010,#5123,.F.);
#10382=EDGE_CURVE('',#7988,#8013,#5831,.T.);
#10383=EDGE_CURVE('',#8013,#7999,#5832,.T.);
#10384=EDGE_CURVE('',#7948,#7994,#5124,.T.);
#10385=EDGE_CURVE('',#7947,#7995,#5125,.F.);
#10386=EDGE_CURVE('',#7959,#8014,#5833,.T.);
#10387=EDGE_CURVE('',#8014,#7983,#5834,.T.);
#10388=EDGE_CURVE('',#8015,#7981,#3870,.T.);
#10389=EDGE_CURVE('',#7982,#8016,#3871,.T.);
#10390=EDGE_CURVE('',#8016,#8015,#5126,.T.);
#10391=EDGE_CURVE('',#8015,#7968,#3872,.T.);
#10392=EDGE_CURVE('',#7944,#8016,#3873,.T.);
#10393=EDGE_CURVE('',#8015,#8017,#5835,.T.);
#10394=EDGE_CURVE('',#8017,#7969,#3874,.T.);
#10395=EDGE_CURVE('',#8018,#8016,#5836,.T.);
#10396=EDGE_CURVE('',#8019,#8018,#5127,.F.);
#10397=EDGE_CURVE('',#8019,#8020,#5837,.T.);
#10398=EDGE_CURVE('',#8017,#8020,#5838,.T.);
#10399=EDGE_CURVE('',#7943,#8018,#5128,.F.);
#10400=EDGE_CURVE('',#8021,#7940,#3875,.T.);
#10401=EDGE_CURVE('',#7939,#8022,#5129,.F.);
#10402=EDGE_CURVE('',#8022,#8021,#5839,.T.);
#10403=EDGE_CURVE('',#8023,#8024,#3876,.T.);
#10404=EDGE_CURVE('',#8024,#8025,#5130,.T.);
#10405=EDGE_CURVE('',#8025,#8021,#3877,.T.);
#10406=EDGE_CURVE('',#8021,#8023,#5131,.T.);
#10407=EDGE_CURVE('',#8023,#7972,#3878,.T.);
#10408=EDGE_CURVE('',#7972,#8024,#3879,.T.);
#10409=EDGE_CURVE('',#8025,#7940,#3880,.T.);
#10410=EDGE_CURVE('',#8025,#8026,#3881,.T.);
#10411=EDGE_CURVE('',#8026,#7941,#3882,.F.);
#10412=EDGE_CURVE('',#8027,#8024,#3883,.T.);
#10413=EDGE_CURVE('',#8026,#8027,#5132,.T.);
#10414=EDGE_CURVE('',#8004,#8028,#3884,.T.);
#10415=EDGE_CURVE('',#8028,#8022,#5133,.F.);
#10416=EDGE_CURVE('',#8029,#8006,#5840,.T.);
#10417=EDGE_CURVE('',#8030,#8029,#3885,.T.);
#10418=EDGE_CURVE('',#8028,#8030,#5841,.T.);
#10419=EDGE_CURVE('',#8031,#8031,#3886,.T.);
#10420=EDGE_CURVE('',#8032,#8026,#3887,.F.);
#10421=EDGE_CURVE('',#7941,#8032,#3888,.F.);
#10422=EDGE_CURVE('',#8027,#8033,#3889,.T.);
#10423=EDGE_CURVE('',#8033,#8032,#5134,.T.);
#10424=EDGE_CURVE('',#7942,#8034,#5135,.T.);
#10425=EDGE_CURVE('',#8032,#8035,#5842,.T.);
#10426=EDGE_CURVE('',#8034,#8035,#3890,.T.);
#10427=EDGE_CURVE('',#7971,#8027,#3891,.T.);
#10428=EDGE_CURVE('',#8023,#8036,#5843,.T.);
#10429=EDGE_CURVE('',#8036,#7973,#3892,.T.);
#10430=EDGE_CURVE('',#8037,#7974,#3893,.T.);
#10431=EDGE_CURVE('',#8036,#8037,#3894,.T.);
#10432=EDGE_CURVE('',#8037,#8003,#5844,.T.);
#10433=EDGE_CURVE('',#7971,#8033,#3895,.T.);
#10434=EDGE_CURVE('',#8036,#8030,#5845,.T.);
#10435=EDGE_CURVE('',#8038,#8033,#5846,.T.);
#10436=EDGE_CURVE('',#8038,#8039,#5847,.T.);
#10437=EDGE_CURVE('',#8039,#8035,#5848,.T.);
#10438=EDGE_CURVE('',#8038,#7970,#3896,.T.);
#10439=EDGE_CURVE('',#8017,#8038,#3897,.T.);
#10440=EDGE_CURVE('',#8020,#8039,#3898,.T.);
#10441=EDGE_CURVE('',#8031,#8040,#3899,.T.);
#10442=EDGE_CURVE('',#8040,#8040,#3900,.T.);
#10443=EDGE_CURVE('',#8040,#8041,#5849,.T.);
#10444=EDGE_CURVE('',#8042,#8041,#3901,.T.);
#10445=EDGE_CURVE('',#8041,#8042,#3902,.T.);
#10446=EDGE_CURVE('',#8043,#8044,#3903,.T.);
#10447=EDGE_CURVE('',#8044,#8045,#3904,.T.);
#10448=EDGE_CURVE('',#8045,#8043,#3905,.T.);
#10449=EDGE_CURVE('',#8046,#8047,#221,.F.);
#10450=EDGE_CURVE('',#8047,#8044,#5850,.T.);
#10451=EDGE_CURVE('',#8043,#8046,#5851,.T.);
#10452=EDGE_CURVE('',#8046,#8048,#5852,.T.);
#10453=EDGE_CURVE('',#8049,#8043,#5853,.T.);
#10454=EDGE_CURVE('',#8050,#8049,#5854,.T.);
#10455=EDGE_CURVE('',#8051,#8050,#5855,.T.);
#10456=EDGE_CURVE('',#8048,#8051,#5856,.T.);
#10457=EDGE_CURVE('',#8045,#8052,#5857,.T.);
#10458=EDGE_CURVE('',#8052,#8049,#3906,.F.);
#10459=EDGE_CURVE('',#8053,#8054,#222,.T.);
#10460=EDGE_CURVE('',#8054,#8055,#5858,.T.);
#10461=EDGE_CURVE('',#8055,#8056,#223,.T.);
#10462=EDGE_CURVE('',#8056,#8057,#224,.T.);
#10463=EDGE_CURVE('',#8057,#8058,#5859,.T.);
#10464=EDGE_CURVE('',#8058,#8053,#225,.T.);
#10465=EDGE_CURVE('',#8055,#8059,#5860,.T.);
#10466=EDGE_CURVE('',#8060,#8059,#3907,.T.);
#10467=EDGE_CURVE('',#8060,#8061,#5861,.T.);
#10468=EDGE_CURVE('',#8061,#8056,#226,.T.);
#10469=EDGE_CURVE('',#8062,#8054,#5862,.T.);
#10470=EDGE_CURVE('',#8059,#8062,#5863,.T.);
#10471=EDGE_CURVE('',#8053,#8063,#227,.T.);
#10472=EDGE_CURVE('',#8063,#8064,#5864,.T.);
#10473=EDGE_CURVE('',#8062,#8064,#3908,.T.);
#10474=EDGE_CURVE('',#8062,#8048,#3909,.T.);
#10475=EDGE_CURVE('',#8051,#8059,#3910,.T.);
#10476=EDGE_CURVE('',#8065,#8060,#5865,.T.);
#10477=EDGE_CURVE('',#8066,#8065,#5866,.T.);
#10478=EDGE_CURVE('',#8061,#8066,#5867,.T.);
#10479=EDGE_CURVE('',#8067,#8063,#5868,.T.);
#10480=EDGE_CURVE('',#8068,#8067,#228,.T.);
#10481=EDGE_CURVE('',#8064,#8068,#5869,.T.);
#10482=EDGE_CURVE('',#8058,#8069,#5870,.T.);
#10483=EDGE_CURVE('',#8069,#8070,#229,.T.);
#10484=EDGE_CURVE('',#8070,#8067,#5136,.T.);
#10485=EDGE_CURVE('',#7984,#7996,#3911,.T.);
#10486=EDGE_CURVE('',#7997,#8014,#3912,.T.);
#10487=EDGE_CURVE('',#8071,#8071,#3913,.T.);
#10488=EDGE_CURVE('',#8071,#8072,#3914,.T.);
#10489=EDGE_CURVE('',#8072,#8072,#3915,.T.);
#10490=EDGE_CURVE('',#8072,#8073,#5871,.T.);
#10491=EDGE_CURVE('',#8074,#8073,#3916,.T.);
#10492=EDGE_CURVE('',#8073,#8074,#3917,.T.);
#10493=EDGE_CURVE('',#8075,#8051,#3918,.T.);
#10494=EDGE_CURVE('',#8050,#8076,#3919,.F.);
#10495=EDGE_CURVE('',#8076,#8075,#5872,.T.);
#10496=EDGE_CURVE('',#8075,#8060,#3920,.T.);
#10497=EDGE_CURVE('',#8048,#8077,#3921,.T.);
#10498=EDGE_CURVE('',#8077,#8047,#5873,.T.);
#10499=EDGE_CURVE('',#8064,#8077,#3922,.T.);
#10500=EDGE_CURVE('',#8075,#8078,#5874,.T.);
#10501=EDGE_CURVE('',#8078,#8065,#3923,.T.);
#10502=EDGE_CURVE('',#8079,#8080,#3924,.T.);
#10503=EDGE_CURVE('',#8079,#8065,#3925,.T.);
#10504=EDGE_CURVE('',#8078,#8080,#3926,.T.);
#10505=EDGE_CURVE('',#8078,#8081,#5875,.T.);
#10506=EDGE_CURVE('',#8081,#8082,#3927,.F.);
#10507=EDGE_CURVE('',#8082,#8080,#5876,.T.);
#10508=EDGE_CURVE('',#8081,#8076,#5877,.T.);
#10509=EDGE_CURVE('',#8066,#8083,#3928,.T.);
#10510=EDGE_CURVE('',#8083,#8057,#5878,.T.);
#10511=EDGE_CURVE('',#8079,#8084,#5879,.T.);
#10512=EDGE_CURVE('',#8084,#8066,#3929,.T.);
#10513=EDGE_CURVE('',#8084,#8083,#3930,.T.);
#10514=EDGE_CURVE('',#8069,#8083,#5880,.T.);
#10515=EDGE_CURVE('',#8084,#8085,#5881,.T.);
#10516=EDGE_CURVE('',#8085,#8070,#230,.T.);
#10517=EDGE_CURVE('',#8086,#8079,#5882,.T.);
#10518=EDGE_CURVE('',#8085,#8086,#5883,.T.);
#10519=EDGE_CURVE('',#8087,#8088,#3931,.T.);
#10520=EDGE_CURVE('',#8088,#8089,#3932,.T.);
#10521=EDGE_CURVE('',#8089,#8089,#3933,.T.);
#10522=EDGE_CURVE('',#8088,#8087,#3934,.T.);
#10523=EDGE_CURVE('',#8090,#8091,#3935,.T.);
#10524=EDGE_CURVE('',#8090,#8087,#5884,.T.);
#10525=EDGE_CURVE('',#8091,#8090,#3936,.T.);
#10526=EDGE_CURVE('',#8092,#8092,#3937,.T.);
#10527=EDGE_CURVE('',#8093,#8094,#3938,.T.);
#10528=EDGE_CURVE('',#8094,#8093,#3939,.T.);
#10529=EDGE_CURVE('',#8093,#8091,#3940,.T.);
#10530=EDGE_CURVE('',#8095,#8096,#3941,.T.);
#10531=EDGE_CURVE('',#8095,#8094,#5885,.T.);
#10532=EDGE_CURVE('',#8096,#8095,#3942,.T.);
#10533=EDGE_CURVE('',#8000,#8011,#3943,.T.);
#10534=EDGE_CURVE('',#8012,#8013,#3944,.T.);
#10535=EDGE_CURVE('',#8097,#8097,#3945,.T.);
#10536=EDGE_CURVE('',#8034,#8019,#3946,.T.);
#10537=EDGE_CURVE('',#8098,#8098,#3947,.T.);
#10538=EDGE_CURVE('',#8099,#8086,#3948,.T.);
#10539=EDGE_CURVE('',#8068,#8099,#231,.T.);
#10540=EDGE_CURVE('',#8099,#8077,#5886,.T.);
#10541=EDGE_CURVE('',#8100,#8099,#5887,.T.);
#10542=EDGE_CURVE('',#8100,#8047,#5888,.T.);
#10543=EDGE_CURVE('',#8080,#8101,#5889,.T.);
#10544=EDGE_CURVE('',#8101,#8086,#3949,.T.);
#10545=EDGE_CURVE('',#8101,#8099,#3950,.T.);
#10546=EDGE_CURVE('',#8102,#8082,#5890,.T.);
#10547=EDGE_CURVE('',#8103,#8102,#5891,.T.);
#10548=EDGE_CURVE('',#8104,#8103,#5892,.T.);
#10549=EDGE_CURVE('',#8101,#8104,#5893,.T.);
#10550=EDGE_CURVE('',#8104,#8100,#232,.F.);
#10551=EDGE_CURVE('',#8098,#8105,#3951,.T.);
#10552=EDGE_CURVE('',#8105,#8105,#3952,.T.);
#10553=EDGE_CURVE('',#8105,#8106,#5894,.T.);
#10554=EDGE_CURVE('',#8107,#8106,#3953,.T.);
#10555=EDGE_CURVE('',#8106,#8107,#3954,.T.);
#10556=EDGE_CURVE('',#8097,#8108,#3955,.T.);
#10557=EDGE_CURVE('',#8108,#8108,#3956,.T.);
#10558=EDGE_CURVE('',#8108,#8109,#5895,.T.);
#10559=EDGE_CURVE('',#8110,#8109,#3957,.T.);
#10560=EDGE_CURVE('',#8109,#8110,#3958,.T.);
#10561=EDGE_CURVE('',#8111,#8111,#3959,.T.);
#10562=EDGE_CURVE('',#8111,#8112,#3960,.T.);
#10563=EDGE_CURVE('',#8112,#8113,#3961,.T.);
#10564=EDGE_CURVE('',#8113,#8112,#3962,.T.);
#10565=EDGE_CURVE('',#8114,#8114,#3963,.T.);
#10566=EDGE_CURVE('',#8115,#8115,#3964,.T.);
#10567=EDGE_CURVE('',#8116,#8116,#3965,.T.);
#10568=EDGE_CURVE('',#8117,#8117,#3966,.T.);
#10569=EDGE_CURVE('',#8118,#8118,#3967,.T.);
#10570=EDGE_CURVE('',#8119,#8119,#3968,.T.);
#10571=EDGE_CURVE('',#8120,#8120,#3969,.T.);
#10572=EDGE_CURVE('',#8121,#8121,#3970,.T.);
#10573=EDGE_CURVE('',#8122,#8122,#3971,.T.);
#10574=EDGE_CURVE('',#8123,#8123,#3972,.T.);
#10575=EDGE_CURVE('',#8124,#8124,#3973,.T.);
#10576=EDGE_CURVE('',#8125,#8125,#3974,.T.);
#10577=EDGE_CURVE('',#8125,#8113,#5896,.T.);
#10578=EDGE_CURVE('',#8115,#8126,#3975,.T.);
#10579=EDGE_CURVE('',#8126,#8127,#3976,.T.);
#10580=EDGE_CURVE('',#8127,#8126,#3977,.T.);
#10581=EDGE_CURVE('',#8128,#8128,#3978,.T.);
#10582=EDGE_CURVE('',#8128,#8127,#5897,.T.);
#10583=EDGE_CURVE('',#8114,#8096,#3979,.T.);
#10584=EDGE_CURVE('',#8116,#8074,#3980,.T.);
#10585=EDGE_CURVE('',#8124,#8042,#3981,.T.);
#10586=EDGE_CURVE('',#8117,#8129,#3982,.T.);
#10587=EDGE_CURVE('',#8129,#8130,#3983,.T.);
#10588=EDGE_CURVE('',#8130,#8129,#3984,.T.);
#10589=EDGE_CURVE('',#8131,#8131,#3985,.T.);
#10590=EDGE_CURVE('',#8131,#8130,#5898,.T.);
#10591=EDGE_CURVE('',#8123,#8110,#3986,.T.);
#10592=EDGE_CURVE('',#8118,#8107,#3987,.T.);
#10593=EDGE_CURVE('',#8132,#8132,#3988,.T.);
#10594=EDGE_CURVE('',#8132,#8133,#3989,.T.);
#10595=EDGE_CURVE('',#8133,#8133,#3990,.T.);
#10596=EDGE_CURVE('',#8134,#8134,#3991,.T.);
#10597=EDGE_CURVE('',#8134,#8132,#5899,.T.);
#10598=EDGE_CURVE('',#8135,#8135,#3992,.T.);
#10599=EDGE_CURVE('',#8136,#8136,#3993,.T.);
#10600=EDGE_CURVE('',#8136,#8137,#3994,.T.);
#10601=EDGE_CURVE('',#8137,#8137,#3995,.T.);
#10602=EDGE_CURVE('',#8138,#8138,#3996,.T.);
#10603=EDGE_CURVE('',#8138,#8136,#5900,.T.);
#10604=EDGE_CURVE('',#8139,#8139,#3997,.T.);
#10605=EDGE_CURVE('',#8140,#8140,#3998,.T.);
#10606=EDGE_CURVE('',#8140,#8141,#3999,.T.);
#10607=EDGE_CURVE('',#8141,#8141,#4000,.T.);
#10608=EDGE_CURVE('',#8142,#8142,#4001,.T.);
#10609=EDGE_CURVE('',#8142,#8140,#5901,.T.);
#10610=EDGE_CURVE('',#8143,#8143,#4002,.T.);
#10611=EDGE_CURVE('',#8044,#8144,#5902,.T.);
#10612=EDGE_CURVE('',#8144,#8145,#4003,.T.);
#10613=EDGE_CURVE('',#8145,#8045,#5903,.T.);
#10614=EDGE_CURVE('',#8103,#8144,#4004,.T.);
#10615=EDGE_CURVE('',#8144,#8100,#5904,.T.);
#10616=EDGE_CURVE('',#8103,#8145,#4005,.T.);
#10617=EDGE_CURVE('',#8052,#8146,#5905,.T.);
#10618=EDGE_CURVE('',#8147,#8145,#5906,.T.);
#10619=EDGE_CURVE('',#8148,#8147,#5137,.F.);
#10620=EDGE_CURVE('',#8149,#8148,#5907,.T.);
#10621=EDGE_CURVE('',#8150,#8149,#5138,.F.);
#10622=EDGE_CURVE('',#8150,#8146,#670,.T.);
#10623=EDGE_CURVE('',#8151,#8102,#4006,.T.);
#10624=EDGE_CURVE('',#8147,#8151,#5139,.T.);
#10625=EDGE_CURVE('',#8152,#8153,#4007,.T.);
#10626=EDGE_CURVE('',#8153,#8152,#4008,.T.);
#10627=EDGE_CURVE('',#8152,#8154,#4009,.T.);
#10628=EDGE_CURVE('',#8154,#8155,#4010,.T.);
#10629=EDGE_CURVE('',#8155,#8154,#4011,.T.);
#10630=EDGE_CURVE('',#8155,#8156,#5908,.T.);
#10631=EDGE_CURVE('',#8157,#8156,#4012,.T.);
#10632=EDGE_CURVE('',#8156,#8157,#4013,.T.);
#10633=EDGE_CURVE('',#8158,#8159,#4014,.T.);
#10634=EDGE_CURVE('',#8158,#8153,#5909,.T.);
#10635=EDGE_CURVE('',#8159,#8158,#4015,.T.);
#10636=EDGE_CURVE('',#8157,#8160,#4016,.T.);
#10637=EDGE_CURVE('',#8160,#8160,#4017,.T.);
#10638=EDGE_CURVE('',#8161,#8161,#4018,.T.);
#10639=EDGE_CURVE('',#8162,#8162,#4019,.T.);
#10640=EDGE_CURVE('',#8163,#8163,#4020,.T.);
#10641=EDGE_CURVE('',#8164,#8164,#4021,.T.);
#10642=EDGE_CURVE('',#8165,#8165,#4022,.T.);
#10643=EDGE_CURVE('',#8166,#8166,#4023,.T.);
#10644=EDGE_CURVE('',#8167,#8167,#4024,.T.);
#10645=EDGE_CURVE('',#8161,#8142,#4025,.T.);
#10646=EDGE_CURVE('',#8167,#8138,#4026,.T.);
#10647=EDGE_CURVE('',#8162,#8134,#4027,.T.);
#10648=EDGE_CURVE('',#8168,#8169,#4028,.T.);
#10649=EDGE_CURVE('',#8169,#8168,#4029,.T.);
#10650=EDGE_CURVE('',#8168,#8122,#4030,.T.);
#10651=EDGE_CURVE('',#8169,#8170,#5910,.T.);
#10652=EDGE_CURVE('',#8171,#8170,#4031,.T.);
#10653=EDGE_CURVE('',#8170,#8171,#4032,.T.);
#10654=EDGE_CURVE('',#8172,#8173,#4033,.T.);
#10655=EDGE_CURVE('',#8173,#7980,#4034,.T.);
#10656=EDGE_CURVE('',#8173,#8172,#4035,.T.);
#10657=EDGE_CURVE('',#8172,#8174,#5911,.T.);
#10658=EDGE_CURVE('',#8175,#8174,#4036,.T.);
#10659=EDGE_CURVE('',#8174,#8175,#4037,.T.);
#10660=EDGE_CURVE('',#8175,#8171,#4038,.T.);
#10661=EDGE_CURVE('',#8166,#8176,#4039,.T.);
#10662=EDGE_CURVE('',#8176,#8177,#4040,.T.);
#10663=EDGE_CURVE('',#8177,#8176,#4041,.T.);
#10664=EDGE_CURVE('',#8178,#8179,#4042,.T.);
#10665=EDGE_CURVE('',#8178,#8177,#5912,.T.);
#10666=EDGE_CURVE('',#8179,#8178,#4043,.T.);
#10667=EDGE_CURVE('',#8180,#8181,#4044,.T.);
#10668=EDGE_CURVE('',#8181,#8180,#4045,.T.);
#10669=EDGE_CURVE('',#8180,#8159,#4046,.T.);
#10670=EDGE_CURVE('',#8182,#8150,#4047,.T.);
#10671=EDGE_CURVE('',#8182,#8181,#5913,.T.);
#10672=EDGE_CURVE('',#8183,#8182,#4048,.T.);
#10673=EDGE_CURVE('',#8184,#8183,#671,.T.);
#10674=EDGE_CURVE('',#8146,#8184,#4049,.T.);
#10675=EDGE_CURVE('',#8151,#7799,#4050,.F.);
#10676=EDGE_CURVE('',#7818,#7817,#4051,.T.);
#10677=EDGE_CURVE('',#7819,#7860,#4052,.F.);
#10678=EDGE_CURVE('',#7857,#7856,#4053,.T.);
#10679=EDGE_CURVE('',#7850,#7931,#4054,.F.);
#10680=EDGE_CURVE('',#8185,#7930,#5140,.T.);
#10681=EDGE_CURVE('',#8185,#8186,#4055,.T.);
#10682=EDGE_CURVE('',#8183,#8186,#5141,.T.);
#10683=EDGE_CURVE('',#8149,#8148,#4056,.T.);
#10684=EDGE_CURVE('',#8187,#8187,#4057,.T.);
#10685=EDGE_CURVE('',#8187,#8188,#4058,.T.);
#10686=EDGE_CURVE('',#8188,#8189,#4059,.T.);
#10687=EDGE_CURVE('',#8189,#8188,#4060,.T.);
#10688=EDGE_CURVE('',#8184,#7888,#5914,.T.);
#10689=EDGE_CURVE('',#7807,#7792,#5915,.T.);
#10690=EDGE_CURVE('',#8190,#8190,#4061,.T.);
#10691=EDGE_CURVE('',#8191,#8191,#4062,.T.);
#10692=EDGE_CURVE('',#8192,#8192,#4063,.T.);
#10693=EDGE_CURVE('',#8143,#8189,#5916,.T.);
#10694=EDGE_CURVE('',#8190,#8193,#4064,.T.);
#10695=EDGE_CURVE('',#8193,#8194,#4065,.T.);
#10696=EDGE_CURVE('',#8194,#8193,#4066,.T.);
#10697=EDGE_CURVE('',#8139,#8194,#5917,.T.);
#10698=EDGE_CURVE('',#8192,#8195,#4067,.T.);
#10699=EDGE_CURVE('',#8195,#8196,#4068,.T.);
#10700=EDGE_CURVE('',#8196,#8195,#4069,.T.);
#10701=EDGE_CURVE('',#8135,#8196,#5918,.T.);
#10702=EDGE_CURVE('',#8197,#8198,#4070,.T.);
#10703=EDGE_CURVE('',#8198,#8179,#4071,.T.);
#10704=EDGE_CURVE('',#8198,#8197,#4072,.T.);
#10705=EDGE_CURVE('',#8197,#8199,#5919,.T.);
#10706=EDGE_CURVE('',#8200,#8199,#4073,.T.);
#10707=EDGE_CURVE('',#8199,#8200,#4074,.T.);
#10708=EDGE_CURVE('',#8200,#8191,#4075,.T.);
#10709=EDGE_CURVE('',#8037,#8029,#5920,.T.);
#10710=EDGE_CURVE('',#8185,#8186,#5921,.T.);
#10711=EDGE_CURVE('',#7953,#8092,#5922,.T.);
#10712=EDGE_CURVE('',#8163,#8119,#5923,.T.);
#10713=EDGE_CURVE('',#8164,#8120,#5924,.T.);
#10714=EDGE_CURVE('',#8165,#8121,#5925,.T.);
#13844=ORIENTED_EDGE('',*,*,#9955,.T.);
#13845=ORIENTED_EDGE('',*,*,#9956,.T.);
#13846=ORIENTED_EDGE('',*,*,#9957,.T.);
#13847=ORIENTED_EDGE('',*,*,#9958,.T.);
#13848=ORIENTED_EDGE('',*,*,#9959,.T.);
#13849=ORIENTED_EDGE('',*,*,#9960,.T.);
#13850=ORIENTED_EDGE('',*,*,#9957,.F.);
#13851=ORIENTED_EDGE('',*,*,#9961,.T.);
#13852=ORIENTED_EDGE('',*,*,#9962,.T.);
#13853=ORIENTED_EDGE('',*,*,#9963,.T.);
#13854=ORIENTED_EDGE('',*,*,#9964,.F.);
#13855=ORIENTED_EDGE('',*,*,#9965,.T.);
#13856=ORIENTED_EDGE('',*,*,#9966,.T.);
#13857=ORIENTED_EDGE('',*,*,#9967,.T.);
#13858=ORIENTED_EDGE('',*,*,#9968,.T.);
#13859=ORIENTED_EDGE('',*,*,#9969,.T.);
#13860=ORIENTED_EDGE('',*,*,#9968,.F.);
#13861=ORIENTED_EDGE('',*,*,#9970,.T.);
#13862=ORIENTED_EDGE('',*,*,#9962,.F.);
#13863=ORIENTED_EDGE('',*,*,#9971,.F.);
#13864=ORIENTED_EDGE('',*,*,#9972,.T.);
#13865=ORIENTED_EDGE('',*,*,#9973,.T.);
#13866=ORIENTED_EDGE('',*,*,#9974,.T.);
#13867=ORIENTED_EDGE('',*,*,#9975,.T.);
#13868=ORIENTED_EDGE('',*,*,#9976,.T.);
#13869=ORIENTED_EDGE('',*,*,#9973,.F.);
#13870=ORIENTED_EDGE('',*,*,#9977,.T.);
#13871=ORIENTED_EDGE('',*,*,#9978,.T.);
#13872=ORIENTED_EDGE('',*,*,#9979,.T.);
#13873=ORIENTED_EDGE('',*,*,#9980,.F.);
#13874=ORIENTED_EDGE('',*,*,#9981,.T.);
#13875=ORIENTED_EDGE('',*,*,#9978,.F.);
#13876=ORIENTED_EDGE('',*,*,#9982,.T.);
#13877=ORIENTED_EDGE('',*,*,#9966,.F.);
#13878=ORIENTED_EDGE('',*,*,#9961,.F.);
#13879=ORIENTED_EDGE('',*,*,#9983,.T.);
#13880=ORIENTED_EDGE('',*,*,#9984,.T.);
#13881=ORIENTED_EDGE('',*,*,#9985,.T.);
#13882=ORIENTED_EDGE('',*,*,#9956,.F.);
#13883=ORIENTED_EDGE('',*,*,#9963,.F.);
#13884=ORIENTED_EDGE('',*,*,#9986,.F.);
#13885=ORIENTED_EDGE('',*,*,#9983,.F.);
#13886=ORIENTED_EDGE('',*,*,#9970,.F.);
#13887=ORIENTED_EDGE('',*,*,#9987,.T.);
#13888=ORIENTED_EDGE('',*,*,#9988,.T.);
#13889=ORIENTED_EDGE('',*,*,#9986,.T.);
#13890=ORIENTED_EDGE('',*,*,#9967,.F.);
#13891=ORIENTED_EDGE('',*,*,#9989,.F.);
#13892=ORIENTED_EDGE('',*,*,#9990,.F.);
#13893=ORIENTED_EDGE('',*,*,#9987,.F.);
#13894=ORIENTED_EDGE('',*,*,#9982,.F.);
#13895=ORIENTED_EDGE('',*,*,#9991,.T.);
#13896=ORIENTED_EDGE('',*,*,#9992,.F.);
#13897=ORIENTED_EDGE('',*,*,#9989,.T.);
#13898=ORIENTED_EDGE('',*,*,#9981,.F.);
#13899=ORIENTED_EDGE('',*,*,#9977,.F.);
#13900=ORIENTED_EDGE('',*,*,#9993,.F.);
#13901=ORIENTED_EDGE('',*,*,#9991,.F.);
#13902=ORIENTED_EDGE('',*,*,#9959,.F.);
#13903=ORIENTED_EDGE('',*,*,#9994,.T.);
#13904=ORIENTED_EDGE('',*,*,#9971,.T.);
#13905=ORIENTED_EDGE('',*,*,#9995,.T.);
#13906=ORIENTED_EDGE('',*,*,#9972,.F.);
#13907=ORIENTED_EDGE('',*,*,#9996,.T.);
#13908=ORIENTED_EDGE('',*,*,#9997,.T.);
#13909=ORIENTED_EDGE('',*,*,#9993,.T.);
#13910=ORIENTED_EDGE('',*,*,#9988,.F.);
#13911=ORIENTED_EDGE('',*,*,#9998,.T.);
#13912=ORIENTED_EDGE('',*,*,#9984,.F.);
#13913=ORIENTED_EDGE('',*,*,#9985,.F.);
#13914=ORIENTED_EDGE('',*,*,#9999,.F.);
#13915=ORIENTED_EDGE('',*,*,#9996,.F.);
#13916=ORIENTED_EDGE('',*,*,#9994,.F.);
#13917=ORIENTED_EDGE('',*,*,#9998,.F.);
#13918=ORIENTED_EDGE('',*,*,#9990,.T.);
#13919=ORIENTED_EDGE('',*,*,#10000,.T.);
#13920=ORIENTED_EDGE('',*,*,#9999,.T.);
#13921=ORIENTED_EDGE('',*,*,#9965,.F.);
#13922=ORIENTED_EDGE('',*,*,#10001,.F.);
#13923=ORIENTED_EDGE('',*,*,#9979,.F.);
#13924=ORIENTED_EDGE('',*,*,#9969,.F.);
#13925=ORIENTED_EDGE('',*,*,#10002,.T.);
#13926=ORIENTED_EDGE('',*,*,#10003,.F.);
#13927=ORIENTED_EDGE('',*,*,#10004,.F.);
#13928=ORIENTED_EDGE('',*,*,#10005,.T.);
#13929=ORIENTED_EDGE('',*,*,#10006,.T.);
#13930=ORIENTED_EDGE('',*,*,#10007,.T.);
#13931=ORIENTED_EDGE('',*,*,#10006,.F.);
#13932=ORIENTED_EDGE('',*,*,#10008,.T.);
#13933=ORIENTED_EDGE('',*,*,#9964,.T.);
#13934=ORIENTED_EDGE('',*,*,#9955,.F.);
#13935=ORIENTED_EDGE('',*,*,#9958,.F.);
#13936=ORIENTED_EDGE('',*,*,#10009,.F.);
#13937=ORIENTED_EDGE('',*,*,#10010,.F.);
#13938=ORIENTED_EDGE('',*,*,#10011,.T.);
#13939=ORIENTED_EDGE('',*,*,#10012,.F.);
#13940=ORIENTED_EDGE('',*,*,#10007,.F.);
#13941=ORIENTED_EDGE('',*,*,#10008,.F.);
#13942=ORIENTED_EDGE('',*,*,#10013,.T.);
#13943=ORIENTED_EDGE('',*,*,#10014,.T.);
#13944=ORIENTED_EDGE('',*,*,#10001,.T.);
#13945=ORIENTED_EDGE('',*,*,#10014,.F.);
#13946=ORIENTED_EDGE('',*,*,#10015,.T.);
#13947=ORIENTED_EDGE('',*,*,#9975,.F.);
#13948=ORIENTED_EDGE('',*,*,#9980,.T.);
#13949=ORIENTED_EDGE('',*,*,#10015,.F.);
#13950=ORIENTED_EDGE('',*,*,#10016,.T.);
#13951=ORIENTED_EDGE('',*,*,#10017,.T.);
#13952=ORIENTED_EDGE('',*,*,#10018,.T.);
#13953=ORIENTED_EDGE('',*,*,#10019,.F.);
#13954=ORIENTED_EDGE('',*,*,#10020,.F.);
#13955=ORIENTED_EDGE('',*,*,#10021,.F.);
#13956=ORIENTED_EDGE('',*,*,#10016,.F.);
#13957=ORIENTED_EDGE('',*,*,#10013,.F.);
#13958=ORIENTED_EDGE('',*,*,#10005,.F.);
#13959=ORIENTED_EDGE('',*,*,#10022,.T.);
#13960=ORIENTED_EDGE('',*,*,#10023,.T.);
#13961=ORIENTED_EDGE('',*,*,#10024,.T.);
#13962=ORIENTED_EDGE('',*,*,#10025,.T.);
#13963=ORIENTED_EDGE('',*,*,#10026,.T.);
#13964=ORIENTED_EDGE('',*,*,#10024,.F.);
#13965=ORIENTED_EDGE('',*,*,#10019,.T.);
#13966=ORIENTED_EDGE('',*,*,#10004,.T.);
#13967=ORIENTED_EDGE('',*,*,#10023,.F.);
#13968=ORIENTED_EDGE('',*,*,#10027,.T.);
#13969=ORIENTED_EDGE('',*,*,#10028,.T.);
#13970=ORIENTED_EDGE('',*,*,#10029,.T.);
#13971=ORIENTED_EDGE('',*,*,#10020,.T.);
#13972=ORIENTED_EDGE('',*,*,#10022,.F.);
#13973=ORIENTED_EDGE('',*,*,#10030,.T.);
#13974=ORIENTED_EDGE('',*,*,#10031,.T.);
#13975=ORIENTED_EDGE('',*,*,#10032,.T.);
#13976=ORIENTED_EDGE('',*,*,#10025,.F.);
#13977=ORIENTED_EDGE('',*,*,#10033,.T.);
#13978=ORIENTED_EDGE('',*,*,#10034,.T.);
#13979=ORIENTED_EDGE('',*,*,#10035,.T.);
#13980=ORIENTED_EDGE('',*,*,#10036,.T.);
#13981=ORIENTED_EDGE('',*,*,#10037,.T.);
#13982=ORIENTED_EDGE('',*,*,#10002,.F.);
#13983=ORIENTED_EDGE('',*,*,#10012,.T.);
#13984=ORIENTED_EDGE('',*,*,#10038,.T.);
#13985=ORIENTED_EDGE('',*,*,#10036,.F.);
#13986=ORIENTED_EDGE('',*,*,#10039,.T.);
#13987=ORIENTED_EDGE('',*,*,#10034,.F.);
#13988=ORIENTED_EDGE('',*,*,#10035,.F.);
#13989=ORIENTED_EDGE('',*,*,#10040,.F.);
#13990=ORIENTED_EDGE('',*,*,#10041,.F.);
#13991=ORIENTED_EDGE('',*,*,#10030,.F.);
#13992=ORIENTED_EDGE('',*,*,#10039,.F.);
#13993=ORIENTED_EDGE('',*,*,#10042,.T.);
#13994=ORIENTED_EDGE('',*,*,#10043,.F.);
#13995=ORIENTED_EDGE('',*,*,#10040,.T.);
#13996=ORIENTED_EDGE('',*,*,#10038,.F.);
#13997=ORIENTED_EDGE('',*,*,#10011,.F.);
#13998=ORIENTED_EDGE('',*,*,#10044,.F.);
#13999=ORIENTED_EDGE('',*,*,#10042,.F.);
#14000=ORIENTED_EDGE('',*,*,#10000,.F.);
#14001=ORIENTED_EDGE('',*,*,#9992,.T.);
#14002=ORIENTED_EDGE('',*,*,#9997,.F.);
#14003=ORIENTED_EDGE('',*,*,#9974,.F.);
#14004=ORIENTED_EDGE('',*,*,#10045,.T.);
#14005=ORIENTED_EDGE('',*,*,#10046,.T.);
#14006=ORIENTED_EDGE('',*,*,#10047,.T.);
#14007=ORIENTED_EDGE('',*,*,#9995,.F.);
#14008=ORIENTED_EDGE('',*,*,#10047,.F.);
#14009=ORIENTED_EDGE('',*,*,#10048,.F.);
#14010=ORIENTED_EDGE('',*,*,#10049,.F.);
#14011=ORIENTED_EDGE('',*,*,#10050,.F.);
#14012=ORIENTED_EDGE('',*,*,#10051,.F.);
#14013=ORIENTED_EDGE('',*,*,#9960,.F.);
#14014=ORIENTED_EDGE('',*,*,#10051,.T.);
#14015=ORIENTED_EDGE('',*,*,#10052,.T.);
#14016=ORIENTED_EDGE('',*,*,#10053,.T.);
#14017=ORIENTED_EDGE('',*,*,#10054,.F.);
#14018=ORIENTED_EDGE('',*,*,#10009,.T.);
#14019=ORIENTED_EDGE('',*,*,#10055,.T.);
#14020=ORIENTED_EDGE('',*,*,#10044,.T.);
#14021=ORIENTED_EDGE('',*,*,#10010,.T.);
#14022=ORIENTED_EDGE('',*,*,#10054,.T.);
#14023=ORIENTED_EDGE('',*,*,#10056,.T.);
#14024=ORIENTED_EDGE('',*,*,#10057,.T.);
#14025=ORIENTED_EDGE('',*,*,#10043,.T.);
#14026=ORIENTED_EDGE('',*,*,#10055,.F.);
#14027=ORIENTED_EDGE('',*,*,#10058,.F.);
#14028=ORIENTED_EDGE('',*,*,#10041,.T.);
#14029=ORIENTED_EDGE('',*,*,#10057,.F.);
#14030=ORIENTED_EDGE('',*,*,#10059,.T.);
#14031=ORIENTED_EDGE('',*,*,#10032,.F.);
#14032=ORIENTED_EDGE('',*,*,#10060,.F.);
#14033=ORIENTED_EDGE('',*,*,#10061,.F.);
#14034=ORIENTED_EDGE('',*,*,#10062,.F.);
#14035=ORIENTED_EDGE('',*,*,#10063,.T.);
#14036=ORIENTED_EDGE('',*,*,#10027,.F.);
#14037=ORIENTED_EDGE('',*,*,#10026,.F.);
#14038=ORIENTED_EDGE('',*,*,#10003,.T.);
#14039=ORIENTED_EDGE('',*,*,#10037,.F.);
#14040=ORIENTED_EDGE('',*,*,#10033,.F.);
#14041=ORIENTED_EDGE('',*,*,#10064,.T.);
#14042=ORIENTED_EDGE('',*,*,#10065,.T.);
#14043=ORIENTED_EDGE('',*,*,#10052,.F.);
#14044=ORIENTED_EDGE('',*,*,#10050,.T.);
#14045=ORIENTED_EDGE('',*,*,#10064,.F.);
#14046=ORIENTED_EDGE('',*,*,#10066,.T.);
#14047=ORIENTED_EDGE('',*,*,#10031,.F.);
#14048=ORIENTED_EDGE('',*,*,#10058,.T.);
#14049=ORIENTED_EDGE('',*,*,#10066,.F.);
#14050=ORIENTED_EDGE('',*,*,#10049,.T.);
#14051=ORIENTED_EDGE('',*,*,#10067,.F.);
#14052=ORIENTED_EDGE('',*,*,#10068,.F.);
#14053=ORIENTED_EDGE('',*,*,#10060,.T.);
#14054=ORIENTED_EDGE('',*,*,#10056,.F.);
#14055=ORIENTED_EDGE('',*,*,#10053,.F.);
#14056=ORIENTED_EDGE('',*,*,#10065,.F.);
#14057=ORIENTED_EDGE('',*,*,#10059,.F.);
#14058=ORIENTED_EDGE('',*,*,#10069,.T.);
#14059=ORIENTED_EDGE('',*,*,#10070,.T.);
#14060=ORIENTED_EDGE('',*,*,#10071,.T.);
#14061=ORIENTED_EDGE('',*,*,#10072,.T.);
#14062=ORIENTED_EDGE('',*,*,#10073,.T.);
#14063=ORIENTED_EDGE('',*,*,#10074,.T.);
#14064=ORIENTED_EDGE('',*,*,#10075,.T.);
#14065=ORIENTED_EDGE('',*,*,#10076,.T.);
#14066=ORIENTED_EDGE('',*,*,#10077,.F.);
#14067=ORIENTED_EDGE('',*,*,#10078,.T.);
#14068=ORIENTED_EDGE('',*,*,#10075,.F.);
#14069=ORIENTED_EDGE('',*,*,#10079,.T.);
#14070=ORIENTED_EDGE('',*,*,#10070,.F.);
#14071=ORIENTED_EDGE('',*,*,#10080,.F.);
#14072=ORIENTED_EDGE('',*,*,#10081,.F.);
#14073=ORIENTED_EDGE('',*,*,#10082,.F.);
#14074=ORIENTED_EDGE('',*,*,#10076,.F.);
#14075=ORIENTED_EDGE('',*,*,#10083,.F.);
#14076=ORIENTED_EDGE('',*,*,#10084,.F.);
#14077=ORIENTED_EDGE('',*,*,#10085,.F.);
#14078=ORIENTED_EDGE('',*,*,#10086,.T.);
#14079=ORIENTED_EDGE('',*,*,#10085,.T.);
#14080=ORIENTED_EDGE('',*,*,#10087,.T.);
#14081=ORIENTED_EDGE('',*,*,#10088,.T.);
#14082=ORIENTED_EDGE('',*,*,#10086,.F.);
#14083=ORIENTED_EDGE('',*,*,#10089,.T.);
#14084=ORIENTED_EDGE('',*,*,#10069,.F.);
#14085=ORIENTED_EDGE('',*,*,#10073,.F.);
#14086=ORIENTED_EDGE('',*,*,#10090,.T.);
#14087=ORIENTED_EDGE('',*,*,#10091,.T.);
#14088=ORIENTED_EDGE('',*,*,#10092,.T.);
#14089=ORIENTED_EDGE('',*,*,#10084,.T.);
#14090=ORIENTED_EDGE('',*,*,#10092,.F.);
#14091=ORIENTED_EDGE('',*,*,#10093,.T.);
#14092=ORIENTED_EDGE('',*,*,#10087,.F.);
#14093=ORIENTED_EDGE('',*,*,#10078,.F.);
#14094=ORIENTED_EDGE('',*,*,#10094,.T.);
#14095=ORIENTED_EDGE('',*,*,#10095,.T.);
#14096=ORIENTED_EDGE('',*,*,#10083,.T.);
#14097=ORIENTED_EDGE('',*,*,#10095,.F.);
#14098=ORIENTED_EDGE('',*,*,#10096,.T.);
#14099=ORIENTED_EDGE('',*,*,#10090,.F.);
#14100=ORIENTED_EDGE('',*,*,#10089,.F.);
#14101=ORIENTED_EDGE('',*,*,#10097,.T.);
#14102=ORIENTED_EDGE('',*,*,#10098,.T.);
#14103=ORIENTED_EDGE('',*,*,#10080,.T.);
#14104=ORIENTED_EDGE('',*,*,#10088,.F.);
#14105=ORIENTED_EDGE('',*,*,#10099,.F.);
#14106=ORIENTED_EDGE('',*,*,#10100,.F.);
#14107=ORIENTED_EDGE('',*,*,#10097,.F.);
#14108=ORIENTED_EDGE('',*,*,#10093,.F.);
#14109=ORIENTED_EDGE('',*,*,#10101,.T.);
#14110=ORIENTED_EDGE('',*,*,#10102,.F.);
#14111=ORIENTED_EDGE('',*,*,#10099,.T.);
#14112=ORIENTED_EDGE('',*,*,#10091,.F.);
#14113=ORIENTED_EDGE('',*,*,#10103,.F.);
#14114=ORIENTED_EDGE('',*,*,#10104,.F.);
#14115=ORIENTED_EDGE('',*,*,#10101,.F.);
#14116=ORIENTED_EDGE('',*,*,#10096,.F.);
#14117=ORIENTED_EDGE('',*,*,#10105,.T.);
#14118=ORIENTED_EDGE('',*,*,#10106,.F.);
#14119=ORIENTED_EDGE('',*,*,#10103,.T.);
#14120=ORIENTED_EDGE('',*,*,#10094,.F.);
#14121=ORIENTED_EDGE('',*,*,#10107,.F.);
#14122=ORIENTED_EDGE('',*,*,#10108,.F.);
#14123=ORIENTED_EDGE('',*,*,#10105,.F.);
#14124=ORIENTED_EDGE('',*,*,#10077,.T.);
#14125=ORIENTED_EDGE('',*,*,#10109,.T.);
#14126=ORIENTED_EDGE('',*,*,#10110,.T.);
#14127=ORIENTED_EDGE('',*,*,#10107,.T.);
#14128=ORIENTED_EDGE('',*,*,#10111,.T.);
#14129=ORIENTED_EDGE('',*,*,#10112,.T.);
#14130=ORIENTED_EDGE('',*,*,#10113,.T.);
#14131=ORIENTED_EDGE('',*,*,#10114,.T.);
#14132=ORIENTED_EDGE('',*,*,#10115,.F.);
#14133=ORIENTED_EDGE('',*,*,#10116,.T.);
#14134=ORIENTED_EDGE('',*,*,#10117,.T.);
#14135=ORIENTED_EDGE('',*,*,#10118,.T.);
#14136=ORIENTED_EDGE('',*,*,#10119,.F.);
#14137=ORIENTED_EDGE('',*,*,#10117,.F.);
#14138=ORIENTED_EDGE('',*,*,#10120,.T.);
#14139=ORIENTED_EDGE('',*,*,#10111,.F.);
#14140=ORIENTED_EDGE('',*,*,#10112,.F.);
#14141=ORIENTED_EDGE('',*,*,#10121,.F.);
#14142=ORIENTED_EDGE('',*,*,#10122,.F.);
#14143=ORIENTED_EDGE('',*,*,#10123,.F.);
#14144=ORIENTED_EDGE('',*,*,#10120,.F.);
#14145=ORIENTED_EDGE('',*,*,#10124,.T.);
#14146=ORIENTED_EDGE('',*,*,#10125,.T.);
#14147=ORIENTED_EDGE('',*,*,#10121,.T.);
#14148=ORIENTED_EDGE('',*,*,#10116,.F.);
#14149=ORIENTED_EDGE('',*,*,#10126,.F.);
#14150=ORIENTED_EDGE('',*,*,#10127,.F.);
#14151=ORIENTED_EDGE('',*,*,#10128,.T.);
#14152=ORIENTED_EDGE('',*,*,#10129,.F.);
#14153=ORIENTED_EDGE('',*,*,#10124,.F.);
#14154=ORIENTED_EDGE('',*,*,#10125,.F.);
#14155=ORIENTED_EDGE('',*,*,#10130,.T.);
#14156=ORIENTED_EDGE('',*,*,#10131,.T.);
#14157=ORIENTED_EDGE('',*,*,#10072,.F.);
#14158=ORIENTED_EDGE('',*,*,#10132,.F.);
#14159=ORIENTED_EDGE('',*,*,#10118,.F.);
#14160=ORIENTED_EDGE('',*,*,#10114,.F.);
#14161=ORIENTED_EDGE('',*,*,#10133,.F.);
#14162=ORIENTED_EDGE('',*,*,#10074,.F.);
#14163=ORIENTED_EDGE('',*,*,#10130,.F.);
#14164=ORIENTED_EDGE('',*,*,#10129,.T.);
#14165=ORIENTED_EDGE('',*,*,#10134,.T.);
#14166=ORIENTED_EDGE('',*,*,#10135,.T.);
#14167=ORIENTED_EDGE('',*,*,#10136,.T.);
#14168=ORIENTED_EDGE('',*,*,#10131,.F.);
#14169=ORIENTED_EDGE('',*,*,#10137,.T.);
#14170=ORIENTED_EDGE('',*,*,#10138,.T.);
#14171=ORIENTED_EDGE('',*,*,#10122,.T.);
#14172=ORIENTED_EDGE('',*,*,#10139,.T.);
#14173=ORIENTED_EDGE('',*,*,#10108,.T.);
#14174=ORIENTED_EDGE('',*,*,#10140,.F.);
#14175=ORIENTED_EDGE('',*,*,#10141,.T.);
#14176=ORIENTED_EDGE('',*,*,#10142,.T.);
#14177=ORIENTED_EDGE('',*,*,#10104,.T.);
#14178=ORIENTED_EDGE('',*,*,#10143,.T.);
#14179=ORIENTED_EDGE('',*,*,#10144,.T.);
#14180=ORIENTED_EDGE('',*,*,#10145,.T.);
#14181=ORIENTED_EDGE('',*,*,#10102,.T.);
#14182=ORIENTED_EDGE('',*,*,#10142,.F.);
#14183=ORIENTED_EDGE('',*,*,#10146,.T.);
#14184=ORIENTED_EDGE('',*,*,#10100,.T.);
#14185=ORIENTED_EDGE('',*,*,#10145,.F.);
#14186=ORIENTED_EDGE('',*,*,#10147,.T.);
#14187=ORIENTED_EDGE('',*,*,#10143,.F.);
#14188=ORIENTED_EDGE('',*,*,#10106,.T.);
#14189=ORIENTED_EDGE('',*,*,#10139,.F.);
#14190=ORIENTED_EDGE('',*,*,#10147,.F.);
#14191=ORIENTED_EDGE('',*,*,#10144,.F.);
#14192=ORIENTED_EDGE('',*,*,#10141,.F.);
#14193=ORIENTED_EDGE('',*,*,#10148,.F.);
#14194=ORIENTED_EDGE('',*,*,#10109,.F.);
#14195=ORIENTED_EDGE('',*,*,#10149,.F.);
#14196=ORIENTED_EDGE('',*,*,#10123,.T.);
#14197=ORIENTED_EDGE('',*,*,#10150,.F.);
#14198=ORIENTED_EDGE('',*,*,#10079,.F.);
#14199=ORIENTED_EDGE('',*,*,#10133,.T.);
#14200=ORIENTED_EDGE('',*,*,#10113,.F.);
#14201=ORIENTED_EDGE('',*,*,#10149,.T.);
#14202=ORIENTED_EDGE('',*,*,#10151,.T.);
#14203=ORIENTED_EDGE('',*,*,#10150,.T.);
#14204=ORIENTED_EDGE('',*,*,#10138,.F.);
#14205=ORIENTED_EDGE('',*,*,#10152,.T.);
#14206=ORIENTED_EDGE('',*,*,#10151,.F.);
#14207=ORIENTED_EDGE('',*,*,#10153,.T.);
#14208=ORIENTED_EDGE('',*,*,#10140,.T.);
#14209=ORIENTED_EDGE('',*,*,#10110,.F.);
#14210=ORIENTED_EDGE('',*,*,#10153,.F.);
#14211=ORIENTED_EDGE('',*,*,#10154,.T.);
#14212=ORIENTED_EDGE('',*,*,#10155,.T.);
#14213=ORIENTED_EDGE('',*,*,#10148,.T.);
#14214=ORIENTED_EDGE('',*,*,#10136,.F.);
#14215=ORIENTED_EDGE('',*,*,#10156,.F.);
#14216=ORIENTED_EDGE('',*,*,#10157,.F.);
#14217=ORIENTED_EDGE('',*,*,#10154,.F.);
#14218=ORIENTED_EDGE('',*,*,#10152,.F.);
#14219=ORIENTED_EDGE('',*,*,#10137,.F.);
#14220=ORIENTED_EDGE('',*,*,#10155,.F.);
#14221=ORIENTED_EDGE('',*,*,#10158,.T.);
#14222=ORIENTED_EDGE('',*,*,#10098,.F.);
#14223=ORIENTED_EDGE('',*,*,#10146,.F.);
#14224=ORIENTED_EDGE('',*,*,#10158,.F.);
#14225=ORIENTED_EDGE('',*,*,#10157,.T.);
#14226=ORIENTED_EDGE('',*,*,#10159,.T.);
#14227=ORIENTED_EDGE('',*,*,#10081,.T.);
#14228=ORIENTED_EDGE('',*,*,#10160,.F.);
#14229=ORIENTED_EDGE('',*,*,#10161,.T.);
#14230=ORIENTED_EDGE('',*,*,#10162,.T.);
#14231=ORIENTED_EDGE('',*,*,#10163,.T.);
#14232=ORIENTED_EDGE('',*,*,#10164,.F.);
#14233=ORIENTED_EDGE('',*,*,#10165,.T.);
#14234=ORIENTED_EDGE('',*,*,#10166,.T.);
#14235=ORIENTED_EDGE('',*,*,#10167,.T.);
#14236=ORIENTED_EDGE('',*,*,#10168,.T.);
#14237=ORIENTED_EDGE('',*,*,#10169,.T.);
#14238=ORIENTED_EDGE('',*,*,#10167,.F.);
#14239=ORIENTED_EDGE('',*,*,#10170,.T.);
#14240=ORIENTED_EDGE('',*,*,#10162,.F.);
#14241=ORIENTED_EDGE('',*,*,#10163,.F.);
#14242=ORIENTED_EDGE('',*,*,#10171,.F.);
#14243=ORIENTED_EDGE('',*,*,#10172,.F.);
#14244=ORIENTED_EDGE('',*,*,#10173,.F.);
#14245=ORIENTED_EDGE('',*,*,#10170,.F.);
#14246=ORIENTED_EDGE('',*,*,#10174,.T.);
#14247=ORIENTED_EDGE('',*,*,#10175,.F.);
#14248=ORIENTED_EDGE('',*,*,#10176,.F.);
#14249=ORIENTED_EDGE('',*,*,#10171,.T.);
#14250=ORIENTED_EDGE('',*,*,#10166,.F.);
#14251=ORIENTED_EDGE('',*,*,#10177,.F.);
#14252=ORIENTED_EDGE('',*,*,#10178,.F.);
#14253=ORIENTED_EDGE('',*,*,#10174,.F.);
#14254=ORIENTED_EDGE('',*,*,#10165,.F.);
#14255=ORIENTED_EDGE('',*,*,#10179,.F.);
#14256=ORIENTED_EDGE('',*,*,#10180,.T.);
#14257=ORIENTED_EDGE('',*,*,#10181,.T.);
#14258=ORIENTED_EDGE('',*,*,#10177,.T.);
#14259=ORIENTED_EDGE('',*,*,#10169,.F.);
#14260=ORIENTED_EDGE('',*,*,#10182,.T.);
#14261=ORIENTED_EDGE('',*,*,#10183,.T.);
#14262=ORIENTED_EDGE('',*,*,#10184,.F.);
#14263=ORIENTED_EDGE('',*,*,#10185,.T.);
#14264=ORIENTED_EDGE('',*,*,#10179,.T.);
#14265=ORIENTED_EDGE('',*,*,#10186,.T.);
#14266=ORIENTED_EDGE('',*,*,#10187,.T.);
#14267=ORIENTED_EDGE('',*,*,#10188,.T.);
#14268=ORIENTED_EDGE('',*,*,#10189,.T.);
#14269=ORIENTED_EDGE('',*,*,#10190,.F.);
#14270=ORIENTED_EDGE('',*,*,#10191,.T.);
#14271=ORIENTED_EDGE('',*,*,#10188,.F.);
#14272=ORIENTED_EDGE('',*,*,#10192,.T.);
#14273=ORIENTED_EDGE('',*,*,#10193,.T.);
#14274=ORIENTED_EDGE('',*,*,#10194,.T.);
#14275=ORIENTED_EDGE('',*,*,#10186,.F.);
#14276=ORIENTED_EDGE('',*,*,#10195,.T.);
#14277=ORIENTED_EDGE('',*,*,#10194,.F.);
#14278=ORIENTED_EDGE('',*,*,#10196,.T.);
#14279=ORIENTED_EDGE('',*,*,#10197,.T.);
#14280=ORIENTED_EDGE('',*,*,#10198,.T.);
#14281=ORIENTED_EDGE('',*,*,#10193,.F.);
#14282=ORIENTED_EDGE('',*,*,#10199,.T.);
#14283=ORIENTED_EDGE('',*,*,#10200,.F.);
#14284=ORIENTED_EDGE('',*,*,#10201,.T.);
#14285=ORIENTED_EDGE('',*,*,#10195,.F.);
#14286=ORIENTED_EDGE('',*,*,#10202,.T.);
#14287=ORIENTED_EDGE('',*,*,#10203,.T.);
#14288=ORIENTED_EDGE('',*,*,#10204,.T.);
#14289=ORIENTED_EDGE('',*,*,#10189,.F.);
#14290=ORIENTED_EDGE('',*,*,#10205,.F.);
#14291=ORIENTED_EDGE('',*,*,#10206,.F.);
#14292=ORIENTED_EDGE('',*,*,#10202,.F.);
#14293=ORIENTED_EDGE('',*,*,#10191,.F.);
#14294=ORIENTED_EDGE('',*,*,#10207,.T.);
#14295=ORIENTED_EDGE('',*,*,#10208,.T.);
#14296=ORIENTED_EDGE('',*,*,#10205,.T.);
#14297=ORIENTED_EDGE('',*,*,#10209,.T.);
#14298=ORIENTED_EDGE('',*,*,#10210,.T.);
#14299=ORIENTED_EDGE('',*,*,#10211,.T.);
#14300=ORIENTED_EDGE('',*,*,#10212,.T.);
#14301=ORIENTED_EDGE('',*,*,#10213,.T.);
#14302=ORIENTED_EDGE('',*,*,#10214,.T.);
#14303=ORIENTED_EDGE('',*,*,#10209,.F.);
#14304=ORIENTED_EDGE('',*,*,#10211,.F.);
#14305=ORIENTED_EDGE('',*,*,#10215,.T.);
#14306=ORIENTED_EDGE('',*,*,#10208,.F.);
#14307=ORIENTED_EDGE('',*,*,#10216,.T.);
#14308=ORIENTED_EDGE('',*,*,#10217,.T.);
#14309=ORIENTED_EDGE('',*,*,#10213,.F.);
#14310=ORIENTED_EDGE('',*,*,#10218,.T.);
#14311=ORIENTED_EDGE('',*,*,#10219,.T.);
#14312=ORIENTED_EDGE('',*,*,#10215,.F.);
#14313=ORIENTED_EDGE('',*,*,#10220,.T.);
#14314=ORIENTED_EDGE('',*,*,#10221,.T.);
#14315=ORIENTED_EDGE('',*,*,#10206,.T.);
#14316=ORIENTED_EDGE('',*,*,#10210,.F.);
#14317=ORIENTED_EDGE('',*,*,#10222,.F.);
#14318=ORIENTED_EDGE('',*,*,#10223,.F.);
#14319=ORIENTED_EDGE('',*,*,#10220,.F.);
#14320=ORIENTED_EDGE('',*,*,#10214,.F.);
#14321=ORIENTED_EDGE('',*,*,#10224,.T.);
#14322=ORIENTED_EDGE('',*,*,#10225,.F.);
#14323=ORIENTED_EDGE('',*,*,#10222,.T.);
#14324=ORIENTED_EDGE('',*,*,#10217,.F.);
#14325=ORIENTED_EDGE('',*,*,#10226,.F.);
#14326=ORIENTED_EDGE('',*,*,#10227,.F.);
#14327=ORIENTED_EDGE('',*,*,#10224,.F.);
#14328=ORIENTED_EDGE('',*,*,#10216,.F.);
#14329=ORIENTED_EDGE('',*,*,#10228,.F.);
#14330=ORIENTED_EDGE('',*,*,#10229,.F.);
#14331=ORIENTED_EDGE('',*,*,#10190,.T.);
#14332=ORIENTED_EDGE('',*,*,#10230,.T.);
#14333=ORIENTED_EDGE('',*,*,#10228,.T.);
#14334=ORIENTED_EDGE('',*,*,#10219,.F.);
#14335=ORIENTED_EDGE('',*,*,#10231,.T.);
#14336=ORIENTED_EDGE('',*,*,#10207,.F.);
#14337=ORIENTED_EDGE('',*,*,#10231,.F.);
#14338=ORIENTED_EDGE('',*,*,#10218,.F.);
#14339=ORIENTED_EDGE('',*,*,#10212,.F.);
#14340=ORIENTED_EDGE('',*,*,#10192,.F.);
#14341=ORIENTED_EDGE('',*,*,#10232,.T.);
#14342=ORIENTED_EDGE('',*,*,#10233,.T.);
#14343=ORIENTED_EDGE('',*,*,#10234,.T.);
#14344=ORIENTED_EDGE('',*,*,#10187,.F.);
#14345=ORIENTED_EDGE('',*,*,#10198,.F.);
#14346=ORIENTED_EDGE('',*,*,#10235,.F.);
#14347=ORIENTED_EDGE('',*,*,#10232,.F.);
#14348=ORIENTED_EDGE('',*,*,#10236,.T.);
#14349=ORIENTED_EDGE('',*,*,#10237,.T.);
#14350=ORIENTED_EDGE('',*,*,#10238,.T.);
#14351=ORIENTED_EDGE('',*,*,#10160,.T.);
#14352=ORIENTED_EDGE('',*,*,#10239,.T.);
#14353=ORIENTED_EDGE('',*,*,#10229,.T.);
#14354=ORIENTED_EDGE('',*,*,#10236,.F.);
#14355=ORIENTED_EDGE('',*,*,#10240,.T.);
#14356=ORIENTED_EDGE('',*,*,#10240,.F.);
#14357=ORIENTED_EDGE('',*,*,#10241,.T.);
#14358=ORIENTED_EDGE('',*,*,#10242,.F.);
#14359=ORIENTED_EDGE('',*,*,#10226,.T.);
#14360=ORIENTED_EDGE('',*,*,#10239,.F.);
#14361=ORIENTED_EDGE('',*,*,#10164,.T.);
#14362=ORIENTED_EDGE('',*,*,#10173,.T.);
#14363=ORIENTED_EDGE('',*,*,#10243,.F.);
#14364=ORIENTED_EDGE('',*,*,#10244,.F.);
#14365=ORIENTED_EDGE('',*,*,#10241,.F.);
#14366=ORIENTED_EDGE('',*,*,#10230,.F.);
#14367=ORIENTED_EDGE('',*,*,#10234,.F.);
#14368=ORIENTED_EDGE('',*,*,#10245,.F.);
#14369=ORIENTED_EDGE('',*,*,#10183,.F.);
#14370=ORIENTED_EDGE('',*,*,#10246,.F.);
#14371=ORIENTED_EDGE('',*,*,#10237,.F.);
#14372=ORIENTED_EDGE('',*,*,#10161,.F.);
#14373=ORIENTED_EDGE('',*,*,#10238,.F.);
#14374=ORIENTED_EDGE('',*,*,#10246,.T.);
#14375=ORIENTED_EDGE('',*,*,#10182,.F.);
#14376=ORIENTED_EDGE('',*,*,#10168,.F.);
#14377=ORIENTED_EDGE('',*,*,#10247,.T.);
#14378=ORIENTED_EDGE('',*,*,#10248,.T.);
#14379=ORIENTED_EDGE('',*,*,#10249,.T.);
#14380=ORIENTED_EDGE('',*,*,#10250,.T.);
#14381=ORIENTED_EDGE('',*,*,#10251,.F.);
#14382=ORIENTED_EDGE('',*,*,#10248,.F.);
#14383=ORIENTED_EDGE('',*,*,#10252,.F.);
#14384=ORIENTED_EDGE('',*,*,#10253,.F.);
#14385=ORIENTED_EDGE('',*,*,#10196,.F.);
#14386=ORIENTED_EDGE('',*,*,#10201,.F.);
#14387=ORIENTED_EDGE('',*,*,#10247,.F.);
#14388=ORIENTED_EDGE('',*,*,#10254,.T.);
#14389=ORIENTED_EDGE('',*,*,#10255,.T.);
#14390=ORIENTED_EDGE('',*,*,#10175,.T.);
#14391=ORIENTED_EDGE('',*,*,#10178,.T.);
#14392=ORIENTED_EDGE('',*,*,#10256,.F.);
#14393=ORIENTED_EDGE('',*,*,#10256,.T.);
#14394=ORIENTED_EDGE('',*,*,#10181,.F.);
#14395=ORIENTED_EDGE('',*,*,#10257,.T.);
#14396=ORIENTED_EDGE('',*,*,#10255,.F.);
#14397=ORIENTED_EDGE('',*,*,#10258,.T.);
#14398=ORIENTED_EDGE('',*,*,#10259,.T.);
#14399=ORIENTED_EDGE('',*,*,#10243,.T.);
#14400=ORIENTED_EDGE('',*,*,#10172,.T.);
#14401=ORIENTED_EDGE('',*,*,#10176,.T.);
#14402=ORIENTED_EDGE('',*,*,#10221,.F.);
#14403=ORIENTED_EDGE('',*,*,#10260,.T.);
#14404=ORIENTED_EDGE('',*,*,#10203,.F.);
#14405=ORIENTED_EDGE('',*,*,#10257,.F.);
#14406=ORIENTED_EDGE('',*,*,#10261,.T.);
#14407=ORIENTED_EDGE('',*,*,#10262,.T.);
#14408=ORIENTED_EDGE('',*,*,#10263,.T.);
#14409=ORIENTED_EDGE('',*,*,#10252,.T.);
#14410=ORIENTED_EDGE('',*,*,#10250,.F.);
#14411=ORIENTED_EDGE('',*,*,#10264,.F.);
#14412=ORIENTED_EDGE('',*,*,#10258,.F.);
#14413=ORIENTED_EDGE('',*,*,#10254,.F.);
#14414=ORIENTED_EDGE('',*,*,#10265,.T.);
#14415=ORIENTED_EDGE('',*,*,#10227,.T.);
#14416=ORIENTED_EDGE('',*,*,#10266,.T.);
#14417=ORIENTED_EDGE('',*,*,#10267,.T.);
#14418=ORIENTED_EDGE('',*,*,#10268,.T.);
#14419=ORIENTED_EDGE('',*,*,#10200,.T.);
#14420=ORIENTED_EDGE('',*,*,#10266,.F.);
#14421=ORIENTED_EDGE('',*,*,#10242,.T.);
#14422=ORIENTED_EDGE('',*,*,#10264,.T.);
#14423=ORIENTED_EDGE('',*,*,#10249,.F.);
#14424=ORIENTED_EDGE('',*,*,#10251,.T.);
#14425=ORIENTED_EDGE('',*,*,#10268,.F.);
#14426=ORIENTED_EDGE('',*,*,#10244,.T.);
#14427=ORIENTED_EDGE('',*,*,#10259,.F.);
#14428=ORIENTED_EDGE('',*,*,#10260,.F.);
#14429=ORIENTED_EDGE('',*,*,#10223,.T.);
#14430=ORIENTED_EDGE('',*,*,#10269,.T.);
#14431=ORIENTED_EDGE('',*,*,#10270,.T.);
#14432=ORIENTED_EDGE('',*,*,#10269,.F.);
#14433=ORIENTED_EDGE('',*,*,#10225,.T.);
#14434=ORIENTED_EDGE('',*,*,#10265,.F.);
#14435=ORIENTED_EDGE('',*,*,#10204,.F.);
#14436=ORIENTED_EDGE('',*,*,#10270,.F.);
#14437=ORIENTED_EDGE('',*,*,#10267,.F.);
#14438=ORIENTED_EDGE('',*,*,#10199,.F.);
#14439=ORIENTED_EDGE('',*,*,#10271,.T.);
#14440=ORIENTED_EDGE('',*,*,#10272,.T.);
#14441=ORIENTED_EDGE('',*,*,#10273,.T.);
#14442=ORIENTED_EDGE('',*,*,#10272,.F.);
#14443=ORIENTED_EDGE('',*,*,#10274,.T.);
#14444=ORIENTED_EDGE('',*,*,#10271,.F.);
#14445=ORIENTED_EDGE('',*,*,#10275,.T.);
#14446=ORIENTED_EDGE('',*,*,#10276,.F.);
#14447=ORIENTED_EDGE('',*,*,#10277,.F.);
#14448=ORIENTED_EDGE('',*,*,#10278,.T.);
#14449=ORIENTED_EDGE('',*,*,#10279,.F.);
#14450=ORIENTED_EDGE('',*,*,#10280,.F.);
#14451=ORIENTED_EDGE('',*,*,#10281,.F.);
#14452=ORIENTED_EDGE('',*,*,#10282,.T.);
#14453=ORIENTED_EDGE('',*,*,#10283,.F.);
#14454=ORIENTED_EDGE('',*,*,#10284,.F.);
#14455=ORIENTED_EDGE('',*,*,#10285,.F.);
#14456=ORIENTED_EDGE('',*,*,#10286,.T.);
#14457=ORIENTED_EDGE('',*,*,#10287,.F.);
#14458=ORIENTED_EDGE('',*,*,#10288,.F.);
#14459=ORIENTED_EDGE('',*,*,#10289,.F.);
#14460=ORIENTED_EDGE('',*,*,#10290,.T.);
#14461=ORIENTED_EDGE('',*,*,#10291,.F.);
#14462=ORIENTED_EDGE('',*,*,#10292,.F.);
#14463=ORIENTED_EDGE('',*,*,#10275,.F.);
#14464=ORIENTED_EDGE('',*,*,#10274,.F.);
#14465=ORIENTED_EDGE('',*,*,#10273,.F.);
#14466=ORIENTED_EDGE('',*,*,#10293,.F.);
#14467=ORIENTED_EDGE('',*,*,#10294,.T.);
#14468=ORIENTED_EDGE('',*,*,#10295,.T.);
#14469=ORIENTED_EDGE('',*,*,#10296,.T.);
#14470=ORIENTED_EDGE('',*,*,#10297,.T.);
#14471=ORIENTED_EDGE('',*,*,#10298,.T.);
#14472=ORIENTED_EDGE('',*,*,#10299,.T.);
#14473=ORIENTED_EDGE('',*,*,#10300,.T.);
#14474=ORIENTED_EDGE('',*,*,#10296,.F.);
#14475=ORIENTED_EDGE('',*,*,#10301,.T.);
#14476=ORIENTED_EDGE('',*,*,#10302,.T.);
#14477=ORIENTED_EDGE('',*,*,#10303,.T.);
#14478=ORIENTED_EDGE('',*,*,#10299,.F.);
#14479=ORIENTED_EDGE('',*,*,#10304,.T.);
#14480=ORIENTED_EDGE('',*,*,#10305,.T.);
#14481=ORIENTED_EDGE('',*,*,#10306,.T.);
#14482=ORIENTED_EDGE('',*,*,#10302,.F.);
#14483=ORIENTED_EDGE('',*,*,#10307,.T.);
#14484=ORIENTED_EDGE('',*,*,#10308,.T.);
#14485=ORIENTED_EDGE('',*,*,#10309,.F.);
#14486=ORIENTED_EDGE('',*,*,#10309,.T.);
#14487=ORIENTED_EDGE('',*,*,#10310,.T.);
#14488=ORIENTED_EDGE('',*,*,#10311,.T.);
#14489=ORIENTED_EDGE('',*,*,#10307,.F.);
#14490=ORIENTED_EDGE('',*,*,#10312,.T.);
#14491=ORIENTED_EDGE('',*,*,#10305,.F.);
#14492=ORIENTED_EDGE('',*,*,#10313,.T.);
#14493=ORIENTED_EDGE('',*,*,#10297,.F.);
#14494=ORIENTED_EDGE('',*,*,#10300,.F.);
#14495=ORIENTED_EDGE('',*,*,#10303,.F.);
#14496=ORIENTED_EDGE('',*,*,#10314,.F.);
#14497=ORIENTED_EDGE('',*,*,#10315,.F.);
#14498=ORIENTED_EDGE('',*,*,#10316,.F.);
#14499=ORIENTED_EDGE('',*,*,#10317,.F.);
#14500=ORIENTED_EDGE('',*,*,#10318,.F.);
#14501=ORIENTED_EDGE('',*,*,#10319,.F.);
#14502=ORIENTED_EDGE('',*,*,#10320,.F.);
#14503=ORIENTED_EDGE('',*,*,#10321,.F.);
#14504=ORIENTED_EDGE('',*,*,#10322,.F.);
#14505=ORIENTED_EDGE('',*,*,#10323,.F.);
#14506=ORIENTED_EDGE('',*,*,#10324,.F.);
#14507=ORIENTED_EDGE('',*,*,#10325,.F.);
#14508=ORIENTED_EDGE('',*,*,#10326,.F.);
#14509=ORIENTED_EDGE('',*,*,#10327,.F.);
#14510=ORIENTED_EDGE('',*,*,#10306,.F.);
#14511=ORIENTED_EDGE('',*,*,#10328,.T.);
#14512=ORIENTED_EDGE('',*,*,#10329,.T.);
#14513=ORIENTED_EDGE('',*,*,#10314,.T.);
#14514=ORIENTED_EDGE('',*,*,#10312,.F.);
#14515=ORIENTED_EDGE('',*,*,#10330,.F.);
#14516=ORIENTED_EDGE('',*,*,#10331,.F.);
#14517=ORIENTED_EDGE('',*,*,#10328,.F.);
#14518=ORIENTED_EDGE('',*,*,#10311,.F.);
#14519=ORIENTED_EDGE('',*,*,#10284,.T.);
#14520=ORIENTED_EDGE('',*,*,#10332,.T.);
#14521=ORIENTED_EDGE('',*,*,#10330,.T.);
#14522=ORIENTED_EDGE('',*,*,#10308,.F.);
#14523=ORIENTED_EDGE('',*,*,#10333,.T.);
#14524=ORIENTED_EDGE('',*,*,#10334,.F.);
#14525=ORIENTED_EDGE('',*,*,#10335,.F.);
#14526=ORIENTED_EDGE('',*,*,#10285,.T.);
#14527=ORIENTED_EDGE('',*,*,#10310,.F.);
#14528=ORIENTED_EDGE('',*,*,#10336,.T.);
#14529=ORIENTED_EDGE('',*,*,#10337,.T.);
#14530=ORIENTED_EDGE('',*,*,#10338,.T.);
#14531=ORIENTED_EDGE('',*,*,#10323,.T.);
#14532=ORIENTED_EDGE('',*,*,#10339,.T.);
#14533=ORIENTED_EDGE('',*,*,#10340,.T.);
#14534=ORIENTED_EDGE('',*,*,#10324,.T.);
#14535=ORIENTED_EDGE('',*,*,#10338,.F.);
#14536=ORIENTED_EDGE('',*,*,#10341,.T.);
#14537=ORIENTED_EDGE('',*,*,#10342,.T.);
#14538=ORIENTED_EDGE('',*,*,#10325,.T.);
#14539=ORIENTED_EDGE('',*,*,#10340,.F.);
#14540=ORIENTED_EDGE('',*,*,#10343,.T.);
#14541=ORIENTED_EDGE('',*,*,#10344,.T.);
#14542=ORIENTED_EDGE('',*,*,#10339,.F.);
#14543=ORIENTED_EDGE('',*,*,#10322,.T.);
#14544=ORIENTED_EDGE('',*,*,#10345,.T.);
#14545=ORIENTED_EDGE('',*,*,#10346,.T.);
#14546=ORIENTED_EDGE('',*,*,#10298,.F.);
#14547=ORIENTED_EDGE('',*,*,#10326,.T.);
#14548=ORIENTED_EDGE('',*,*,#10342,.F.);
#14549=ORIENTED_EDGE('',*,*,#10347,.T.);
#14550=ORIENTED_EDGE('',*,*,#10348,.T.);
#14551=ORIENTED_EDGE('',*,*,#10295,.F.);
#14552=ORIENTED_EDGE('',*,*,#10349,.F.);
#14553=ORIENTED_EDGE('',*,*,#10350,.F.);
#14554=ORIENTED_EDGE('',*,*,#10351,.F.);
#14555=ORIENTED_EDGE('',*,*,#10352,.F.);
#14556=ORIENTED_EDGE('',*,*,#10353,.T.);
#14557=ORIENTED_EDGE('',*,*,#10354,.F.);
#14558=ORIENTED_EDGE('',*,*,#10294,.F.);
#14559=ORIENTED_EDGE('',*,*,#10348,.F.);
#14560=ORIENTED_EDGE('',*,*,#10355,.F.);
#14561=ORIENTED_EDGE('',*,*,#10356,.F.);
#14562=ORIENTED_EDGE('',*,*,#10349,.T.);
#14563=ORIENTED_EDGE('',*,*,#10344,.F.);
#14564=ORIENTED_EDGE('',*,*,#10357,.T.);
#14565=ORIENTED_EDGE('',*,*,#10358,.F.);
#14566=ORIENTED_EDGE('',*,*,#10359,.F.);
#14567=ORIENTED_EDGE('',*,*,#10289,.T.);
#14568=ORIENTED_EDGE('',*,*,#10360,.T.);
#14569=ORIENTED_EDGE('',*,*,#10355,.T.);
#14570=ORIENTED_EDGE('',*,*,#10347,.F.);
#14571=ORIENTED_EDGE('',*,*,#10361,.T.);
#14572=ORIENTED_EDGE('',*,*,#10362,.T.);
#14573=ORIENTED_EDGE('',*,*,#10363,.T.);
#14574=ORIENTED_EDGE('',*,*,#10364,.T.);
#14575=ORIENTED_EDGE('',*,*,#10345,.F.);
#14576=ORIENTED_EDGE('',*,*,#10365,.T.);
#14577=ORIENTED_EDGE('',*,*,#10363,.F.);
#14578=ORIENTED_EDGE('',*,*,#10366,.F.);
#14579=ORIENTED_EDGE('',*,*,#10277,.T.);
#14580=ORIENTED_EDGE('',*,*,#10367,.T.);
#14581=ORIENTED_EDGE('',*,*,#10368,.T.);
#14582=ORIENTED_EDGE('',*,*,#10369,.T.);
#14583=ORIENTED_EDGE('',*,*,#10370,.F.);
#14584=ORIENTED_EDGE('',*,*,#10367,.F.);
#14585=ORIENTED_EDGE('',*,*,#10371,.T.);
#14586=ORIENTED_EDGE('',*,*,#10361,.F.);
#14587=ORIENTED_EDGE('',*,*,#10368,.F.);
#14588=ORIENTED_EDGE('',*,*,#10372,.T.);
#14589=ORIENTED_EDGE('',*,*,#10372,.F.);
#14590=ORIENTED_EDGE('',*,*,#10337,.F.);
#14591=ORIENTED_EDGE('',*,*,#10373,.F.);
#14592=ORIENTED_EDGE('',*,*,#10374,.F.);
#14593=ORIENTED_EDGE('',*,*,#10375,.F.);
#14594=ORIENTED_EDGE('',*,*,#10376,.F.);
#14595=ORIENTED_EDGE('',*,*,#10377,.T.);
#14596=ORIENTED_EDGE('',*,*,#10378,.F.);
#14597=ORIENTED_EDGE('',*,*,#10336,.F.);
#14598=ORIENTED_EDGE('',*,*,#10346,.F.);
#14599=ORIENTED_EDGE('',*,*,#10362,.F.);
#14600=ORIENTED_EDGE('',*,*,#10379,.F.);
#14601=ORIENTED_EDGE('',*,*,#10373,.T.);
#14602=ORIENTED_EDGE('',*,*,#10371,.F.);
#14603=ORIENTED_EDGE('',*,*,#10276,.T.);
#14604=ORIENTED_EDGE('',*,*,#10292,.T.);
#14605=ORIENTED_EDGE('',*,*,#10380,.T.);
#14606=ORIENTED_EDGE('',*,*,#10374,.T.);
#14607=ORIENTED_EDGE('',*,*,#10379,.T.);
#14608=ORIENTED_EDGE('',*,*,#10291,.T.);
#14609=ORIENTED_EDGE('',*,*,#10381,.T.);
#14610=ORIENTED_EDGE('',*,*,#10375,.T.);
#14611=ORIENTED_EDGE('',*,*,#10380,.F.);
#14612=ORIENTED_EDGE('',*,*,#10343,.F.);
#14613=ORIENTED_EDGE('',*,*,#10382,.T.);
#14614=ORIENTED_EDGE('',*,*,#10383,.T.);
#14615=ORIENTED_EDGE('',*,*,#10357,.F.);
#14616=ORIENTED_EDGE('',*,*,#10360,.F.);
#14617=ORIENTED_EDGE('',*,*,#10288,.T.);
#14618=ORIENTED_EDGE('',*,*,#10384,.T.);
#14619=ORIENTED_EDGE('',*,*,#10350,.T.);
#14620=ORIENTED_EDGE('',*,*,#10356,.T.);
#14621=ORIENTED_EDGE('',*,*,#10287,.T.);
#14622=ORIENTED_EDGE('',*,*,#10385,.T.);
#14623=ORIENTED_EDGE('',*,*,#10351,.T.);
#14624=ORIENTED_EDGE('',*,*,#10384,.F.);
#14625=ORIENTED_EDGE('',*,*,#10304,.F.);
#14626=ORIENTED_EDGE('',*,*,#10386,.T.);
#14627=ORIENTED_EDGE('',*,*,#10387,.T.);
#14628=ORIENTED_EDGE('',*,*,#10333,.F.);
#14629=ORIENTED_EDGE('',*,*,#10313,.F.);
#14630=ORIENTED_EDGE('',*,*,#10388,.T.);
#14631=ORIENTED_EDGE('',*,*,#10331,.T.);
#14632=ORIENTED_EDGE('',*,*,#10389,.T.);
#14633=ORIENTED_EDGE('',*,*,#10390,.T.);
#14634=ORIENTED_EDGE('',*,*,#10388,.F.);
#14635=ORIENTED_EDGE('',*,*,#10391,.T.);
#14636=ORIENTED_EDGE('',*,*,#10329,.F.);
#14637=ORIENTED_EDGE('',*,*,#10332,.F.);
#14638=ORIENTED_EDGE('',*,*,#10392,.T.);
#14639=ORIENTED_EDGE('',*,*,#10389,.F.);
#14640=ORIENTED_EDGE('',*,*,#10391,.F.);
#14641=ORIENTED_EDGE('',*,*,#10393,.T.);
#14642=ORIENTED_EDGE('',*,*,#10394,.T.);
#14643=ORIENTED_EDGE('',*,*,#10315,.T.);
#14644=ORIENTED_EDGE('',*,*,#10390,.F.);
#14645=ORIENTED_EDGE('',*,*,#10395,.F.);
#14646=ORIENTED_EDGE('',*,*,#10396,.F.);
#14647=ORIENTED_EDGE('',*,*,#10397,.T.);
#14648=ORIENTED_EDGE('',*,*,#10398,.F.);
#14649=ORIENTED_EDGE('',*,*,#10393,.F.);
#14650=ORIENTED_EDGE('',*,*,#10392,.F.);
#14651=ORIENTED_EDGE('',*,*,#10283,.T.);
#14652=ORIENTED_EDGE('',*,*,#10399,.T.);
#14653=ORIENTED_EDGE('',*,*,#10395,.T.);
#14654=ORIENTED_EDGE('',*,*,#10400,.T.);
#14655=ORIENTED_EDGE('',*,*,#10279,.T.);
#14656=ORIENTED_EDGE('',*,*,#10401,.T.);
#14657=ORIENTED_EDGE('',*,*,#10402,.T.);
#14658=ORIENTED_EDGE('',*,*,#10403,.T.);
#14659=ORIENTED_EDGE('',*,*,#10404,.T.);
#14660=ORIENTED_EDGE('',*,*,#10405,.T.);
#14661=ORIENTED_EDGE('',*,*,#10406,.T.);
#14662=ORIENTED_EDGE('',*,*,#10403,.F.);
#14663=ORIENTED_EDGE('',*,*,#10407,.T.);
#14664=ORIENTED_EDGE('',*,*,#10408,.T.);
#14665=ORIENTED_EDGE('',*,*,#10405,.F.);
#14666=ORIENTED_EDGE('',*,*,#10409,.T.);
#14667=ORIENTED_EDGE('',*,*,#10400,.F.);
#14668=ORIENTED_EDGE('',*,*,#10409,.F.);
#14669=ORIENTED_EDGE('',*,*,#10410,.T.);
#14670=ORIENTED_EDGE('',*,*,#10411,.T.);
#14671=ORIENTED_EDGE('',*,*,#10280,.T.);
#14672=ORIENTED_EDGE('',*,*,#10404,.F.);
#14673=ORIENTED_EDGE('',*,*,#10412,.F.);
#14674=ORIENTED_EDGE('',*,*,#10413,.F.);
#14675=ORIENTED_EDGE('',*,*,#10410,.F.);
#14676=ORIENTED_EDGE('',*,*,#10414,.T.);
#14677=ORIENTED_EDGE('',*,*,#10415,.T.);
#14678=ORIENTED_EDGE('',*,*,#10401,.F.);
#14679=ORIENTED_EDGE('',*,*,#10278,.F.);
#14680=ORIENTED_EDGE('',*,*,#10366,.T.);
#14681=ORIENTED_EDGE('',*,*,#10414,.F.);
#14682=ORIENTED_EDGE('',*,*,#10370,.T.);
#14683=ORIENTED_EDGE('',*,*,#10416,.F.);
#14684=ORIENTED_EDGE('',*,*,#10417,.F.);
#14685=ORIENTED_EDGE('',*,*,#10418,.F.);
#14686=ORIENTED_EDGE('',*,*,#10419,.F.);
#14687=ORIENTED_EDGE('',*,*,#10411,.F.);
#14688=ORIENTED_EDGE('',*,*,#10420,.F.);
#14689=ORIENTED_EDGE('',*,*,#10421,.F.);
#14690=ORIENTED_EDGE('',*,*,#10420,.T.);
#14691=ORIENTED_EDGE('',*,*,#10413,.T.);
#14692=ORIENTED_EDGE('',*,*,#10422,.T.);
#14693=ORIENTED_EDGE('',*,*,#10423,.T.);
#14694=ORIENTED_EDGE('',*,*,#10424,.F.);
#14695=ORIENTED_EDGE('',*,*,#10281,.T.);
#14696=ORIENTED_EDGE('',*,*,#10421,.T.);
#14697=ORIENTED_EDGE('',*,*,#10425,.T.);
#14698=ORIENTED_EDGE('',*,*,#10426,.F.);
#14699=ORIENTED_EDGE('',*,*,#10408,.F.);
#14700=ORIENTED_EDGE('',*,*,#10318,.T.);
#14701=ORIENTED_EDGE('',*,*,#10427,.T.);
#14702=ORIENTED_EDGE('',*,*,#10412,.T.);
#14703=ORIENTED_EDGE('',*,*,#10407,.F.);
#14704=ORIENTED_EDGE('',*,*,#10428,.T.);
#14705=ORIENTED_EDGE('',*,*,#10429,.T.);
#14706=ORIENTED_EDGE('',*,*,#10319,.T.);
#14707=ORIENTED_EDGE('',*,*,#10430,.T.);
#14708=ORIENTED_EDGE('',*,*,#10320,.T.);
#14709=ORIENTED_EDGE('',*,*,#10429,.F.);
#14710=ORIENTED_EDGE('',*,*,#10431,.T.);
#14711=ORIENTED_EDGE('',*,*,#10365,.F.);
#14712=ORIENTED_EDGE('',*,*,#10321,.T.);
#14713=ORIENTED_EDGE('',*,*,#10430,.F.);
#14714=ORIENTED_EDGE('',*,*,#10432,.T.);
#14715=ORIENTED_EDGE('',*,*,#10427,.F.);
#14716=ORIENTED_EDGE('',*,*,#10433,.T.);
#14717=ORIENTED_EDGE('',*,*,#10422,.F.);
#14718=ORIENTED_EDGE('',*,*,#10402,.F.);
#14719=ORIENTED_EDGE('',*,*,#10415,.F.);
#14720=ORIENTED_EDGE('',*,*,#10418,.T.);
#14721=ORIENTED_EDGE('',*,*,#10434,.F.);
#14722=ORIENTED_EDGE('',*,*,#10428,.F.);
#14723=ORIENTED_EDGE('',*,*,#10406,.F.);
#14724=ORIENTED_EDGE('',*,*,#10425,.F.);
#14725=ORIENTED_EDGE('',*,*,#10423,.F.);
#14726=ORIENTED_EDGE('',*,*,#10435,.F.);
#14727=ORIENTED_EDGE('',*,*,#10436,.T.);
#14728=ORIENTED_EDGE('',*,*,#10437,.T.);
#14729=ORIENTED_EDGE('',*,*,#10433,.F.);
#14730=ORIENTED_EDGE('',*,*,#10317,.T.);
#14731=ORIENTED_EDGE('',*,*,#10438,.F.);
#14732=ORIENTED_EDGE('',*,*,#10435,.T.);
#14733=ORIENTED_EDGE('',*,*,#10438,.T.);
#14734=ORIENTED_EDGE('',*,*,#10316,.T.);
#14735=ORIENTED_EDGE('',*,*,#10394,.F.);
#14736=ORIENTED_EDGE('',*,*,#10439,.T.);
#14737=ORIENTED_EDGE('',*,*,#10439,.F.);
#14738=ORIENTED_EDGE('',*,*,#10398,.T.);
#14739=ORIENTED_EDGE('',*,*,#10440,.T.);
#14740=ORIENTED_EDGE('',*,*,#10436,.F.);
#14741=ORIENTED_EDGE('',*,*,#10419,.T.);
#14742=ORIENTED_EDGE('',*,*,#10441,.T.);
#14743=ORIENTED_EDGE('',*,*,#10442,.T.);
#14744=ORIENTED_EDGE('',*,*,#10441,.F.);
#14745=ORIENTED_EDGE('',*,*,#10442,.F.);
#14746=ORIENTED_EDGE('',*,*,#10443,.T.);
#14747=ORIENTED_EDGE('',*,*,#10444,.F.);
#14748=ORIENTED_EDGE('',*,*,#10445,.F.);
#14749=ORIENTED_EDGE('',*,*,#10443,.F.);
#14750=ORIENTED_EDGE('',*,*,#10446,.T.);
#14751=ORIENTED_EDGE('',*,*,#10447,.T.);
#14752=ORIENTED_EDGE('',*,*,#10448,.T.);
#14753=ORIENTED_EDGE('',*,*,#10449,.T.);
#14754=ORIENTED_EDGE('',*,*,#10450,.T.);
#14755=ORIENTED_EDGE('',*,*,#10446,.F.);
#14756=ORIENTED_EDGE('',*,*,#10451,.T.);
#14757=ORIENTED_EDGE('',*,*,#10452,.F.);
#14758=ORIENTED_EDGE('',*,*,#10451,.F.);
#14759=ORIENTED_EDGE('',*,*,#10453,.F.);
#14760=ORIENTED_EDGE('',*,*,#10454,.F.);
#14761=ORIENTED_EDGE('',*,*,#10455,.F.);
#14762=ORIENTED_EDGE('',*,*,#10456,.F.);
#14763=ORIENTED_EDGE('',*,*,#10448,.F.);
#14764=ORIENTED_EDGE('',*,*,#10457,.T.);
#14765=ORIENTED_EDGE('',*,*,#10458,.T.);
#14766=ORIENTED_EDGE('',*,*,#10453,.T.);
#14767=ORIENTED_EDGE('',*,*,#10459,.T.);
#14768=ORIENTED_EDGE('',*,*,#10460,.T.);
#14769=ORIENTED_EDGE('',*,*,#10461,.T.);
#14770=ORIENTED_EDGE('',*,*,#10462,.T.);
#14771=ORIENTED_EDGE('',*,*,#10463,.T.);
#14772=ORIENTED_EDGE('',*,*,#10464,.T.);
#14773=ORIENTED_EDGE('',*,*,#10461,.F.);
#14774=ORIENTED_EDGE('',*,*,#10465,.T.);
#14775=ORIENTED_EDGE('',*,*,#10466,.F.);
#14776=ORIENTED_EDGE('',*,*,#10467,.T.);
#14777=ORIENTED_EDGE('',*,*,#10468,.T.);
#14778=ORIENTED_EDGE('',*,*,#10460,.F.);
#14779=ORIENTED_EDGE('',*,*,#10469,.F.);
#14780=ORIENTED_EDGE('',*,*,#10470,.F.);
#14781=ORIENTED_EDGE('',*,*,#10465,.F.);
#14782=ORIENTED_EDGE('',*,*,#10459,.F.);
#14783=ORIENTED_EDGE('',*,*,#10471,.T.);
#14784=ORIENTED_EDGE('',*,*,#10472,.T.);
#14785=ORIENTED_EDGE('',*,*,#10473,.F.);
#14786=ORIENTED_EDGE('',*,*,#10469,.T.);
#14787=ORIENTED_EDGE('',*,*,#10474,.T.);
#14788=ORIENTED_EDGE('',*,*,#10456,.T.);
#14789=ORIENTED_EDGE('',*,*,#10475,.T.);
#14790=ORIENTED_EDGE('',*,*,#10470,.T.);
#14791=ORIENTED_EDGE('',*,*,#10467,.F.);
#14792=ORIENTED_EDGE('',*,*,#10476,.F.);
#14793=ORIENTED_EDGE('',*,*,#10477,.F.);
#14794=ORIENTED_EDGE('',*,*,#10478,.F.);
#14795=ORIENTED_EDGE('',*,*,#10472,.F.);
#14796=ORIENTED_EDGE('',*,*,#10479,.F.);
#14797=ORIENTED_EDGE('',*,*,#10480,.F.);
#14798=ORIENTED_EDGE('',*,*,#10481,.F.);
#14799=ORIENTED_EDGE('',*,*,#10464,.F.);
#14800=ORIENTED_EDGE('',*,*,#10482,.T.);
#14801=ORIENTED_EDGE('',*,*,#10483,.T.);
#14802=ORIENTED_EDGE('',*,*,#10484,.T.);
#14803=ORIENTED_EDGE('',*,*,#10479,.T.);
#14804=ORIENTED_EDGE('',*,*,#10471,.F.);
#14805=ORIENTED_EDGE('',*,*,#10485,.T.);
#14806=ORIENTED_EDGE('',*,*,#10352,.T.);
#14807=ORIENTED_EDGE('',*,*,#10385,.F.);
#14808=ORIENTED_EDGE('',*,*,#10286,.F.);
#14809=ORIENTED_EDGE('',*,*,#10335,.T.);
#14810=ORIENTED_EDGE('',*,*,#10485,.F.);
#14811=ORIENTED_EDGE('',*,*,#10334,.T.);
#14812=ORIENTED_EDGE('',*,*,#10387,.F.);
#14813=ORIENTED_EDGE('',*,*,#10486,.F.);
#14814=ORIENTED_EDGE('',*,*,#10353,.F.);
#14815=ORIENTED_EDGE('',*,*,#10487,.F.);
#14816=ORIENTED_EDGE('',*,*,#10487,.T.);
#14817=ORIENTED_EDGE('',*,*,#10488,.T.);
#14818=ORIENTED_EDGE('',*,*,#10489,.T.);
#14819=ORIENTED_EDGE('',*,*,#10488,.F.);
#14820=ORIENTED_EDGE('',*,*,#10489,.F.);
#14821=ORIENTED_EDGE('',*,*,#10490,.T.);
#14822=ORIENTED_EDGE('',*,*,#10491,.F.);
#14823=ORIENTED_EDGE('',*,*,#10492,.F.);
#14824=ORIENTED_EDGE('',*,*,#10490,.F.);
#14825=ORIENTED_EDGE('',*,*,#10493,.T.);
#14826=ORIENTED_EDGE('',*,*,#10455,.T.);
#14827=ORIENTED_EDGE('',*,*,#10494,.T.);
#14828=ORIENTED_EDGE('',*,*,#10495,.T.);
#14829=ORIENTED_EDGE('',*,*,#10493,.F.);
#14830=ORIENTED_EDGE('',*,*,#10496,.T.);
#14831=ORIENTED_EDGE('',*,*,#10466,.T.);
#14832=ORIENTED_EDGE('',*,*,#10475,.F.);
#14833=ORIENTED_EDGE('',*,*,#10497,.T.);
#14834=ORIENTED_EDGE('',*,*,#10498,.T.);
#14835=ORIENTED_EDGE('',*,*,#10449,.F.);
#14836=ORIENTED_EDGE('',*,*,#10452,.T.);
#14837=ORIENTED_EDGE('',*,*,#10499,.T.);
#14838=ORIENTED_EDGE('',*,*,#10497,.F.);
#14839=ORIENTED_EDGE('',*,*,#10474,.F.);
#14840=ORIENTED_EDGE('',*,*,#10473,.T.);
#14841=ORIENTED_EDGE('',*,*,#10496,.F.);
#14842=ORIENTED_EDGE('',*,*,#10500,.T.);
#14843=ORIENTED_EDGE('',*,*,#10501,.T.);
#14844=ORIENTED_EDGE('',*,*,#10476,.T.);
#14845=ORIENTED_EDGE('',*,*,#10502,.F.);
#14846=ORIENTED_EDGE('',*,*,#10503,.T.);
#14847=ORIENTED_EDGE('',*,*,#10501,.F.);
#14848=ORIENTED_EDGE('',*,*,#10504,.T.);
#14849=ORIENTED_EDGE('',*,*,#10504,.F.);
#14850=ORIENTED_EDGE('',*,*,#10505,.T.);
#14851=ORIENTED_EDGE('',*,*,#10506,.T.);
#14852=ORIENTED_EDGE('',*,*,#10507,.T.);
#14853=ORIENTED_EDGE('',*,*,#10495,.F.);
#14854=ORIENTED_EDGE('',*,*,#10508,.F.);
#14855=ORIENTED_EDGE('',*,*,#10505,.F.);
#14856=ORIENTED_EDGE('',*,*,#10500,.F.);
#14857=ORIENTED_EDGE('',*,*,#10462,.F.);
#14858=ORIENTED_EDGE('',*,*,#10468,.F.);
#14859=ORIENTED_EDGE('',*,*,#10478,.T.);
#14860=ORIENTED_EDGE('',*,*,#10509,.T.);
#14861=ORIENTED_EDGE('',*,*,#10510,.T.);
#14862=ORIENTED_EDGE('',*,*,#10503,.F.);
#14863=ORIENTED_EDGE('',*,*,#10511,.T.);
#14864=ORIENTED_EDGE('',*,*,#10512,.T.);
#14865=ORIENTED_EDGE('',*,*,#10477,.T.);
#14866=ORIENTED_EDGE('',*,*,#10512,.F.);
#14867=ORIENTED_EDGE('',*,*,#10513,.T.);
#14868=ORIENTED_EDGE('',*,*,#10509,.F.);
#14869=ORIENTED_EDGE('',*,*,#10463,.F.);
#14870=ORIENTED_EDGE('',*,*,#10510,.F.);
#14871=ORIENTED_EDGE('',*,*,#10514,.F.);
#14872=ORIENTED_EDGE('',*,*,#10482,.F.);
#14873=ORIENTED_EDGE('',*,*,#10513,.F.);
#14874=ORIENTED_EDGE('',*,*,#10515,.T.);
#14875=ORIENTED_EDGE('',*,*,#10516,.T.);
#14876=ORIENTED_EDGE('',*,*,#10483,.F.);
#14877=ORIENTED_EDGE('',*,*,#10514,.T.);
#14878=ORIENTED_EDGE('',*,*,#10511,.F.);
#14879=ORIENTED_EDGE('',*,*,#10517,.F.);
#14880=ORIENTED_EDGE('',*,*,#10518,.F.);
#14881=ORIENTED_EDGE('',*,*,#10515,.F.);
#14882=ORIENTED_EDGE('',*,*,#10519,.T.);
#14883=ORIENTED_EDGE('',*,*,#10520,.T.);
#14884=ORIENTED_EDGE('',*,*,#10521,.T.);
#14885=ORIENTED_EDGE('',*,*,#10520,.F.);
#14886=ORIENTED_EDGE('',*,*,#10522,.T.);
#14887=ORIENTED_EDGE('',*,*,#10523,.F.);
#14888=ORIENTED_EDGE('',*,*,#10524,.T.);
#14889=ORIENTED_EDGE('',*,*,#10522,.F.);
#14890=ORIENTED_EDGE('',*,*,#10519,.F.);
#14891=ORIENTED_EDGE('',*,*,#10524,.F.);
#14892=ORIENTED_EDGE('',*,*,#10525,.F.);
#14893=ORIENTED_EDGE('',*,*,#10521,.F.);
#14894=ORIENTED_EDGE('',*,*,#10526,.T.);
#14895=ORIENTED_EDGE('',*,*,#10527,.T.);
#14896=ORIENTED_EDGE('',*,*,#10528,.T.);
#14897=ORIENTED_EDGE('',*,*,#10529,.T.);
#14898=ORIENTED_EDGE('',*,*,#10525,.T.);
#14899=ORIENTED_EDGE('',*,*,#10523,.T.);
#14900=ORIENTED_EDGE('',*,*,#10529,.F.);
#14901=ORIENTED_EDGE('',*,*,#10530,.F.);
#14902=ORIENTED_EDGE('',*,*,#10531,.T.);
#14903=ORIENTED_EDGE('',*,*,#10527,.F.);
#14904=ORIENTED_EDGE('',*,*,#10528,.F.);
#14905=ORIENTED_EDGE('',*,*,#10531,.F.);
#14906=ORIENTED_EDGE('',*,*,#10532,.F.);
#14907=ORIENTED_EDGE('',*,*,#10533,.T.);
#14908=ORIENTED_EDGE('',*,*,#10376,.T.);
#14909=ORIENTED_EDGE('',*,*,#10381,.F.);
#14910=ORIENTED_EDGE('',*,*,#10290,.F.);
#14911=ORIENTED_EDGE('',*,*,#10359,.T.);
#14912=ORIENTED_EDGE('',*,*,#10533,.F.);
#14913=ORIENTED_EDGE('',*,*,#10358,.T.);
#14914=ORIENTED_EDGE('',*,*,#10383,.F.);
#14915=ORIENTED_EDGE('',*,*,#10534,.F.);
#14916=ORIENTED_EDGE('',*,*,#10377,.F.);
#14917=ORIENTED_EDGE('',*,*,#10535,.F.);
#14918=ORIENTED_EDGE('',*,*,#10536,.T.);
#14919=ORIENTED_EDGE('',*,*,#10396,.T.);
#14920=ORIENTED_EDGE('',*,*,#10399,.F.);
#14921=ORIENTED_EDGE('',*,*,#10282,.F.);
#14922=ORIENTED_EDGE('',*,*,#10424,.T.);
#14923=ORIENTED_EDGE('',*,*,#10536,.F.);
#14924=ORIENTED_EDGE('',*,*,#10426,.T.);
#14925=ORIENTED_EDGE('',*,*,#10437,.F.);
#14926=ORIENTED_EDGE('',*,*,#10440,.F.);
#14927=ORIENTED_EDGE('',*,*,#10397,.F.);
#14928=ORIENTED_EDGE('',*,*,#10537,.F.);
#14929=ORIENTED_EDGE('',*,*,#10484,.F.);
#14930=ORIENTED_EDGE('',*,*,#10516,.F.);
#14931=ORIENTED_EDGE('',*,*,#10518,.T.);
#14932=ORIENTED_EDGE('',*,*,#10538,.F.);
#14933=ORIENTED_EDGE('',*,*,#10539,.F.);
#14934=ORIENTED_EDGE('',*,*,#10480,.T.);
#14935=ORIENTED_EDGE('',*,*,#10499,.F.);
#14936=ORIENTED_EDGE('',*,*,#10481,.T.);
#14937=ORIENTED_EDGE('',*,*,#10539,.T.);
#14938=ORIENTED_EDGE('',*,*,#10540,.T.);
#14939=ORIENTED_EDGE('',*,*,#10498,.F.);
#14940=ORIENTED_EDGE('',*,*,#10540,.F.);
#14941=ORIENTED_EDGE('',*,*,#10541,.F.);
#14942=ORIENTED_EDGE('',*,*,#10542,.T.);
#14943=ORIENTED_EDGE('',*,*,#10502,.T.);
#14944=ORIENTED_EDGE('',*,*,#10543,.T.);
#14945=ORIENTED_EDGE('',*,*,#10544,.T.);
#14946=ORIENTED_EDGE('',*,*,#10517,.T.);
#14947=ORIENTED_EDGE('',*,*,#10538,.T.);
#14948=ORIENTED_EDGE('',*,*,#10544,.F.);
#14949=ORIENTED_EDGE('',*,*,#10545,.T.);
#14950=ORIENTED_EDGE('',*,*,#10507,.F.);
#14951=ORIENTED_EDGE('',*,*,#10546,.F.);
#14952=ORIENTED_EDGE('',*,*,#10547,.F.);
#14953=ORIENTED_EDGE('',*,*,#10548,.F.);
#14954=ORIENTED_EDGE('',*,*,#10549,.F.);
#14955=ORIENTED_EDGE('',*,*,#10543,.F.);
#14956=ORIENTED_EDGE('',*,*,#10545,.F.);
#14957=ORIENTED_EDGE('',*,*,#10549,.T.);
#14958=ORIENTED_EDGE('',*,*,#10550,.T.);
#14959=ORIENTED_EDGE('',*,*,#10541,.T.);
#14960=ORIENTED_EDGE('',*,*,#10537,.T.);
#14961=ORIENTED_EDGE('',*,*,#10551,.T.);
#14962=ORIENTED_EDGE('',*,*,#10552,.T.);
#14963=ORIENTED_EDGE('',*,*,#10551,.F.);
#14964=ORIENTED_EDGE('',*,*,#10552,.F.);
#14965=ORIENTED_EDGE('',*,*,#10553,.T.);
#14966=ORIENTED_EDGE('',*,*,#10554,.F.);
#14967=ORIENTED_EDGE('',*,*,#10555,.F.);
#14968=ORIENTED_EDGE('',*,*,#10553,.F.);
#14969=ORIENTED_EDGE('',*,*,#10535,.T.);
#14970=ORIENTED_EDGE('',*,*,#10556,.T.);
#14971=ORIENTED_EDGE('',*,*,#10557,.T.);
#14972=ORIENTED_EDGE('',*,*,#10556,.F.);
#14973=ORIENTED_EDGE('',*,*,#10557,.F.);
#14974=ORIENTED_EDGE('',*,*,#10558,.T.);
#14975=ORIENTED_EDGE('',*,*,#10559,.F.);
#14976=ORIENTED_EDGE('',*,*,#10560,.F.);
#14977=ORIENTED_EDGE('',*,*,#10558,.F.);
#14978=ORIENTED_EDGE('',*,*,#10561,.T.);
#14979=ORIENTED_EDGE('',*,*,#10562,.T.);
#14980=ORIENTED_EDGE('',*,*,#10563,.T.);
#14981=ORIENTED_EDGE('',*,*,#10564,.T.);
#14982=ORIENTED_EDGE('',*,*,#10562,.F.);
#14983=ORIENTED_EDGE('',*,*,#10565,.F.);
#14984=ORIENTED_EDGE('',*,*,#10566,.F.);
#14985=ORIENTED_EDGE('',*,*,#10567,.F.);
#14986=ORIENTED_EDGE('',*,*,#10568,.F.);
#14987=ORIENTED_EDGE('',*,*,#10569,.F.);
#14988=ORIENTED_EDGE('',*,*,#10570,.T.);
#14989=ORIENTED_EDGE('',*,*,#10571,.T.);
#14990=ORIENTED_EDGE('',*,*,#10572,.T.);
#14991=ORIENTED_EDGE('',*,*,#10573,.F.);
#14992=ORIENTED_EDGE('',*,*,#10574,.F.);
#14993=ORIENTED_EDGE('',*,*,#10575,.F.);
#14994=ORIENTED_EDGE('',*,*,#10561,.F.);
#14995=ORIENTED_EDGE('',*,*,#10576,.F.);
#14996=ORIENTED_EDGE('',*,*,#10577,.T.);
#14997=ORIENTED_EDGE('',*,*,#10563,.F.);
#14998=ORIENTED_EDGE('',*,*,#10564,.F.);
#14999=ORIENTED_EDGE('',*,*,#10577,.F.);
#15000=ORIENTED_EDGE('',*,*,#10566,.T.);
#15001=ORIENTED_EDGE('',*,*,#10578,.T.);
#15002=ORIENTED_EDGE('',*,*,#10579,.T.);
#15003=ORIENTED_EDGE('',*,*,#10580,.T.);
#15004=ORIENTED_EDGE('',*,*,#10578,.F.);
#15005=ORIENTED_EDGE('',*,*,#10581,.F.);
#15006=ORIENTED_EDGE('',*,*,#10582,.T.);
#15007=ORIENTED_EDGE('',*,*,#10579,.F.);
#15008=ORIENTED_EDGE('',*,*,#10580,.F.);
#15009=ORIENTED_EDGE('',*,*,#10582,.F.);
#15010=ORIENTED_EDGE('',*,*,#10565,.T.);
#15011=ORIENTED_EDGE('',*,*,#10583,.T.);
#15012=ORIENTED_EDGE('',*,*,#10532,.T.);
#15013=ORIENTED_EDGE('',*,*,#10530,.T.);
#15014=ORIENTED_EDGE('',*,*,#10583,.F.);
#15015=ORIENTED_EDGE('',*,*,#10567,.T.);
#15016=ORIENTED_EDGE('',*,*,#10584,.T.);
#15017=ORIENTED_EDGE('',*,*,#10491,.T.);
#15018=ORIENTED_EDGE('',*,*,#10492,.T.);
#15019=ORIENTED_EDGE('',*,*,#10584,.F.);
#15020=ORIENTED_EDGE('',*,*,#10575,.T.);
#15021=ORIENTED_EDGE('',*,*,#10585,.T.);
#15022=ORIENTED_EDGE('',*,*,#10444,.T.);
#15023=ORIENTED_EDGE('',*,*,#10445,.T.);
#15024=ORIENTED_EDGE('',*,*,#10585,.F.);
#15025=ORIENTED_EDGE('',*,*,#10568,.T.);
#15026=ORIENTED_EDGE('',*,*,#10586,.T.);
#15027=ORIENTED_EDGE('',*,*,#10587,.T.);
#15028=ORIENTED_EDGE('',*,*,#10588,.T.);
#15029=ORIENTED_EDGE('',*,*,#10586,.F.);
#15030=ORIENTED_EDGE('',*,*,#10589,.F.);
#15031=ORIENTED_EDGE('',*,*,#10590,.T.);
#15032=ORIENTED_EDGE('',*,*,#10587,.F.);
#15033=ORIENTED_EDGE('',*,*,#10588,.F.);
#15034=ORIENTED_EDGE('',*,*,#10590,.F.);
#15035=ORIENTED_EDGE('',*,*,#10574,.T.);
#15036=ORIENTED_EDGE('',*,*,#10591,.T.);
#15037=ORIENTED_EDGE('',*,*,#10559,.T.);
#15038=ORIENTED_EDGE('',*,*,#10560,.T.);
#15039=ORIENTED_EDGE('',*,*,#10591,.F.);
#15040=ORIENTED_EDGE('',*,*,#10569,.T.);
#15041=ORIENTED_EDGE('',*,*,#10592,.T.);
#15042=ORIENTED_EDGE('',*,*,#10554,.T.);
#15043=ORIENTED_EDGE('',*,*,#10555,.T.);
#15044=ORIENTED_EDGE('',*,*,#10592,.F.);
#15045=ORIENTED_EDGE('',*,*,#10593,.T.);
#15046=ORIENTED_EDGE('',*,*,#10594,.T.);
#15047=ORIENTED_EDGE('',*,*,#10595,.T.);
#15048=ORIENTED_EDGE('',*,*,#10594,.F.);
#15049=ORIENTED_EDGE('',*,*,#10596,.F.);
#15050=ORIENTED_EDGE('',*,*,#10597,.T.);
#15051=ORIENTED_EDGE('',*,*,#10593,.F.);
#15052=ORIENTED_EDGE('',*,*,#10597,.F.);
#15053=ORIENTED_EDGE('',*,*,#10598,.T.);
#15054=ORIENTED_EDGE('',*,*,#10595,.F.);
#15055=ORIENTED_EDGE('',*,*,#10599,.T.);
#15056=ORIENTED_EDGE('',*,*,#10600,.T.);
#15057=ORIENTED_EDGE('',*,*,#10601,.T.);
#15058=ORIENTED_EDGE('',*,*,#10600,.F.);
#15059=ORIENTED_EDGE('',*,*,#10602,.F.);
#15060=ORIENTED_EDGE('',*,*,#10603,.T.);
#15061=ORIENTED_EDGE('',*,*,#10599,.F.);
#15062=ORIENTED_EDGE('',*,*,#10603,.F.);
#15063=ORIENTED_EDGE('',*,*,#10604,.T.);
#15064=ORIENTED_EDGE('',*,*,#10601,.F.);
#15065=ORIENTED_EDGE('',*,*,#10605,.T.);
#15066=ORIENTED_EDGE('',*,*,#10606,.T.);
#15067=ORIENTED_EDGE('',*,*,#10607,.T.);
#15068=ORIENTED_EDGE('',*,*,#10606,.F.);
#15069=ORIENTED_EDGE('',*,*,#10608,.F.);
#15070=ORIENTED_EDGE('',*,*,#10609,.T.);
#15071=ORIENTED_EDGE('',*,*,#10605,.F.);
#15072=ORIENTED_EDGE('',*,*,#10609,.F.);
#15073=ORIENTED_EDGE('',*,*,#10610,.T.);
#15074=ORIENTED_EDGE('',*,*,#10607,.F.);
#15075=ORIENTED_EDGE('',*,*,#10447,.F.);
#15076=ORIENTED_EDGE('',*,*,#10611,.T.);
#15077=ORIENTED_EDGE('',*,*,#10612,.T.);
#15078=ORIENTED_EDGE('',*,*,#10613,.T.);
#15079=ORIENTED_EDGE('',*,*,#10614,.T.);
#15080=ORIENTED_EDGE('',*,*,#10615,.T.);
#15081=ORIENTED_EDGE('',*,*,#10550,.F.);
#15082=ORIENTED_EDGE('',*,*,#10548,.T.);
#15083=ORIENTED_EDGE('',*,*,#10614,.F.);
#15084=ORIENTED_EDGE('',*,*,#10616,.T.);
#15085=ORIENTED_EDGE('',*,*,#10612,.F.);
#15086=ORIENTED_EDGE('',*,*,#10617,.F.);
#15087=ORIENTED_EDGE('',*,*,#10457,.F.);
#15088=ORIENTED_EDGE('',*,*,#10613,.F.);
#15089=ORIENTED_EDGE('',*,*,#10618,.F.);
#15090=ORIENTED_EDGE('',*,*,#10619,.F.);
#15091=ORIENTED_EDGE('',*,*,#10620,.F.);
#15092=ORIENTED_EDGE('',*,*,#10621,.F.);
#15093=ORIENTED_EDGE('',*,*,#10622,.T.);
#15094=ORIENTED_EDGE('',*,*,#10616,.F.);
#15095=ORIENTED_EDGE('',*,*,#10547,.T.);
#15096=ORIENTED_EDGE('',*,*,#10623,.F.);
#15097=ORIENTED_EDGE('',*,*,#10624,.F.);
#15098=ORIENTED_EDGE('',*,*,#10618,.T.);
#15099=ORIENTED_EDGE('',*,*,#10625,.T.);
#15100=ORIENTED_EDGE('',*,*,#10626,.T.);
#15101=ORIENTED_EDGE('',*,*,#10627,.T.);
#15102=ORIENTED_EDGE('',*,*,#10628,.T.);
#15103=ORIENTED_EDGE('',*,*,#10629,.T.);
#15104=ORIENTED_EDGE('',*,*,#10627,.F.);
#15105=ORIENTED_EDGE('',*,*,#10629,.F.);
#15106=ORIENTED_EDGE('',*,*,#10630,.T.);
#15107=ORIENTED_EDGE('',*,*,#10631,.F.);
#15108=ORIENTED_EDGE('',*,*,#10632,.F.);
#15109=ORIENTED_EDGE('',*,*,#10630,.F.);
#15110=ORIENTED_EDGE('',*,*,#10628,.F.);
#15111=ORIENTED_EDGE('',*,*,#10633,.F.);
#15112=ORIENTED_EDGE('',*,*,#10634,.T.);
#15113=ORIENTED_EDGE('',*,*,#10625,.F.);
#15114=ORIENTED_EDGE('',*,*,#10626,.F.);
#15115=ORIENTED_EDGE('',*,*,#10634,.F.);
#15116=ORIENTED_EDGE('',*,*,#10635,.F.);
#15117=ORIENTED_EDGE('',*,*,#10631,.T.);
#15118=ORIENTED_EDGE('',*,*,#10632,.T.);
#15119=ORIENTED_EDGE('',*,*,#10636,.T.);
#15120=ORIENTED_EDGE('',*,*,#10637,.T.);
#15121=ORIENTED_EDGE('',*,*,#10636,.F.);
#15122=ORIENTED_EDGE('',*,*,#10637,.F.);
#15123=ORIENTED_EDGE('',*,*,#10638,.F.);
#15124=ORIENTED_EDGE('',*,*,#10639,.F.);
#15125=ORIENTED_EDGE('',*,*,#10640,.T.);
#15126=ORIENTED_EDGE('',*,*,#10641,.T.);
#15127=ORIENTED_EDGE('',*,*,#10642,.T.);
#15128=ORIENTED_EDGE('',*,*,#10643,.F.);
#15129=ORIENTED_EDGE('',*,*,#10644,.F.);
#15130=ORIENTED_EDGE('',*,*,#10638,.T.);
#15131=ORIENTED_EDGE('',*,*,#10645,.T.);
#15132=ORIENTED_EDGE('',*,*,#10608,.T.);
#15133=ORIENTED_EDGE('',*,*,#10645,.F.);
#15134=ORIENTED_EDGE('',*,*,#10644,.T.);
#15135=ORIENTED_EDGE('',*,*,#10646,.T.);
#15136=ORIENTED_EDGE('',*,*,#10602,.T.);
#15137=ORIENTED_EDGE('',*,*,#10646,.F.);
#15138=ORIENTED_EDGE('',*,*,#10639,.T.);
#15139=ORIENTED_EDGE('',*,*,#10647,.T.);
#15140=ORIENTED_EDGE('',*,*,#10596,.T.);
#15141=ORIENTED_EDGE('',*,*,#10647,.F.);
#15142=ORIENTED_EDGE('',*,*,#10648,.T.);
#15143=ORIENTED_EDGE('',*,*,#10649,.T.);
#15144=ORIENTED_EDGE('',*,*,#10650,.T.);
#15145=ORIENTED_EDGE('',*,*,#10573,.T.);
#15146=ORIENTED_EDGE('',*,*,#10650,.F.);
#15147=ORIENTED_EDGE('',*,*,#10648,.F.);
#15148=ORIENTED_EDGE('',*,*,#10649,.F.);
#15149=ORIENTED_EDGE('',*,*,#10651,.T.);
#15150=ORIENTED_EDGE('',*,*,#10652,.F.);
#15151=ORIENTED_EDGE('',*,*,#10653,.F.);
#15152=ORIENTED_EDGE('',*,*,#10651,.F.);
#15153=ORIENTED_EDGE('',*,*,#10654,.T.);
#15154=ORIENTED_EDGE('',*,*,#10655,.T.);
#15155=ORIENTED_EDGE('',*,*,#10327,.T.);
#15156=ORIENTED_EDGE('',*,*,#10655,.F.);
#15157=ORIENTED_EDGE('',*,*,#10656,.T.);
#15158=ORIENTED_EDGE('',*,*,#10654,.F.);
#15159=ORIENTED_EDGE('',*,*,#10657,.T.);
#15160=ORIENTED_EDGE('',*,*,#10658,.F.);
#15161=ORIENTED_EDGE('',*,*,#10659,.F.);
#15162=ORIENTED_EDGE('',*,*,#10657,.F.);
#15163=ORIENTED_EDGE('',*,*,#10656,.F.);
#15164=ORIENTED_EDGE('',*,*,#10659,.T.);
#15165=ORIENTED_EDGE('',*,*,#10660,.T.);
#15166=ORIENTED_EDGE('',*,*,#10652,.T.);
#15167=ORIENTED_EDGE('',*,*,#10653,.T.);
#15168=ORIENTED_EDGE('',*,*,#10660,.F.);
#15169=ORIENTED_EDGE('',*,*,#10658,.T.);
#15170=ORIENTED_EDGE('',*,*,#10643,.T.);
#15171=ORIENTED_EDGE('',*,*,#10661,.T.);
#15172=ORIENTED_EDGE('',*,*,#10662,.T.);
#15173=ORIENTED_EDGE('',*,*,#10663,.T.);
#15174=ORIENTED_EDGE('',*,*,#10661,.F.);
#15175=ORIENTED_EDGE('',*,*,#10664,.F.);
#15176=ORIENTED_EDGE('',*,*,#10665,.T.);
#15177=ORIENTED_EDGE('',*,*,#10662,.F.);
#15178=ORIENTED_EDGE('',*,*,#10663,.F.);
#15179=ORIENTED_EDGE('',*,*,#10665,.F.);
#15180=ORIENTED_EDGE('',*,*,#10666,.F.);
#15181=ORIENTED_EDGE('',*,*,#10667,.T.);
#15182=ORIENTED_EDGE('',*,*,#10668,.T.);
#15183=ORIENTED_EDGE('',*,*,#10669,.T.);
#15184=ORIENTED_EDGE('',*,*,#10635,.T.);
#15185=ORIENTED_EDGE('',*,*,#10633,.T.);
#15186=ORIENTED_EDGE('',*,*,#10669,.F.);
#15187=ORIENTED_EDGE('',*,*,#10622,.F.);
#15188=ORIENTED_EDGE('',*,*,#10670,.F.);
#15189=ORIENTED_EDGE('',*,*,#10671,.T.);
#15190=ORIENTED_EDGE('',*,*,#10667,.F.);
#15191=ORIENTED_EDGE('',*,*,#10668,.F.);
#15192=ORIENTED_EDGE('',*,*,#10671,.F.);
#15193=ORIENTED_EDGE('',*,*,#10672,.F.);
#15194=ORIENTED_EDGE('',*,*,#10673,.F.);
#15195=ORIENTED_EDGE('',*,*,#10674,.F.);
#15196=ORIENTED_EDGE('',*,*,#10675,.T.);
#15197=ORIENTED_EDGE('',*,*,#10028,.F.);
#15198=ORIENTED_EDGE('',*,*,#10063,.F.);
#15199=ORIENTED_EDGE('',*,*,#10676,.T.);
#15200=ORIENTED_EDGE('',*,*,#10061,.T.);
#15201=ORIENTED_EDGE('',*,*,#10068,.T.);
#15202=ORIENTED_EDGE('',*,*,#10677,.T.);
#15203=ORIENTED_EDGE('',*,*,#10134,.F.);
#15204=ORIENTED_EDGE('',*,*,#10128,.F.);
#15205=ORIENTED_EDGE('',*,*,#10678,.T.);
#15206=ORIENTED_EDGE('',*,*,#10126,.T.);
#15207=ORIENTED_EDGE('',*,*,#10115,.T.);
#15208=ORIENTED_EDGE('',*,*,#10679,.T.);
#15209=ORIENTED_EDGE('',*,*,#10262,.F.);
#15210=ORIENTED_EDGE('',*,*,#10680,.F.);
#15211=ORIENTED_EDGE('',*,*,#10681,.T.);
#15212=ORIENTED_EDGE('',*,*,#10682,.F.);
#15213=ORIENTED_EDGE('',*,*,#10672,.T.);
#15214=ORIENTED_EDGE('',*,*,#10670,.T.);
#15215=ORIENTED_EDGE('',*,*,#10621,.T.);
#15216=ORIENTED_EDGE('',*,*,#10683,.T.);
#15217=ORIENTED_EDGE('',*,*,#10619,.T.);
#15218=ORIENTED_EDGE('',*,*,#10624,.T.);
#15219=ORIENTED_EDGE('',*,*,#10684,.T.);
#15220=ORIENTED_EDGE('',*,*,#10685,.T.);
#15221=ORIENTED_EDGE('',*,*,#10686,.T.);
#15222=ORIENTED_EDGE('',*,*,#10687,.T.);
#15223=ORIENTED_EDGE('',*,*,#10685,.F.);
#15224=ORIENTED_EDGE('',*,*,#10675,.F.);
#15225=ORIENTED_EDGE('',*,*,#10623,.T.);
#15226=ORIENTED_EDGE('',*,*,#10546,.T.);
#15227=ORIENTED_EDGE('',*,*,#10506,.F.);
#15228=ORIENTED_EDGE('',*,*,#10508,.T.);
#15229=ORIENTED_EDGE('',*,*,#10494,.F.);
#15230=ORIENTED_EDGE('',*,*,#10454,.T.);
#15231=ORIENTED_EDGE('',*,*,#10458,.F.);
#15232=ORIENTED_EDGE('',*,*,#10617,.T.);
#15233=ORIENTED_EDGE('',*,*,#10674,.T.);
#15234=ORIENTED_EDGE('',*,*,#10688,.T.);
#15235=ORIENTED_EDGE('',*,*,#10184,.T.);
#15236=ORIENTED_EDGE('',*,*,#10245,.T.);
#15237=ORIENTED_EDGE('',*,*,#10233,.F.);
#15238=ORIENTED_EDGE('',*,*,#10235,.T.);
#15239=ORIENTED_EDGE('',*,*,#10197,.F.);
#15240=ORIENTED_EDGE('',*,*,#10253,.T.);
#15241=ORIENTED_EDGE('',*,*,#10263,.F.);
#15242=ORIENTED_EDGE('',*,*,#10679,.F.);
#15243=ORIENTED_EDGE('',*,*,#10119,.T.);
#15244=ORIENTED_EDGE('',*,*,#10132,.T.);
#15245=ORIENTED_EDGE('',*,*,#10071,.F.);
#15246=ORIENTED_EDGE('',*,*,#10082,.T.);
#15247=ORIENTED_EDGE('',*,*,#10159,.F.);
#15248=ORIENTED_EDGE('',*,*,#10156,.T.);
#15249=ORIENTED_EDGE('',*,*,#10135,.F.);
#15250=ORIENTED_EDGE('',*,*,#10677,.F.);
#15251=ORIENTED_EDGE('',*,*,#10067,.T.);
#15252=ORIENTED_EDGE('',*,*,#10048,.T.);
#15253=ORIENTED_EDGE('',*,*,#10046,.F.);
#15254=ORIENTED_EDGE('',*,*,#10689,.T.);
#15255=ORIENTED_EDGE('',*,*,#10017,.F.);
#15256=ORIENTED_EDGE('',*,*,#10021,.T.);
#15257=ORIENTED_EDGE('',*,*,#10029,.F.);
#15258=ORIENTED_EDGE('',*,*,#10690,.F.);
#15259=ORIENTED_EDGE('',*,*,#10691,.F.);
#15260=ORIENTED_EDGE('',*,*,#10692,.F.);
#15261=ORIENTED_EDGE('',*,*,#10684,.F.);
#15262=ORIENTED_EDGE('',*,*,#10610,.F.);
#15263=ORIENTED_EDGE('',*,*,#10693,.T.);
#15264=ORIENTED_EDGE('',*,*,#10686,.F.);
#15265=ORIENTED_EDGE('',*,*,#10687,.F.);
#15266=ORIENTED_EDGE('',*,*,#10693,.F.);
#15267=ORIENTED_EDGE('',*,*,#10690,.T.);
#15268=ORIENTED_EDGE('',*,*,#10694,.T.);
#15269=ORIENTED_EDGE('',*,*,#10695,.T.);
#15270=ORIENTED_EDGE('',*,*,#10696,.T.);
#15271=ORIENTED_EDGE('',*,*,#10694,.F.);
#15272=ORIENTED_EDGE('',*,*,#10604,.F.);
#15273=ORIENTED_EDGE('',*,*,#10697,.T.);
#15274=ORIENTED_EDGE('',*,*,#10695,.F.);
#15275=ORIENTED_EDGE('',*,*,#10696,.F.);
#15276=ORIENTED_EDGE('',*,*,#10697,.F.);
#15277=ORIENTED_EDGE('',*,*,#10692,.T.);
#15278=ORIENTED_EDGE('',*,*,#10698,.T.);
#15279=ORIENTED_EDGE('',*,*,#10699,.T.);
#15280=ORIENTED_EDGE('',*,*,#10700,.T.);
#15281=ORIENTED_EDGE('',*,*,#10698,.F.);
#15282=ORIENTED_EDGE('',*,*,#10598,.F.);
#15283=ORIENTED_EDGE('',*,*,#10701,.T.);
#15284=ORIENTED_EDGE('',*,*,#10699,.F.);
#15285=ORIENTED_EDGE('',*,*,#10700,.F.);
#15286=ORIENTED_EDGE('',*,*,#10701,.F.);
#15287=ORIENTED_EDGE('',*,*,#10702,.T.);
#15288=ORIENTED_EDGE('',*,*,#10703,.T.);
#15289=ORIENTED_EDGE('',*,*,#10666,.T.);
#15290=ORIENTED_EDGE('',*,*,#10664,.T.);
#15291=ORIENTED_EDGE('',*,*,#10703,.F.);
#15292=ORIENTED_EDGE('',*,*,#10704,.T.);
#15293=ORIENTED_EDGE('',*,*,#10702,.F.);
#15294=ORIENTED_EDGE('',*,*,#10705,.T.);
#15295=ORIENTED_EDGE('',*,*,#10706,.F.);
#15296=ORIENTED_EDGE('',*,*,#10707,.F.);
#15297=ORIENTED_EDGE('',*,*,#10705,.F.);
#15298=ORIENTED_EDGE('',*,*,#10704,.F.);
#15299=ORIENTED_EDGE('',*,*,#10707,.T.);
#15300=ORIENTED_EDGE('',*,*,#10708,.T.);
#15301=ORIENTED_EDGE('',*,*,#10691,.T.);
#15302=ORIENTED_EDGE('',*,*,#10708,.F.);
#15303=ORIENTED_EDGE('',*,*,#10706,.T.);
#15304=ORIENTED_EDGE('',*,*,#10364,.F.);
#15305=ORIENTED_EDGE('',*,*,#10432,.F.);
#15306=ORIENTED_EDGE('',*,*,#10709,.T.);
#15307=ORIENTED_EDGE('',*,*,#10416,.T.);
#15308=ORIENTED_EDGE('',*,*,#10369,.F.);
#15309=ORIENTED_EDGE('',*,*,#10431,.F.);
#15310=ORIENTED_EDGE('',*,*,#10434,.T.);
#15311=ORIENTED_EDGE('',*,*,#10417,.T.);
#15312=ORIENTED_EDGE('',*,*,#10709,.F.);
#15313=ORIENTED_EDGE('',*,*,#10341,.F.);
#15314=ORIENTED_EDGE('',*,*,#10378,.T.);
#15315=ORIENTED_EDGE('',*,*,#10534,.T.);
#15316=ORIENTED_EDGE('',*,*,#10382,.F.);
#15317=ORIENTED_EDGE('',*,*,#10301,.F.);
#15318=ORIENTED_EDGE('',*,*,#10354,.T.);
#15319=ORIENTED_EDGE('',*,*,#10486,.T.);
#15320=ORIENTED_EDGE('',*,*,#10386,.F.);
#15321=ORIENTED_EDGE('',*,*,#10589,.T.);
#15322=ORIENTED_EDGE('',*,*,#10576,.T.);
#15323=ORIENTED_EDGE('',*,*,#10581,.T.);
#15324=ORIENTED_EDGE('',*,*,#10688,.F.);
#15325=ORIENTED_EDGE('',*,*,#10673,.T.);
#15326=ORIENTED_EDGE('',*,*,#10682,.T.);
#15327=ORIENTED_EDGE('',*,*,#10710,.F.);
#15328=ORIENTED_EDGE('',*,*,#10680,.T.);
#15329=ORIENTED_EDGE('',*,*,#10261,.F.);
#15330=ORIENTED_EDGE('',*,*,#10180,.F.);
#15331=ORIENTED_EDGE('',*,*,#10185,.F.);
#15332=ORIENTED_EDGE('',*,*,#10681,.F.);
#15333=ORIENTED_EDGE('',*,*,#10710,.T.);
#15334=ORIENTED_EDGE('',*,*,#10678,.F.);
#15335=ORIENTED_EDGE('',*,*,#10127,.T.);
#15336=ORIENTED_EDGE('',*,*,#10676,.F.);
#15337=ORIENTED_EDGE('',*,*,#10062,.T.);
#15338=ORIENTED_EDGE('',*,*,#10450,.F.);
#15339=ORIENTED_EDGE('',*,*,#10542,.F.);
#15340=ORIENTED_EDGE('',*,*,#10615,.F.);
#15341=ORIENTED_EDGE('',*,*,#10611,.F.);
#15342=ORIENTED_EDGE('',*,*,#10683,.F.);
#15343=ORIENTED_EDGE('',*,*,#10620,.T.);
#15344=ORIENTED_EDGE('',*,*,#9976,.F.);
#15345=ORIENTED_EDGE('',*,*,#10018,.F.);
#15346=ORIENTED_EDGE('',*,*,#10689,.F.);
#15347=ORIENTED_EDGE('',*,*,#10045,.F.);
#15348=ORIENTED_EDGE('',*,*,#10293,.T.);
#15349=ORIENTED_EDGE('',*,*,#10711,.T.);
#15350=ORIENTED_EDGE('',*,*,#10526,.F.);
#15351=ORIENTED_EDGE('',*,*,#10711,.F.);
#15352=ORIENTED_EDGE('',*,*,#10640,.F.);
#15353=ORIENTED_EDGE('',*,*,#10712,.T.);
#15354=ORIENTED_EDGE('',*,*,#10570,.F.);
#15355=ORIENTED_EDGE('',*,*,#10712,.F.);
#15356=ORIENTED_EDGE('',*,*,#10641,.F.);
#15357=ORIENTED_EDGE('',*,*,#10713,.T.);
#15358=ORIENTED_EDGE('',*,*,#10571,.F.);
#15359=ORIENTED_EDGE('',*,*,#10713,.F.);
#15360=ORIENTED_EDGE('',*,*,#10642,.F.);
#15361=ORIENTED_EDGE('',*,*,#10714,.T.);
#15362=ORIENTED_EDGE('',*,*,#10572,.F.);
#15363=ORIENTED_EDGE('',*,*,#10714,.F.);
#18501=CYLINDRICAL_SURFACE('',#20556,0.5);
#18502=CYLINDRICAL_SURFACE('',#20563,0.5);
#18503=CYLINDRICAL_SURFACE('',#20566,0.5);
#18504=CYLINDRICAL_SURFACE('',#20576,0.5);
#18505=CYLINDRICAL_SURFACE('',#20578,0.5);
#18506=CYLINDRICAL_SURFACE('',#20583,0.5);
#18507=CYLINDRICAL_SURFACE('',#20586,0.5);
#18508=CYLINDRICAL_SURFACE('',#20589,0.5);
#18509=CYLINDRICAL_SURFACE('',#20592,0.5);
#18510=CYLINDRICAL_SURFACE('',#20593,0.5);
#18511=CYLINDRICAL_SURFACE('',#20598,0.5);
#18512=CYLINDRICAL_SURFACE('',#20601,0.5);
#18513=CYLINDRICAL_SURFACE('',#20610,0.5);
#18514=CYLINDRICAL_SURFACE('',#20614,0.5);
#18515=CYLINDRICAL_SURFACE('',#20622,0.5);
#18516=CYLINDRICAL_SURFACE('',#20623,0.5);
#18517=CYLINDRICAL_SURFACE('',#20625,0.5);
#18518=CYLINDRICAL_SURFACE('',#20627,0.5);
#18519=CYLINDRICAL_SURFACE('',#20629,0.5);
#18520=CYLINDRICAL_SURFACE('',#20634,0.5);
#18521=CYLINDRICAL_SURFACE('',#20638,0.5);
#18522=CYLINDRICAL_SURFACE('',#20641,0.5);
#18523=CYLINDRICAL_SURFACE('',#20644,0.5);
#18524=CYLINDRICAL_SURFACE('',#20648,0.5);
#18525=CYLINDRICAL_SURFACE('',#20652,0.5);
#18526=CYLINDRICAL_SURFACE('',#20656,0.5);
#18527=CYLINDRICAL_SURFACE('',#20659,0.5);
#18528=CYLINDRICAL_SURFACE('',#20662,0.5);
#18529=CYLINDRICAL_SURFACE('',#20671,0.5);
#18530=CYLINDRICAL_SURFACE('',#20676,0.5);
#18531=CYLINDRICAL_SURFACE('',#20681,0.5);
#18532=CYLINDRICAL_SURFACE('',#20685,0.5);
#18533=CYLINDRICAL_SURFACE('',#20688,0.5);
#18534=CYLINDRICAL_SURFACE('',#20691,0.5);
#18535=CYLINDRICAL_SURFACE('',#20694,0.5);
#18536=CYLINDRICAL_SURFACE('',#20696,0.5);
#18537=CYLINDRICAL_SURFACE('',#20699,0.5);
#18538=CYLINDRICAL_SURFACE('',#20705,0.5);
#18539=CYLINDRICAL_SURFACE('',#20712,0.5);
#18540=CYLINDRICAL_SURFACE('',#20714,0.5);
#18541=CYLINDRICAL_SURFACE('',#20716,0.5);
#18542=CYLINDRICAL_SURFACE('',#20719,0.5);
#18543=CYLINDRICAL_SURFACE('',#20724,0.5);
#18544=CYLINDRICAL_SURFACE('',#20729,0.5);
#18545=CYLINDRICAL_SURFACE('',#20730,0.5);
#18546=CYLINDRICAL_SURFACE('',#20734,0.5);
#18547=CYLINDRICAL_SURFACE('',#20739,0.5);
#18548=CYLINDRICAL_SURFACE('',#20741,0.5);
#18549=CYLINDRICAL_SURFACE('',#20744,0.5);
#18550=CYLINDRICAL_SURFACE('',#20751,0.5);
#18551=CYLINDRICAL_SURFACE('',#20755,0.5);
#18552=CYLINDRICAL_SURFACE('',#20758,0.5);
#18553=CYLINDRICAL_SURFACE('',#20761,0.5);
#18554=CYLINDRICAL_SURFACE('',#20772,0.5);
#18555=CYLINDRICAL_SURFACE('',#20774,0.5);
#18556=CYLINDRICAL_SURFACE('',#20776,0.5);
#18557=CYLINDRICAL_SURFACE('',#20779,0.5);
#18558=CYLINDRICAL_SURFACE('',#20781,0.5);
#18559=CYLINDRICAL_SURFACE('',#20789,0.499999999999999);
#18560=CYLINDRICAL_SURFACE('',#20792,0.5);
#18561=CYLINDRICAL_SURFACE('',#20795,0.5);
#18562=CYLINDRICAL_SURFACE('',#20798,0.499999999999999);
#18563=CYLINDRICAL_SURFACE('',#20801,0.5);
#18564=CYLINDRICAL_SURFACE('',#20803,0.5);
#18565=CYLINDRICAL_SURFACE('',#20806,0.5);
#18566=CYLINDRICAL_SURFACE('',#20811,0.5);
#18567=CYLINDRICAL_SURFACE('',#20817,0.5);
#18568=CYLINDRICAL_SURFACE('',#20821,0.499999999999999);
#18569=CYLINDRICAL_SURFACE('',#20826,0.5);
#18570=CYLINDRICAL_SURFACE('',#20829,0.5);
#18571=CYLINDRICAL_SURFACE('',#20833,0.5);
#18572=CYLINDRICAL_SURFACE('',#20838,0.5);
#18573=CYLINDRICAL_SURFACE('',#20839,0.5);
#18574=CYLINDRICAL_SURFACE('',#20848,44.);
#18575=CYLINDRICAL_SURFACE('',#20860,0.5);
#18576=CYLINDRICAL_SURFACE('',#20866,0.5);
#18577=CYLINDRICAL_SURFACE('',#20893,0.5);
#18578=CYLINDRICAL_SURFACE('',#20895,0.5);
#18579=CYLINDRICAL_SURFACE('',#20900,0.5);
#18580=CYLINDRICAL_SURFACE('',#20910,0.5);
#18581=CYLINDRICAL_SURFACE('',#20916,0.5);
#18582=CYLINDRICAL_SURFACE('',#20927,0.5);
#18583=CYLINDRICAL_SURFACE('',#20930,0.5);
#18584=CYLINDRICAL_SURFACE('',#20938,0.5);
#18585=CYLINDRICAL_SURFACE('',#20941,0.5);
#18586=CYLINDRICAL_SURFACE('',#20942,0.5);
#18587=CYLINDRICAL_SURFACE('',#20965,0.5);
#18588=CYLINDRICAL_SURFACE('',#20969,0.5);
#18589=CYLINDRICAL_SURFACE('',#20974,0.5);
#18590=CYLINDRICAL_SURFACE('',#20979,0.5);
#18591=CYLINDRICAL_SURFACE('',#20983,3.);
#18592=CYLINDRICAL_SURFACE('',#20988,1.25);
#18593=CYLINDRICAL_SURFACE('',#20995,0.5);
#18594=CYLINDRICAL_SURFACE('',#20998,0.5);
#18595=CYLINDRICAL_SURFACE('',#21000,0.5);
#18596=CYLINDRICAL_SURFACE('',#21005,0.499999999999997);
#18597=CYLINDRICAL_SURFACE('',#21009,0.499999999999999);
#18598=CYLINDRICAL_SURFACE('',#21012,0.5);
#18599=CYLINDRICAL_SURFACE('',#21018,0.5);
#18600=CYLINDRICAL_SURFACE('',#21028,1.25);
#18601=CYLINDRICAL_SURFACE('',#21031,0.5);
#18602=CYLINDRICAL_SURFACE('',#21036,0.5);
#18603=CYLINDRICAL_SURFACE('',#21040,0.5);
#18604=CYLINDRICAL_SURFACE('',#21046,0.5);
#18605=CYLINDRICAL_SURFACE('',#21049,0.5);
#18606=CYLINDRICAL_SURFACE('',#21051,0.5);
#18607=CYLINDRICAL_SURFACE('',#21056,0.5);
#18608=CYLINDRICAL_SURFACE('',#21064,44.);
#18609=CYLINDRICAL_SURFACE('',#21085,0.499999999999997);
#18610=CYLINDRICAL_SURFACE('',#21088,0.5);
#18611=CYLINDRICAL_SURFACE('',#21090,0.5);
#18612=CYLINDRICAL_SURFACE('',#21095,0.5);
#18613=CYLINDRICAL_SURFACE('',#21100,1.25);
#18614=CYLINDRICAL_SURFACE('',#21106,1.25);
#18615=CYLINDRICAL_SURFACE('',#21126,3.);
#18616=CYLINDRICAL_SURFACE('',#21132,3.);
#18617=CYLINDRICAL_SURFACE('',#21144,3.);
#18618=CYLINDRICAL_SURFACE('',#21154,3.);
#18619=CYLINDRICAL_SURFACE('',#21162,3.);
#18620=CYLINDRICAL_SURFACE('',#21170,3.);
#18621=CYLINDRICAL_SURFACE('',#21174,0.5);
#18622=CYLINDRICAL_SURFACE('',#21176,0.5);
#18623=CYLINDRICAL_SURFACE('',#21181,0.5);
#18624=CYLINDRICAL_SURFACE('',#21192,44.);
#18625=CYLINDRICAL_SURFACE('',#21216,7.05);
#18626=CYLINDRICAL_SURFACE('',#21232,12.);
#18627=CYLINDRICAL_SURFACE('',#21260,5.);
#18628=CYLINDRICAL_SURFACE('',#21265,5.);
#18629=CYLINDRICAL_SURFACE('',#21270,5.);
#18630=CYLINDRICAL_SURFACE('',#21281,3.);
#18631=CYLINDRICAL_SURFACE('',#21282,3.);
#18632=CYLINDRICAL_SURFACE('',#21283,3.);
#18633=CYLINDRICAL_SURFACE('',#21294,42.4);
#18634=CYLINDRICAL_SURFACE('',#21295,4.5);
#18635=CYLINDRICAL_SURFACE('',#21296,4.5);
#18636=CYLINDRICAL_SURFACE('',#21297,4.5);
#19121=ADVANCED_FACE('',(#1425),#18501,.T.);
#19122=ADVANCED_FACE('',(#1426),#243,.T.);
#19123=ADVANCED_FACE('',(#1427),#18502,.T.);
#19124=ADVANCED_FACE('',(#1428),#18503,.T.);
#19125=ADVANCED_FACE('',(#1429),#244,.T.);
#19126=ADVANCED_FACE('',(#1430),#245,.T.);
#19127=ADVANCED_FACE('',(#1431),#18504,.T.);
#19128=ADVANCED_FACE('',(#1432),#18505,.T.);
#19129=ADVANCED_FACE('',(#1433),#246,.T.);
#19130=ADVANCED_FACE('',(#1434),#18506,.T.);
#19131=ADVANCED_FACE('',(#1435),#893,.T.);
#19132=ADVANCED_FACE('',(#1436),#18507,.T.);
#19133=ADVANCED_FACE('',(#1437),#894,.T.);
#19134=ADVANCED_FACE('',(#1438),#18508,.T.);
#19135=ADVANCED_FACE('',(#1439),#895,.T.);
#19136=ADVANCED_FACE('',(#1440),#18509,.T.);
#19137=ADVANCED_FACE('',(#1441),#18510,.T.);
#19138=ADVANCED_FACE('',(#1442),#247,.T.);
#19139=ADVANCED_FACE('',(#1443),#896,.T.);
#19140=ADVANCED_FACE('',(#1444),#18511,.T.);
#19141=ADVANCED_FACE('',(#1445),#897,.T.);
#19142=ADVANCED_FACE('',(#1446),#18512,.T.);
#19143=ADVANCED_FACE('',(#1447),#248,.T.);
#19144=ADVANCED_FACE('',(#1448),#898,.T.);
#19145=ADVANCED_FACE('',(#1449),#18513,.T.);
#19146=ADVANCED_FACE('',(#1450),#249,.T.);
#19147=ADVANCED_FACE('',(#1451),#18514,.T.);
#19148=ADVANCED_FACE('',(#1452),#899,.T.);
#19149=ADVANCED_FACE('',(#1453),#250,.T.);
#19150=ADVANCED_FACE('',(#1454),#18515,.T.);
#19151=ADVANCED_FACE('',(#1455),#18516,.T.);
#19152=ADVANCED_FACE('',(#1456),#18517,.T.);
#19153=ADVANCED_FACE('',(#1457),#18518,.T.);
#19154=ADVANCED_FACE('',(#1458),#18519,.T.);
#19155=ADVANCED_FACE('',(#1459),#251,.T.);
#19156=ADVANCED_FACE('',(#1460),#900,.T.);
#19157=ADVANCED_FACE('',(#1461),#18520,.T.);
#19158=ADVANCED_FACE('',(#1462),#901,.T.);
#19159=ADVANCED_FACE('',(#1463),#252,.T.);
#19160=ADVANCED_FACE('',(#1464),#18521,.T.);
#19161=ADVANCED_FACE('',(#1465),#902,.T.);
#19162=ADVANCED_FACE('',(#1466),#18522,.T.);
#19163=ADVANCED_FACE('',(#1467),#18523,.T.);
#19164=ADVANCED_FACE('',(#1468),#253,.T.);
#19165=ADVANCED_FACE('',(#1469),#18524,.T.);
#19166=ADVANCED_FACE('',(#1470),#903,.T.);
#19167=ADVANCED_FACE('',(#1471),#904,.T.);
#19168=ADVANCED_FACE('',(#1472),#18525,.T.);
#19169=ADVANCED_FACE('',(#1473),#254,.T.);
#19170=ADVANCED_FACE('',(#1474),#18526,.T.);
#19171=ADVANCED_FACE('',(#1475),#905,.T.);
#19172=ADVANCED_FACE('',(#1476),#18527,.T.);
#19173=ADVANCED_FACE('',(#1477),#18528,.T.);
#19174=ADVANCED_FACE('',(#1478),#255,.T.);
#19175=ADVANCED_FACE('',(#1479),#906,.T.);
#19176=ADVANCED_FACE('',(#1480),#907,.T.);
#19177=ADVANCED_FACE('',(#1481),#18529,.T.);
#19178=ADVANCED_FACE('',(#1482),#256,.T.);
#19179=ADVANCED_FACE('',(#1483),#18530,.T.);
#19180=ADVANCED_FACE('',(#1484),#257,.T.);
#19181=ADVANCED_FACE('',(#1485),#18531,.T.);
#19182=ADVANCED_FACE('',(#1486),#258,.T.);
#19183=ADVANCED_FACE('',(#1487),#18532,.T.);
#19184=ADVANCED_FACE('',(#1488),#908,.T.);
#19185=ADVANCED_FACE('',(#1489),#18533,.T.);
#19186=ADVANCED_FACE('',(#1490),#909,.T.);
#19187=ADVANCED_FACE('',(#1491),#18534,.T.);
#19188=ADVANCED_FACE('',(#1492),#910,.T.);
#19189=ADVANCED_FACE('',(#1493),#18535,.T.);
#19190=ADVANCED_FACE('',(#1494),#18536,.T.);
#19191=ADVANCED_FACE('',(#1495),#18537,.T.);
#19192=ADVANCED_FACE('',(#1496),#259,.T.);
#19193=ADVANCED_FACE('',(#1497),#911,.T.);
#19194=ADVANCED_FACE('',(#1498),#18538,.T.);
#19195=ADVANCED_FACE('',(#1499),#912,.T.);
#19196=ADVANCED_FACE('',(#1500),#260,.T.);
#19197=ADVANCED_FACE('',(#1501),#913,.T.);
#19198=ADVANCED_FACE('',(#1502),#18539,.T.);
#19199=ADVANCED_FACE('',(#1503),#18540,.T.);
#19200=ADVANCED_FACE('',(#1504),#18541,.T.);
#19201=ADVANCED_FACE('',(#1505),#18542,.T.);
#19202=ADVANCED_FACE('',(#1506),#261,.T.);
#19203=ADVANCED_FACE('',(#1507),#18543,.T.);
#19204=ADVANCED_FACE('',(#1508),#262,.T.);
#19205=ADVANCED_FACE('',(#1509),#914,.T.);
#19206=ADVANCED_FACE('',(#1510),#915,.T.);
#19207=ADVANCED_FACE('',(#1511),#18544,.T.);
#19208=ADVANCED_FACE('',(#1512),#18545,.T.);
#19209=ADVANCED_FACE('',(#1513),#263,.T.);
#19210=ADVANCED_FACE('',(#1514),#18546,.T.);
#19211=ADVANCED_FACE('',(#1515),#916,.T.);
#19212=ADVANCED_FACE('',(#1516),#264,.T.);
#19213=ADVANCED_FACE('',(#1517),#18547,.T.);
#19214=ADVANCED_FACE('',(#1518),#18548,.T.);
#19215=ADVANCED_FACE('',(#1519),#18549,.T.);
#19216=ADVANCED_FACE('',(#1520),#265,.T.);
#19217=ADVANCED_FACE('',(#1521),#917,.T.);
#19218=ADVANCED_FACE('',(#1522),#18550,.T.);
#19219=ADVANCED_FACE('',(#1523),#918,.T.);
#19220=ADVANCED_FACE('',(#1524),#18551,.T.);
#19221=ADVANCED_FACE('',(#1525),#18552,.T.);
#19222=ADVANCED_FACE('',(#1526),#18553,.T.);
#19223=ADVANCED_FACE('',(#1527),#266,.T.);
#19224=ADVANCED_FACE('',(#1528),#267,.T.);
#19225=ADVANCED_FACE('',(#1529),#18554,.T.);
#19226=ADVANCED_FACE('',(#1530),#18555,.T.);
#19227=ADVANCED_FACE('',(#1531),#18556,.T.);
#19228=ADVANCED_FACE('',(#1532),#919,.T.);
#19229=ADVANCED_FACE('',(#1533),#18557,.T.);
#19230=ADVANCED_FACE('',(#1534),#18558,.T.);
#19231=ADVANCED_FACE('',(#1535),#268,.T.);
#19232=ADVANCED_FACE('',(#1536),#269,.T.);
#19233=ADVANCED_FACE('',(#1537),#18559,.T.);
#19234=ADVANCED_FACE('',(#1538),#18560,.T.);
#19235=ADVANCED_FACE('',(#1539),#920,.T.);
#19236=ADVANCED_FACE('',(#1540),#18561,.T.);
#19237=ADVANCED_FACE('',(#1541),#921,.T.);
#19238=ADVANCED_FACE('',(#1542),#18562,.T.);
#19239=ADVANCED_FACE('',(#1543),#18563,.T.);
#19240=ADVANCED_FACE('',(#1544),#922,.T.);
#19241=ADVANCED_FACE('',(#1545),#18564,.T.);
#19242=ADVANCED_FACE('',(#1546),#923,.T.);
#19243=ADVANCED_FACE('',(#1547),#18565,.T.);
#19244=ADVANCED_FACE('',(#1548),#270,.T.);
#19245=ADVANCED_FACE('',(#1549),#18566,.T.);
#19246=ADVANCED_FACE('',(#1550),#924,.T.);
#19247=ADVANCED_FACE('',(#1551),#925,.T.);
#19248=ADVANCED_FACE('',(#1552),#926,.T.);
#19249=ADVANCED_FACE('',(#1553),#18567,.T.);
#19250=ADVANCED_FACE('',(#1554),#927,.T.);
#19251=ADVANCED_FACE('',(#1555),#18568,.T.);
#19252=ADVANCED_FACE('',(#1556),#271,.T.);
#19253=ADVANCED_FACE('',(#1557),#18569,.T.);
#19254=ADVANCED_FACE('',(#1558),#272,.T.);
#19255=ADVANCED_FACE('',(#1559),#18570,.T.);
#19256=ADVANCED_FACE('',(#1560),#928,.T.);
#19257=ADVANCED_FACE('',(#1561),#18571,.T.);
#19258=ADVANCED_FACE('',(#1562),#273,.T.);
#19259=ADVANCED_FACE('',(#1563),#18572,.T.);
#19260=ADVANCED_FACE('',(#1564),#18573,.T.);
#19261=ADVANCED_FACE('',(#1565),#274,.T.);
#19262=ADVANCED_FACE('',(#1566),#929,.T.);
#19263=ADVANCED_FACE('',(#1567),#95,.T.);
#19264=ADVANCED_FACE('',(#1568),#18574,.T.);
#19265=ADVANCED_FACE('',(#1569,#1083),#930,.F.);
#19266=ADVANCED_FACE('',(#1570),#18575,.T.);
#19267=ADVANCED_FACE('',(#1571),#96,.T.);
#19268=ADVANCED_FACE('',(#1572),#18576,.T.);
#19269=ADVANCED_FACE('',(#1573),#275,.T.);
#19270=ADVANCED_FACE('',(#1574),#276,.T.);
#19271=ADVANCED_FACE('',(#1575),#838,.F.);
#19272=ADVANCED_FACE('',(#1576,#1084),#931,.T.);
#19273=ADVANCED_FACE('',(#1577),#97,.T.);
#19274=ADVANCED_FACE('',(#1578),#414,.T.);
#19275=ADVANCED_FACE('',(#1579),#98,.T.);
#19276=ADVANCED_FACE('',(#1580),#18577,.T.);
#19277=ADVANCED_FACE('',(#1581),#18578,.T.);
#19278=ADVANCED_FACE('',(#1582),#99,.T.);
#19279=ADVANCED_FACE('',(#1583),#18579,.T.);
#19280=ADVANCED_FACE('',(#1584),#100,.T.);
#19281=ADVANCED_FACE('',(#1585),#101,.T.);
#19282=ADVANCED_FACE('',(#1586),#932,.F.);
#19283=ADVANCED_FACE('',(#1587),#415,.T.);
#19284=ADVANCED_FACE('',(#1588),#18580,.T.);
#19285=ADVANCED_FACE('',(#1589),#839,.F.);
#19286=ADVANCED_FACE('',(#1590),#277,.T.);
#19287=ADVANCED_FACE('',(#1591),#18581,.T.);
#19288=ADVANCED_FACE('',(#1592),#278,.T.);
#19289=ADVANCED_FACE('',(#1593),#933,.F.);
#19290=ADVANCED_FACE('',(#1594),#416,.T.);
#19291=ADVANCED_FACE('',(#1595),#102,.T.);
#19292=ADVANCED_FACE('',(#1596),#18582,.T.);
#19293=ADVANCED_FACE('',(#1597),#934,.F.);
#19294=ADVANCED_FACE('',(#1598),#103,.T.);
#19295=ADVANCED_FACE('',(#1599),#18583,.T.);
#19296=ADVANCED_FACE('',(#1600),#935,.F.);
#19297=ADVANCED_FACE('',(#1601),#840,.F.);
#19298=ADVANCED_FACE('',(#1602),#279,.T.);
#19299=ADVANCED_FACE('',(#1603),#280,.T.);
#19300=ADVANCED_FACE('',(#1604),#18584,.T.);
#19301=ADVANCED_FACE('',(#1605),#936,.F.);
#19302=ADVANCED_FACE('',(#1606),#18585,.T.);
#19303=ADVANCED_FACE('',(#1607),#18586,.T.);
#19304=ADVANCED_FACE('',(#1608),#841,.F.);
#19305=ADVANCED_FACE('',(#1609),#281,.T.);
#19306=ADVANCED_FACE('',(#1610),#282,.T.);
#19307=ADVANCED_FACE('',(#1611),#104,.T.);
#19308=ADVANCED_FACE('',(#1612),#417,.T.);
#19309=ADVANCED_FACE('',(#1613),#105,.T.);
#19310=ADVANCED_FACE('',(#1614,#1085),#937,.F.);
#19311=ADVANCED_FACE('',(#1615),#283,.T.);
#19312=ADVANCED_FACE('',(#1616),#842,.F.);
#19313=ADVANCED_FACE('',(#1617),#18587,.T.);
#19314=ADVANCED_FACE('',(#1618),#106,.T.);
#19315=ADVANCED_FACE('',(#1619),#18588,.T.);
#19316=ADVANCED_FACE('',(#1620),#107,.T.);
#19317=ADVANCED_FACE('',(#1621),#18589,.T.);
#19318=ADVANCED_FACE('',(#1622),#284,.T.);
#19319=ADVANCED_FACE('',(#1623),#938,.F.);
#19320=ADVANCED_FACE('',(#1624),#939,.F.);
#19321=ADVANCED_FACE('',(#1625),#18590,.T.);
#19322=ADVANCED_FACE('',(#1626),#108,.T.);
#19323=ADVANCED_FACE('',(#1627),#18591,.F.);
#19324=ADVANCED_FACE('',(#1628),#109,.T.);
#19325=ADVANCED_FACE('',(#1629),#18592,.F.);
#19326=ADVANCED_FACE('',(#1630),#285,.T.);
#19327=ADVANCED_FACE('',(#1631),#18593,.T.);
#19328=ADVANCED_FACE('',(#1632),#940,.T.);
#19329=ADVANCED_FACE('',(#1633),#18594,.T.);
#19330=ADVANCED_FACE('',(#1634),#18595,.T.);
#19331=ADVANCED_FACE('',(#1635),#18596,.T.);
#19332=ADVANCED_FACE('',(#1636),#941,.T.);
#19333=ADVANCED_FACE('',(#1637),#18597,.T.);
#19334=ADVANCED_FACE('',(#1638),#18598,.T.);
#19335=ADVANCED_FACE('',(#1639),#942,.T.);
#19336=ADVANCED_FACE('',(#1640),#943,.T.);
#19337=ADVANCED_FACE('',(#1641),#18599,.T.);
#19338=ADVANCED_FACE('',(#1642),#110,.T.);
#19339=ADVANCED_FACE('',(#1643,#1086),#944,.F.);
#19340=ADVANCED_FACE('',(#1644),#111,.T.);
#19341=ADVANCED_FACE('',(#1645),#18600,.F.);
#19342=ADVANCED_FACE('',(#1646),#18601,.T.);
#19343=ADVANCED_FACE('',(#1647),#286,.T.);
#19344=ADVANCED_FACE('',(#1648),#18602,.T.);
#19345=ADVANCED_FACE('',(#1649),#287,.T.);
#19346=ADVANCED_FACE('',(#1650),#18603,.T.);
#19347=ADVANCED_FACE('',(#1651),#288,.T.);
#19348=ADVANCED_FACE('',(#1652),#18604,.T.);
#19349=ADVANCED_FACE('',(#1653),#945,.T.);
#19350=ADVANCED_FACE('',(#1654),#18605,.T.);
#19351=ADVANCED_FACE('',(#1655),#18606,.T.);
#19352=ADVANCED_FACE('',(#1656),#289,.T.);
#19353=ADVANCED_FACE('',(#1657),#946,.T.);
#19354=ADVANCED_FACE('',(#1658),#18607,.T.);
#19355=ADVANCED_FACE('',(#1659),#947,.T.);
#19356=ADVANCED_FACE('',(#1660),#112,.T.);
#19357=ADVANCED_FACE('',(#1661),#18608,.T.);
#19358=ADVANCED_FACE('',(#1662,#1087),#948,.F.);
#19359=ADVANCED_FACE('',(#1663),#113,.T.);
#19360=ADVANCED_FACE('',(#1664),#418,.T.);
#19361=ADVANCED_FACE('',(#1665),#114,.T.);
#19362=ADVANCED_FACE('',(#1666,#1088),#949,.F.);
#19363=ADVANCED_FACE('',(#1667),#115,.T.);
#19364=ADVANCED_FACE('',(#1668,#1089),#950,.F.);
#19365=ADVANCED_FACE('',(#1669),#18609,.T.);
#19366=ADVANCED_FACE('',(#1670),#18610,.T.);
#19367=ADVANCED_FACE('',(#1671),#951,.T.);
#19368=ADVANCED_FACE('',(#1672),#18611,.T.);
#19369=ADVANCED_FACE('',(#1673),#290,.T.);
#19370=ADVANCED_FACE('',(#1674),#952,.T.);
#19371=ADVANCED_FACE('',(#1675),#18612,.T.);
#19372=ADVANCED_FACE('',(#1676),#116,.T.);
#19373=ADVANCED_FACE('',(#1677),#18613,.F.);
#19374=ADVANCED_FACE('',(#1678),#117,.T.);
#19375=ADVANCED_FACE('',(#1679),#18614,.F.);
#19376=ADVANCED_FACE('',(#1680),#118,.T.);
#19377=ADVANCED_FACE('',(#1681,#1090,#1091,#1092,#1093,#1094,#1095,#1096,
#1097,#1098,#1099,#1100),#953,.T.);
#19378=ADVANCED_FACE('',(#1682),#18615,.F.);
#19379=ADVANCED_FACE('',(#1683),#119,.T.);
#19380=ADVANCED_FACE('',(#1684),#18616,.F.);
#19381=ADVANCED_FACE('',(#1685),#120,.T.);
#19382=ADVANCED_FACE('',(#1686),#121,.T.);
#19383=ADVANCED_FACE('',(#1687),#122,.T.);
#19384=ADVANCED_FACE('',(#1688),#123,.T.);
#19385=ADVANCED_FACE('',(#1689),#18617,.F.);
#19386=ADVANCED_FACE('',(#1690),#124,.T.);
#19387=ADVANCED_FACE('',(#1691),#125,.T.);
#19388=ADVANCED_FACE('',(#1692),#126,.T.);
#19389=ADVANCED_FACE('',(#1693),#18618,.F.);
#19390=ADVANCED_FACE('',(#1694,#1101),#954,.T.);
#19391=ADVANCED_FACE('',(#1695),#127,.T.);
#19392=ADVANCED_FACE('',(#1696),#18619,.F.);
#19393=ADVANCED_FACE('',(#1697,#1102),#955,.T.);
#19394=ADVANCED_FACE('',(#1698),#128,.T.);
#19395=ADVANCED_FACE('',(#1699),#18620,.F.);
#19396=ADVANCED_FACE('',(#1700,#1103),#956,.T.);
#19397=ADVANCED_FACE('',(#1701),#18621,.T.);
#19398=ADVANCED_FACE('',(#1702),#18622,.T.);
#19399=ADVANCED_FACE('',(#1703),#291,.T.);
#19400=ADVANCED_FACE('',(#1704),#957,.T.);
#19401=ADVANCED_FACE('',(#1705),#18623,.T.);
#19402=ADVANCED_FACE('',(#1706),#129,.T.);
#19403=ADVANCED_FACE('',(#1707),#419,.T.);
#19404=ADVANCED_FACE('',(#1708),#18624,.T.);
#19405=ADVANCED_FACE('',(#1709),#130,.T.);
#19406=ADVANCED_FACE('',(#1710,#1104,#1105,#1106,#1107,#1108,#1109,#1110),
#958,.T.);
#19407=ADVANCED_FACE('',(#1711),#131,.T.);
#19408=ADVANCED_FACE('',(#1712),#132,.T.);
#19409=ADVANCED_FACE('',(#1713),#133,.T.);
#19410=ADVANCED_FACE('',(#1714),#134,.T.);
#19411=ADVANCED_FACE('',(#1715),#18625,.F.);
#19412=ADVANCED_FACE('',(#1716),#135,.T.);
#19413=ADVANCED_FACE('',(#1717),#420,.F.);
#19414=ADVANCED_FACE('',(#1718),#136,.T.);
#19415=ADVANCED_FACE('',(#1719),#137,.T.);
#19416=ADVANCED_FACE('',(#1720),#18626,.F.);
#19417=ADVANCED_FACE('',(#1721),#138,.T.);
#19418=ADVANCED_FACE('',(#1722),#421,.T.);
#19419=ADVANCED_FACE('',(#1723),#139,.T.);
#19420=ADVANCED_FACE('',(#1724),#140,.T.);
#19421=ADVANCED_FACE('',(#1725,#1111,#1112,#1113,#1114),#959,.T.);
#19422=ADVANCED_FACE('',(#1726),#18627,.F.);
#19423=ADVANCED_FACE('',(#1727),#141,.T.);
#19424=ADVANCED_FACE('',(#1728),#18628,.F.);
#19425=ADVANCED_FACE('',(#1729),#142,.T.);
#19426=ADVANCED_FACE('',(#1730),#18629,.F.);
#19427=ADVANCED_FACE('',(#1731),#143,.T.);
#19428=ADVANCED_FACE('',(#1732),#422,.F.);
#19429=ADVANCED_FACE('',(#1733),#144,.T.);
#19430=ADVANCED_FACE('',(#1734),#960,.F.);
#19431=ADVANCED_FACE('',(#1735),#18630,.F.);
#19432=ADVANCED_FACE('',(#1736),#18631,.F.);
#19433=ADVANCED_FACE('',(#1737),#18632,.F.);
#19434=ADVANCED_FACE('',(#1738),#961,.T.);
#19435=ADVANCED_FACE('',(#1739),#962,.T.);
#19436=ADVANCED_FACE('',(#1740),#963,.T.);
#19437=ADVANCED_FACE('',(#1741),#964,.T.);
#19438=ADVANCED_FACE('',(#1742),#965,.T.);
#19439=ADVANCED_FACE('',(#1743),#966,.T.);
#19440=ADVANCED_FACE('',(#1744),#967,.T.);
#19441=ADVANCED_FACE('',(#1745),#968,.T.);
#19442=ADVANCED_FACE('',(#1746),#969,.T.);
#19443=ADVANCED_FACE('',(#1747),#970,.T.);
#19444=ADVANCED_FACE('',(#1748),#18633,.T.);
#19445=ADVANCED_FACE('',(#1749),#18634,.T.);
#19446=ADVANCED_FACE('',(#1750),#18635,.T.);
#19447=ADVANCED_FACE('',(#1751),#18636,.T.);
#20009=CLOSED_SHELL('',(#19121,#19122,#19123,#19124,#19125,#19126,#19127,
#19128,#19129,#19130,#19131,#19132,#19133,#19134,#19135,#19136,#19137,#19138,
#19139,#19140,#19141,#19142,#19143,#19144,#19145,#19146,#19147,#19148,#19149,
#19150,#19151,#19152,#19153,#19154,#19155,#19156,#19157,#19158,#19159,#19160,
#19161,#19162,#19163,#19164,#19165,#19166,#19167,#19168,#19169,#19170,#19171,
#19172,#19173,#19174,#19175,#19176,#19177,#19178,#19179,#19180,#19181,#19182,
#19183,#19184,#19185,#19186,#19187,#19188,#19189,#19190,#19191,#19192,#19193,
#19194,#19195,#19196,#19197,#19198,#19199,#19200,#19201,#19202,#19203,#19204,
#19205,#19206,#19207,#19208,#19209,#19210,#19211,#19212,#19213,#19214,#19215,
#19216,#19217,#19218,#19219,#19220,#19221,#19222,#19223,#19224,#19225,#19226,
#19227,#19228,#19229,#19230,#19231,#19232,#19233,#19234,#19235,#19236,#19237,
#19238,#19239,#19240,#19241,#19242,#19243,#19244,#19245,#19246,#19247,#19248,
#19249,#19250,#19251,#19252,#19253,#19254,#19255,#19256,#19257,#19258,#19259,
#19260,#19261,#19262,#19263,#19264,#19265,#19266,#19267,#19268,#19269,#19270,
#19271,#19272,#19273,#19274,#19275,#19276,#19277,#19278,#19279,#19280,#19281,
#19282,#19283,#19284,#19285,#19286,#19287,#19288,#19289,#19290,#19291,#19292,
#19293,#19294,#19295,#19296,#19297,#19298,#19299,#19300,#19301,#19302,#19303,
#19304,#19305,#19306,#19307,#19308,#19309,#19310,#19311,#19312,#19313,#19314,
#19315,#19316,#19317,#19318,#19319,#19320,#19321,#19322,#19323,#19324,#19325,
#19326,#19327,#19328,#19329,#19330,#19331,#19332,#19333,#19334,#19335,#19336,
#19337,#19338,#19339,#19340,#19341,#19342,#19343,#19344,#19345,#19346,#19347,
#19348,#19349,#19350,#19351,#19352,#19353,#19354,#19355,#19356,#19357,#19358,
#19359,#19360,#19361,#19362,#19363,#19364,#19365,#19366,#19367,#19368,#19369,
#19370,#19371,#19372,#19373,#19374,#19375,#19376,#19377,#19378,#19379,#19380,
#19381,#19382,#19383,#19384,#19385,#19386,#19387,#19388,#19389,#19390,#19391,
#19392,#19393,#19394,#19395,#19396,#19397,#19398,#19399,#19400,#19401,#19402,
#19403,#19404,#19405,#19406,#19407,#19408,#19409,#19410,#19411,#19412,#19413,
#19414,#19415,#19416,#19417,#19418,#19419,#19420,#19421,#19422,#19423,#19424,
#19425,#19426,#19427,#19428,#19429,#19430,#19431,#19432,#19433,#19434,#19435,
#19436,#19437,#19438,#19439,#19440,#19441,#19442,#19443,#19444,#19445,#19446,
#19447));
#20555=AXIS2_PLACEMENT_3D('',#47239,#23433,#23434);
#20556=AXIS2_PLACEMENT_3D('',#47240,#23435,#23436);
#20557=AXIS2_PLACEMENT_3D('',#47243,#23437,#23438);
#20558=AXIS2_PLACEMENT_3D('',#47247,#23440,#23441);
#20559=AXIS2_PLACEMENT_3D('',#47249,#23443,#23444);
#20560=AXIS2_PLACEMENT_3D('',#47252,#23445,#23446);
#20561=AXIS2_PLACEMENT_3D('',#47253,#23447,#23448);
#20562=AXIS2_PLACEMENT_3D('',#47254,#23449,#23450);
#20563=AXIS2_PLACEMENT_3D('',#47255,#23451,#23452);
#20564=AXIS2_PLACEMENT_3D('',#47258,#23453,#23454);
#20565=AXIS2_PLACEMENT_3D('',#47261,#23456,#23457);
#20566=AXIS2_PLACEMENT_3D('',#47263,#23459,#23460);
#20567=AXIS2_PLACEMENT_3D('',#47266,#23461,#23462);
#20568=AXIS2_PLACEMENT_3D('',#47269,#23464,#23465);
#20569=AXIS2_PLACEMENT_3D('',#47271,#23467,#23468);
#20570=AXIS2_PLACEMENT_3D('',#47272,#23469,#23470);
#20571=AXIS2_PLACEMENT_3D('',#47273,#23471,#23472);
#20572=AXIS2_PLACEMENT_3D('',#47276,#23473,#23474);
#20573=AXIS2_PLACEMENT_3D('',#47278,#23475,#23476);
#20574=AXIS2_PLACEMENT_3D('',#47280,#23477,#23478);
#20575=AXIS2_PLACEMENT_3D('',#47281,#23479,#23480);
#20576=AXIS2_PLACEMENT_3D('',#47282,#23481,#23482);
#20577=AXIS2_PLACEMENT_3D('',#47285,#23483,#23484);
#20578=AXIS2_PLACEMENT_3D('',#47288,#23487,#23488);
#20579=AXIS2_PLACEMENT_3D('',#47290,#23489,#23490);
#20580=AXIS2_PLACEMENT_3D('',#47293,#23492,#23493);
#20581=AXIS2_PLACEMENT_3D('',#47295,#23495,#23496);
#20582=AXIS2_PLACEMENT_3D('',#47296,#23497,#23498);
#20583=AXIS2_PLACEMENT_3D('',#47297,#23499,#23500);
#20584=AXIS2_PLACEMENT_3D('',#47301,#23502,#23503);
#20585=AXIS2_PLACEMENT_3D('',#47303,#23505,#23506);
#20586=AXIS2_PLACEMENT_3D('',#47305,#23508,#23509);
#20587=AXIS2_PLACEMENT_3D('',#47308,#23511,#23512);
#20588=AXIS2_PLACEMENT_3D('',#47309,#23513,#23514);
#20589=AXIS2_PLACEMENT_3D('',#47313,#23517,#23518);
#20590=AXIS2_PLACEMENT_3D('',#47316,#23520,#23521);
#20591=AXIS2_PLACEMENT_3D('',#47317,#23522,#23523);
#20592=AXIS2_PLACEMENT_3D('',#47319,#23525,#23526);
#20593=AXIS2_PLACEMENT_3D('',#47322,#23529,#23530);
#20594=AXIS2_PLACEMENT_3D('',#47325,#23532,#23533);
#20595=AXIS2_PLACEMENT_3D('',#47326,#23534,#23535);
#20596=AXIS2_PLACEMENT_3D('',#47327,#23536,#23537);
#20597=AXIS2_PLACEMENT_3D('',#47328,#23538,#23539);
#20598=AXIS2_PLACEMENT_3D('',#47330,#23541,#23542);
#20599=AXIS2_PLACEMENT_3D('',#47331,#23543,#23544);
#20600=AXIS2_PLACEMENT_3D('',#47332,#23545,#23546);
#20601=AXIS2_PLACEMENT_3D('',#47334,#23548,#23549);
#20602=AXIS2_PLACEMENT_3D('',#47344,#23550,#23551);
#20603=AXIS2_PLACEMENT_3D('',#47346,#23552,#23553);
#20604=AXIS2_PLACEMENT_3D('',#47349,#23555,#23556);
#20605=AXIS2_PLACEMENT_3D('',#47351,#23558,#23559);
#20606=AXIS2_PLACEMENT_3D('',#47352,#23560,#23561);
#20607=AXIS2_PLACEMENT_3D('',#47353,#23562,#23563);
#20608=AXIS2_PLACEMENT_3D('',#47357,#23565,#23566);
#20609=AXIS2_PLACEMENT_3D('',#47360,#23568,#23569);
#20610=AXIS2_PLACEMENT_3D('',#47361,#23570,#23571);
#20611=AXIS2_PLACEMENT_3D('',#47364,#23573,#23574);
#20612=AXIS2_PLACEMENT_3D('',#47365,#23575,#23576);
#20613=AXIS2_PLACEMENT_3D('',#47366,#23577,#23578);
#20614=AXIS2_PLACEMENT_3D('',#47367,#23579,#23580);
#20615=AXIS2_PLACEMENT_3D('',#47371,#23582,#23583);
#20616=AXIS2_PLACEMENT_3D('',#47373,#23585,#23586);
#20617=AXIS2_PLACEMENT_3D('',#47379,#23590,#23591);
#20618=AXIS2_PLACEMENT_3D('',#47382,#23592,#23593);
#20619=AXIS2_PLACEMENT_3D('',#47383,#23594,#23595);
#20620=AXIS2_PLACEMENT_3D('',#47385,#23596,#23597);
#20621=AXIS2_PLACEMENT_3D('',#47386,#23598,#23599);
#20622=AXIS2_PLACEMENT_3D('',#47387,#23600,#23601);
#20623=AXIS2_PLACEMENT_3D('',#47389,#23603,#23604);
#20624=AXIS2_PLACEMENT_3D('',#47404,#23606,#23607);
#20625=AXIS2_PLACEMENT_3D('',#47405,#23608,#23609);
#20626=AXIS2_PLACEMENT_3D('',#47409,#23611,#23612);
#20627=AXIS2_PLACEMENT_3D('',#47411,#23614,#23615);
#20628=AXIS2_PLACEMENT_3D('',#47415,#23617,#23618);
#20629=AXIS2_PLACEMENT_3D('',#47417,#23620,#23621);
#20630=AXIS2_PLACEMENT_3D('',#47419,#23622,#23623);
#20631=AXIS2_PLACEMENT_3D('',#47422,#23626,#23627);
#20632=AXIS2_PLACEMENT_3D('',#47423,#23628,#23629);
#20633=AXIS2_PLACEMENT_3D('',#47424,#23630,#23631);
#20634=AXIS2_PLACEMENT_3D('',#47428,#23634,#23635);
#20635=AXIS2_PLACEMENT_3D('',#47431,#23637,#23638);
#20636=AXIS2_PLACEMENT_3D('',#47432,#23639,#23640);
#20637=AXIS2_PLACEMENT_3D('',#47434,#23642,#23643);
#20638=AXIS2_PLACEMENT_3D('',#47435,#23644,#23645);
#20639=AXIS2_PLACEMENT_3D('',#47439,#23647,#23648);
#20640=AXIS2_PLACEMENT_3D('',#47441,#23650,#23651);
#20641=AXIS2_PLACEMENT_3D('',#47449,#23656,#23657);
#20642=AXIS2_PLACEMENT_3D('',#47451,#23658,#23659);
#20643=AXIS2_PLACEMENT_3D('',#47453,#23660,#23661);
#20644=AXIS2_PLACEMENT_3D('',#47460,#23662,#23663);
#20645=AXIS2_PLACEMENT_3D('',#47462,#23664,#23665);
#20646=AXIS2_PLACEMENT_3D('',#47464,#23667,#23668);
#20647=AXIS2_PLACEMENT_3D('',#47465,#23669,#23670);
#20648=AXIS2_PLACEMENT_3D('',#47466,#23671,#23672);
#20649=AXIS2_PLACEMENT_3D('',#47468,#23673,#23674);
#20650=AXIS2_PLACEMENT_3D('',#47470,#23676,#23677);
#20651=AXIS2_PLACEMENT_3D('',#47484,#23680,#23681);
#20652=AXIS2_PLACEMENT_3D('',#47485,#23682,#23683);
#20653=AXIS2_PLACEMENT_3D('',#47486,#23684,#23685);
#20654=AXIS2_PLACEMENT_3D('',#47488,#23687,#23688);
#20655=AXIS2_PLACEMENT_3D('',#47489,#23689,#23690);
#20656=AXIS2_PLACEMENT_3D('',#47490,#23691,#23692);
#20657=AXIS2_PLACEMENT_3D('',#47492,#23693,#23694);
#20658=AXIS2_PLACEMENT_3D('',#47504,#23695,#23696);
#20659=AXIS2_PLACEMENT_3D('',#47505,#23697,#23698);
#20660=AXIS2_PLACEMENT_3D('',#47508,#23699,#23700);
#20661=AXIS2_PLACEMENT_3D('',#47512,#23702,#23703);
#20662=AXIS2_PLACEMENT_3D('',#47514,#23705,#23706);
#20663=AXIS2_PLACEMENT_3D('',#47516,#23707,#23708);
#20664=AXIS2_PLACEMENT_3D('',#47520,#23710,#23711);
#20665=AXIS2_PLACEMENT_3D('',#47522,#23713,#23714);
#20666=AXIS2_PLACEMENT_3D('',#47525,#23715,#23716);
#20667=AXIS2_PLACEMENT_3D('',#47526,#23717,#23718);
#20668=AXIS2_PLACEMENT_3D('',#47527,#23719,#23720);
#20669=AXIS2_PLACEMENT_3D('',#47528,#23721,#23722);
#20670=AXIS2_PLACEMENT_3D('',#47534,#23726,#23727);
#20671=AXIS2_PLACEMENT_3D('',#47540,#23731,#23732);
#20672=AXIS2_PLACEMENT_3D('',#47542,#23733,#23734);
#20673=AXIS2_PLACEMENT_3D('',#47544,#23735,#23736);
#20674=AXIS2_PLACEMENT_3D('',#47546,#23738,#23739);
#20675=AXIS2_PLACEMENT_3D('',#47547,#23740,#23741);
#20676=AXIS2_PLACEMENT_3D('',#47548,#23742,#23743);
#20677=AXIS2_PLACEMENT_3D('',#47550,#23744,#23745);
#20678=AXIS2_PLACEMENT_3D('',#47553,#23747,#23748);
#20679=AXIS2_PLACEMENT_3D('',#47554,#23749,#23750);
#20680=AXIS2_PLACEMENT_3D('',#47555,#23751,#23752);
#20681=AXIS2_PLACEMENT_3D('',#47556,#23753,#23754);
#20682=AXIS2_PLACEMENT_3D('',#47559,#23756,#23757);
#20683=AXIS2_PLACEMENT_3D('',#47560,#23758,#23759);
#20684=AXIS2_PLACEMENT_3D('',#47561,#23760,#23761);
#20685=AXIS2_PLACEMENT_3D('',#47562,#23762,#23763);
#20686=AXIS2_PLACEMENT_3D('',#47565,#23765,#23766);
#20687=AXIS2_PLACEMENT_3D('',#47566,#23767,#23768);
#20688=AXIS2_PLACEMENT_3D('',#47570,#23771,#23772);
#20689=AXIS2_PLACEMENT_3D('',#47573,#23774,#23775);
#20690=AXIS2_PLACEMENT_3D('',#47574,#23776,#23777);
#20691=AXIS2_PLACEMENT_3D('',#47578,#23780,#23781);
#20692=AXIS2_PLACEMENT_3D('',#47581,#23783,#23784);
#20693=AXIS2_PLACEMENT_3D('',#47582,#23785,#23786);
#20694=AXIS2_PLACEMENT_3D('',#47586,#23789,#23790);
#20695=AXIS2_PLACEMENT_3D('',#47589,#23792,#23793);
#20696=AXIS2_PLACEMENT_3D('',#47590,#23794,#23795);
#20697=AXIS2_PLACEMENT_3D('',#47593,#23796,#23797);
#20698=AXIS2_PLACEMENT_3D('',#47597,#23799,#23800);
#20699=AXIS2_PLACEMENT_3D('',#47599,#23802,#23803);
#20700=AXIS2_PLACEMENT_3D('',#47615,#23805,#23806);
#20701=AXIS2_PLACEMENT_3D('',#47618,#23808,#23809);
#20702=AXIS2_PLACEMENT_3D('',#47619,#23810,#23811);
#20703=AXIS2_PLACEMENT_3D('',#47620,#23812,#23813);
#20704=AXIS2_PLACEMENT_3D('',#47621,#23814,#23815);
#20705=AXIS2_PLACEMENT_3D('',#47627,#23819,#23820);
#20706=AXIS2_PLACEMENT_3D('',#47630,#23822,#23823);
#20707=AXIS2_PLACEMENT_3D('',#47631,#23824,#23825);
#20708=AXIS2_PLACEMENT_3D('',#47645,#23828,#23829);
#20709=AXIS2_PLACEMENT_3D('',#47647,#23830,#23831);
#20710=AXIS2_PLACEMENT_3D('',#47648,#23832,#23833);
#20711=AXIS2_PLACEMENT_3D('',#47649,#23834,#23835);
#20712=AXIS2_PLACEMENT_3D('',#47652,#23838,#23839);
#20713=AXIS2_PLACEMENT_3D('',#47666,#23840,#23841);
#20714=AXIS2_PLACEMENT_3D('',#47668,#23843,#23844);
#20715=AXIS2_PLACEMENT_3D('',#47671,#23846,#23847);
#20716=AXIS2_PLACEMENT_3D('',#47672,#23848,#23849);
#20717=AXIS2_PLACEMENT_3D('',#47674,#23850,#23851);
#20718=AXIS2_PLACEMENT_3D('',#47676,#23852,#23853);
#20719=AXIS2_PLACEMENT_3D('',#47678,#23855,#23856);
#20720=AXIS2_PLACEMENT_3D('',#47680,#23857,#23858);
#20721=AXIS2_PLACEMENT_3D('',#47681,#23859,#23860);
#20722=AXIS2_PLACEMENT_3D('',#47683,#23862,#23863);
#20723=AXIS2_PLACEMENT_3D('',#47684,#23864,#23865);
#20724=AXIS2_PLACEMENT_3D('',#47685,#23866,#23867);
#20725=AXIS2_PLACEMENT_3D('',#47687,#23868,#23869);
#20726=AXIS2_PLACEMENT_3D('',#47689,#23871,#23872);
#20727=AXIS2_PLACEMENT_3D('',#47690,#23873,#23874);
#20728=AXIS2_PLACEMENT_3D('',#47692,#23876,#23877);
#20729=AXIS2_PLACEMENT_3D('',#47695,#23880,#23881);
#20730=AXIS2_PLACEMENT_3D('',#47696,#23882,#23883);
#20731=AXIS2_PLACEMENT_3D('',#47698,#23884,#23885);
#20732=AXIS2_PLACEMENT_3D('',#47700,#23887,#23888);
#20733=AXIS2_PLACEMENT_3D('',#47701,#23889,#23890);
#20734=AXIS2_PLACEMENT_3D('',#47702,#23891,#23892);
#20735=AXIS2_PLACEMENT_3D('',#47705,#23894,#23895);
#20736=AXIS2_PLACEMENT_3D('',#47706,#23896,#23897);
#20737=AXIS2_PLACEMENT_3D('',#47710,#23900,#23901);
#20738=AXIS2_PLACEMENT_3D('',#47711,#23902,#23903);
#20739=AXIS2_PLACEMENT_3D('',#47712,#23904,#23905);
#20740=AXIS2_PLACEMENT_3D('',#47713,#23906,#23907);
#20741=AXIS2_PLACEMENT_3D('',#47714,#23908,#23909);
#20742=AXIS2_PLACEMENT_3D('',#47728,#23911,#23912);
#20743=AXIS2_PLACEMENT_3D('',#47731,#23914,#23915);
#20744=AXIS2_PLACEMENT_3D('',#47732,#23916,#23917);
#20745=AXIS2_PLACEMENT_3D('',#47735,#23918,#23919);
#20746=AXIS2_PLACEMENT_3D('',#47738,#23921,#23922);
#20747=AXIS2_PLACEMENT_3D('',#47741,#23924,#23925);
#20748=AXIS2_PLACEMENT_3D('',#47742,#23926,#23927);
#20749=AXIS2_PLACEMENT_3D('',#47743,#23928,#23929);
#20750=AXIS2_PLACEMENT_3D('',#47744,#23930,#23931);
#20751=AXIS2_PLACEMENT_3D('',#47750,#23935,#23936);
#20752=AXIS2_PLACEMENT_3D('',#47754,#23938,#23939);
#20753=AXIS2_PLACEMENT_3D('',#47755,#23940,#23941);
#20754=AXIS2_PLACEMENT_3D('',#47756,#23942,#23943);
#20755=AXIS2_PLACEMENT_3D('',#47760,#23946,#23947);
#20756=AXIS2_PLACEMENT_3D('',#47762,#23948,#23949);
#20757=AXIS2_PLACEMENT_3D('',#47765,#23951,#23952);
#20758=AXIS2_PLACEMENT_3D('',#47766,#23953,#23954);
#20759=AXIS2_PLACEMENT_3D('',#47768,#23955,#23956);
#20760=AXIS2_PLACEMENT_3D('',#47772,#23958,#23959);
#20761=AXIS2_PLACEMENT_3D('',#47774,#23961,#23962);
#20762=AXIS2_PLACEMENT_3D('',#47777,#23963,#23964);
#20763=AXIS2_PLACEMENT_3D('',#47781,#23966,#23967);
#20764=AXIS2_PLACEMENT_3D('',#47783,#23969,#23970);
#20765=AXIS2_PLACEMENT_3D('',#47786,#23971,#23972);
#20766=AXIS2_PLACEMENT_3D('',#47787,#23973,#23974);
#20767=AXIS2_PLACEMENT_3D('',#47788,#23975,#23976);
#20768=AXIS2_PLACEMENT_3D('',#47789,#23977,#23978);
#20769=AXIS2_PLACEMENT_3D('',#47792,#23979,#23980);
#20770=AXIS2_PLACEMENT_3D('',#47793,#23981,#23982);
#20771=AXIS2_PLACEMENT_3D('',#47794,#23983,#23984);
#20772=AXIS2_PLACEMENT_3D('',#47795,#23985,#23986);
#20773=AXIS2_PLACEMENT_3D('',#47799,#23988,#23989);
#20774=AXIS2_PLACEMENT_3D('',#47801,#23991,#23992);
#20775=AXIS2_PLACEMENT_3D('',#47805,#23994,#23995);
#20776=AXIS2_PLACEMENT_3D('',#47807,#23997,#23998);
#20777=AXIS2_PLACEMENT_3D('',#47811,#24000,#24001);
#20778=AXIS2_PLACEMENT_3D('',#47813,#24003,#24004);
#20779=AXIS2_PLACEMENT_3D('',#47817,#24007,#24008);
#20780=AXIS2_PLACEMENT_3D('',#47820,#24010,#24011);
#20781=AXIS2_PLACEMENT_3D('',#47821,#24012,#24013);
#20782=AXIS2_PLACEMENT_3D('',#47824,#24014,#24015);
#20783=AXIS2_PLACEMENT_3D('',#47827,#24017,#24018);
#20784=AXIS2_PLACEMENT_3D('',#47829,#24020,#24021);
#20785=AXIS2_PLACEMENT_3D('',#47831,#24022,#24023);
#20786=AXIS2_PLACEMENT_3D('',#47832,#24024,#24025);
#20787=AXIS2_PLACEMENT_3D('',#47833,#24026,#24027);
#20788=AXIS2_PLACEMENT_3D('',#47834,#24028,#24029);
#20789=AXIS2_PLACEMENT_3D('',#47835,#24030,#24031);
#20790=AXIS2_PLACEMENT_3D('',#47838,#24032,#24033);
#20791=AXIS2_PLACEMENT_3D('',#47842,#24036,#24037);
#20792=AXIS2_PLACEMENT_3D('',#47843,#24038,#24039);
#20793=AXIS2_PLACEMENT_3D('',#47846,#24041,#24042);
#20794=AXIS2_PLACEMENT_3D('',#47847,#24043,#24044);
#20795=AXIS2_PLACEMENT_3D('',#47851,#24047,#24048);
#20796=AXIS2_PLACEMENT_3D('',#47854,#24050,#24051);
#20797=AXIS2_PLACEMENT_3D('',#47855,#24052,#24053);
#20798=AXIS2_PLACEMENT_3D('',#47859,#24056,#24057);
#20799=AXIS2_PLACEMENT_3D('',#47861,#24058,#24059);
#20800=AXIS2_PLACEMENT_3D('',#47862,#24060,#24061);
#20801=AXIS2_PLACEMENT_3D('',#47863,#24062,#24063);
#20802=AXIS2_PLACEMENT_3D('',#47866,#24066,#24067);
#20803=AXIS2_PLACEMENT_3D('',#47867,#24068,#24069);
#20804=AXIS2_PLACEMENT_3D('',#47871,#24071,#24072);
#20805=AXIS2_PLACEMENT_3D('',#47873,#24074,#24075);
#20806=AXIS2_PLACEMENT_3D('',#47875,#24077,#24078);
#20807=AXIS2_PLACEMENT_3D('',#47877,#24079,#24080);
#20808=AXIS2_PLACEMENT_3D('',#47880,#24082,#24083);
#20809=AXIS2_PLACEMENT_3D('',#47882,#24085,#24086);
#20810=AXIS2_PLACEMENT_3D('',#47883,#24087,#24088);
#20811=AXIS2_PLACEMENT_3D('',#47884,#24089,#24090);
#20812=AXIS2_PLACEMENT_3D('',#47887,#24092,#24093);
#20813=AXIS2_PLACEMENT_3D('',#47888,#24094,#24095);
#20814=AXIS2_PLACEMENT_3D('',#47890,#24096,#24097);
#20815=AXIS2_PLACEMENT_3D('',#47892,#24099,#24100);
#20816=AXIS2_PLACEMENT_3D('',#47895,#24103,#24104);
#20817=AXIS2_PLACEMENT_3D('',#47896,#24105,#24106);
#20818=AXIS2_PLACEMENT_3D('',#47899,#24107,#24108);
#20819=AXIS2_PLACEMENT_3D('',#47903,#24110,#24111);
#20820=AXIS2_PLACEMENT_3D('',#47905,#24113,#24114);
#20821=AXIS2_PLACEMENT_3D('',#47910,#24118,#24119);
#20822=AXIS2_PLACEMENT_3D('',#47912,#24120,#24121);
#20823=AXIS2_PLACEMENT_3D('',#47917,#24122,#24123);
#20824=AXIS2_PLACEMENT_3D('',#47918,#24124,#24125);
#20825=AXIS2_PLACEMENT_3D('',#47919,#24126,#24127);
#20826=AXIS2_PLACEMENT_3D('',#47920,#24128,#24129);
#20827=AXIS2_PLACEMENT_3D('',#47931,#24131,#24132);
#20828=AXIS2_PLACEMENT_3D('',#47932,#24133,#24134);
#20829=AXIS2_PLACEMENT_3D('',#47933,#24135,#24136);
#20830=AXIS2_PLACEMENT_3D('',#47948,#24138,#24139);
#20831=AXIS2_PLACEMENT_3D('',#47949,#24140,#24141);
#20832=AXIS2_PLACEMENT_3D('',#47950,#24142,#24143);
#20833=AXIS2_PLACEMENT_3D('',#47951,#24144,#24145);
#20834=AXIS2_PLACEMENT_3D('',#47953,#24146,#24147);
#20835=AXIS2_PLACEMENT_3D('',#47954,#24148,#24149);
#20836=AXIS2_PLACEMENT_3D('',#47956,#24151,#24152);
#20837=AXIS2_PLACEMENT_3D('',#47957,#24153,#24154);
#20838=AXIS2_PLACEMENT_3D('',#47958,#24155,#24156);
#20839=AXIS2_PLACEMENT_3D('',#47959,#24157,#24158);
#20840=AXIS2_PLACEMENT_3D('',#47960,#24159,#24160);
#20841=AXIS2_PLACEMENT_3D('',#47962,#24162,#24163);
#20842=AXIS2_PLACEMENT_3D('',#47963,#24164,#24165);
#20843=AXIS2_PLACEMENT_3D('',#47964,#24166,#24167);
#20844=AXIS2_PLACEMENT_3D('',#47967,#24168,#24169);
#20845=AXIS2_PLACEMENT_3D('',#47969,#24170,#24171);
#20846=AXIS2_PLACEMENT_3D('',#47970,#24172,#24173);
#20847=AXIS2_PLACEMENT_3D('',#47971,#24174,#24175);
#20848=AXIS2_PLACEMENT_3D('',#47972,#24176,#24177);
#20849=AXIS2_PLACEMENT_3D('',#47976,#24179,#24180);
#20850=AXIS2_PLACEMENT_3D('',#47980,#24182,#24183);
#20851=AXIS2_PLACEMENT_3D('',#47984,#24185,#24186);
#20852=AXIS2_PLACEMENT_3D('',#47988,#24188,#24189);
#20853=AXIS2_PLACEMENT_3D('',#47992,#24191,#24192);
#20854=AXIS2_PLACEMENT_3D('',#47996,#24194,#24195);
#20855=AXIS2_PLACEMENT_3D('',#48000,#24197,#24198);
#20856=AXIS2_PLACEMENT_3D('',#48004,#24200,#24201);
#20857=AXIS2_PLACEMENT_3D('',#48007,#24203,#24204);
#20858=AXIS2_PLACEMENT_3D('',#48008,#24205,#24206);
#20859=AXIS2_PLACEMENT_3D('',#48010,#24207,#24208);
#20860=AXIS2_PLACEMENT_3D('',#48011,#24209,#24210);
#20861=AXIS2_PLACEMENT_3D('',#48027,#24212,#24213);
#20862=AXIS2_PLACEMENT_3D('',#48040,#24215,#24216);
#20863=AXIS2_PLACEMENT_3D('',#48043,#24217,#24218);
#20864=AXIS2_PLACEMENT_3D('',#48044,#24219,#24220);
#20865=AXIS2_PLACEMENT_3D('',#48045,#24221,#24222);
#20866=AXIS2_PLACEMENT_3D('',#48046,#24223,#24224);
#20867=AXIS2_PLACEMENT_3D('',#48049,#24225,#24226);
#20868=AXIS2_PLACEMENT_3D('',#48052,#24229,#24230);
#20869=AXIS2_PLACEMENT_3D('',#48054,#24231,#24232);
#20870=AXIS2_PLACEMENT_3D('',#48055,#24233,#24234);
#20871=AXIS2_PLACEMENT_3D('',#48056,#24235,#24236);
#20872=AXIS2_PLACEMENT_3D('',#48059,#24237,#24238);
#20873=AXIS2_PLACEMENT_3D('',#48061,#24239,#24240);
#20874=AXIS2_PLACEMENT_3D('',#48063,#24241,#24242);
#20875=AXIS2_PLACEMENT_3D('',#48064,#24243,#24244);
#20876=AXIS2_PLACEMENT_3D('',#48065,#24245,#24246);
#20877=AXIS2_PLACEMENT_3D('',#48102,#24247,#24248);
#20878=AXIS2_PLACEMENT_3D('',#48104,#24249,#24250);
#20879=AXIS2_PLACEMENT_3D('',#48108,#24252,#24253);
#20880=AXIS2_PLACEMENT_3D('',#48112,#24255,#24256);
#20881=AXIS2_PLACEMENT_3D('',#48116,#24258,#24259);
#20882=AXIS2_PLACEMENT_3D('',#48120,#24261,#24262);
#20883=AXIS2_PLACEMENT_3D('',#48124,#24264,#24265);
#20884=AXIS2_PLACEMENT_3D('',#48127,#24267,#24268);
#20885=AXIS2_PLACEMENT_3D('',#48129,#24269,#24270);
#20886=AXIS2_PLACEMENT_3D('',#48130,#24271,#24272);
#20887=AXIS2_PLACEMENT_3D('',#48132,#24273,#24274);
#20888=AXIS2_PLACEMENT_3D('',#48133,#24275,#24276);
#20889=AXIS2_PLACEMENT_3D('',#48134,#24277,#24278);
#20890=AXIS2_PLACEMENT_3D('',#48136,#24279,#24280);
#20891=AXIS2_PLACEMENT_3D('',#48141,#24281,#24282);
#20892=AXIS2_PLACEMENT_3D('',#48142,#24283,#24284);
#20893=AXIS2_PLACEMENT_3D('',#48143,#24285,#24286);
#20894=AXIS2_PLACEMENT_3D('',#48147,#24288,#24289);
#20895=AXIS2_PLACEMENT_3D('',#48162,#24290,#24291);
#20896=AXIS2_PLACEMENT_3D('',#48177,#24293,#24294);
#20897=AXIS2_PLACEMENT_3D('',#48188,#24295,#24296);
#20898=AXIS2_PLACEMENT_3D('',#48190,#24297,#24298);
#20899=AXIS2_PLACEMENT_3D('',#48191,#24299,#24300);
#20900=AXIS2_PLACEMENT_3D('',#48192,#24301,#24302);
#20901=AXIS2_PLACEMENT_3D('',#48202,#24304,#24305);
#20902=AXIS2_PLACEMENT_3D('',#48203,#24306,#24307);
#20903=AXIS2_PLACEMENT_3D('',#48205,#24308,#24309);
#20904=AXIS2_PLACEMENT_3D('',#48206,#24310,#24311);
#20905=AXIS2_PLACEMENT_3D('',#48207,#24312,#24313);
#20906=AXIS2_PLACEMENT_3D('',#48213,#24314,#24315);
#20907=AXIS2_PLACEMENT_3D('',#48214,#24316,#24317);
#20908=AXIS2_PLACEMENT_3D('',#48236,#24321,#24322);
#20909=AXIS2_PLACEMENT_3D('',#48248,#24323,#24324);
#20910=AXIS2_PLACEMENT_3D('',#48249,#24325,#24326);
#20911=AXIS2_PLACEMENT_3D('',#48253,#24328,#24329);
#20912=AXIS2_PLACEMENT_3D('',#48308,#24330,#24331);
#20913=AXIS2_PLACEMENT_3D('',#48314,#24332,#24333);
#20914=AXIS2_PLACEMENT_3D('',#48319,#24334,#24335);
#20915=AXIS2_PLACEMENT_3D('',#48320,#24336,#24337);
#20916=AXIS2_PLACEMENT_3D('',#48321,#24338,#24339);
#20917=AXIS2_PLACEMENT_3D('',#48338,#24340,#24341);
#20918=AXIS2_PLACEMENT_3D('',#48339,#24342,#24343);
#20919=AXIS2_PLACEMENT_3D('',#48342,#24345,#24346);
#20920=AXIS2_PLACEMENT_3D('',#48343,#24347,#24348);
#20921=AXIS2_PLACEMENT_3D('',#48344,#24349,#24350);
#20922=AXIS2_PLACEMENT_3D('',#48346,#24351,#24352);
#20923=AXIS2_PLACEMENT_3D('',#48347,#24353,#24354);
#20924=AXIS2_PLACEMENT_3D('',#48369,#24358,#24359);
#20925=AXIS2_PLACEMENT_3D('',#48370,#24360,#24361);
#20926=AXIS2_PLACEMENT_3D('',#48371,#24362,#24363);
#20927=AXIS2_PLACEMENT_3D('',#48380,#24364,#24365);
#20928=AXIS2_PLACEMENT_3D('',#48389,#24366,#24367);
#20929=AXIS2_PLACEMENT_3D('',#48393,#24370,#24371);
#20930=AXIS2_PLACEMENT_3D('',#48402,#24372,#24373);
#20931=AXIS2_PLACEMENT_3D('',#48411,#24374,#24375);
#20932=AXIS2_PLACEMENT_3D('',#48432,#24378,#24379);
#20933=AXIS2_PLACEMENT_3D('',#48434,#24380,#24381);
#20934=AXIS2_PLACEMENT_3D('',#48439,#24382,#24383);
#20935=AXIS2_PLACEMENT_3D('',#48440,#24384,#24385);
#20936=AXIS2_PLACEMENT_3D('',#48441,#24386,#24387);
#20937=AXIS2_PLACEMENT_3D('',#48442,#24388,#24389);
#20938=AXIS2_PLACEMENT_3D('',#48443,#24390,#24391);
#20939=AXIS2_PLACEMENT_3D('',#48446,#24393,#24394);
#20940=AXIS2_PLACEMENT_3D('',#48447,#24395,#24396);
#20941=AXIS2_PLACEMENT_3D('',#48460,#24400,#24401);
#20942=AXIS2_PLACEMENT_3D('',#48469,#24402,#24403);
#20943=AXIS2_PLACEMENT_3D('',#48471,#24404,#24405);
#20944=AXIS2_PLACEMENT_3D('',#48500,#24407,#24408);
#20945=AXIS2_PLACEMENT_3D('',#48506,#24409,#24410);
#20946=AXIS2_PLACEMENT_3D('',#48511,#24411,#24412);
#20947=AXIS2_PLACEMENT_3D('',#48512,#24413,#24414);
#20948=AXIS2_PLACEMENT_3D('',#48513,#24415,#24416);
#20949=AXIS2_PLACEMENT_3D('',#48514,#24417,#24418);
#20950=AXIS2_PLACEMENT_3D('',#48515,#24419,#24420);
#20951=AXIS2_PLACEMENT_3D('',#48516,#24421,#24422);
#20952=AXIS2_PLACEMENT_3D('',#48518,#24423,#24424);
#20953=AXIS2_PLACEMENT_3D('',#48519,#24425,#24426);
#20954=AXIS2_PLACEMENT_3D('',#48520,#24427,#24428);
#20955=AXIS2_PLACEMENT_3D('',#48522,#24429,#24430);
#20956=AXIS2_PLACEMENT_3D('',#48527,#24431,#24432);
#20957=AXIS2_PLACEMENT_3D('',#48529,#24433,#24434);
#20958=AXIS2_PLACEMENT_3D('',#48536,#24435,#24436);
#20959=AXIS2_PLACEMENT_3D('',#48540,#24438,#24439);
#20960=AXIS2_PLACEMENT_3D('',#48543,#24441,#24442);
#20961=AXIS2_PLACEMENT_3D('',#48544,#24443,#24444);
#20962=AXIS2_PLACEMENT_3D('',#48546,#24445,#24446);
#20963=AXIS2_PLACEMENT_3D('',#48547,#24447,#24448);
#20964=AXIS2_PLACEMENT_3D('',#48577,#24449,#24450);
#20965=AXIS2_PLACEMENT_3D('',#48582,#24451,#24452);
#20966=AXIS2_PLACEMENT_3D('',#48600,#24454,#24455);
#20967=AXIS2_PLACEMENT_3D('',#48601,#24456,#24457);
#20968=AXIS2_PLACEMENT_3D('',#48602,#24458,#24459);
#20969=AXIS2_PLACEMENT_3D('',#48603,#24460,#24461);
#20970=AXIS2_PLACEMENT_3D('',#48606,#24463,#24464);
#20971=AXIS2_PLACEMENT_3D('',#48607,#24465,#24466);
#20972=AXIS2_PLACEMENT_3D('',#48609,#24467,#24468);
#20973=AXIS2_PLACEMENT_3D('',#48610,#24469,#24470);
#20974=AXIS2_PLACEMENT_3D('',#48611,#24471,#24472);
#20975=AXIS2_PLACEMENT_3D('',#48613,#24474,#24475);
#20976=AXIS2_PLACEMENT_3D('',#48614,#24476,#24477);
#20977=AXIS2_PLACEMENT_3D('',#48615,#24478,#24479);
#20978=AXIS2_PLACEMENT_3D('',#48617,#24481,#24482);
#20979=AXIS2_PLACEMENT_3D('',#48623,#24486,#24487);
#20980=AXIS2_PLACEMENT_3D('',#48624,#24488,#24489);
#20981=AXIS2_PLACEMENT_3D('',#48625,#24490,#24491);
#20982=AXIS2_PLACEMENT_3D('',#48626,#24492,#24493);
#20983=AXIS2_PLACEMENT_3D('',#48627,#24494,#24495);
#20984=AXIS2_PLACEMENT_3D('',#48628,#24496,#24497);
#20985=AXIS2_PLACEMENT_3D('',#48629,#24498,#24499);
#20986=AXIS2_PLACEMENT_3D('',#48631,#24500,#24501);
#20987=AXIS2_PLACEMENT_3D('',#48632,#24502,#24503);
#20988=AXIS2_PLACEMENT_3D('',#48633,#24504,#24505);
#20989=AXIS2_PLACEMENT_3D('',#48637,#24507,#24508);
#20990=AXIS2_PLACEMENT_3D('',#48638,#24509,#24510);
#20991=AXIS2_PLACEMENT_3D('',#48639,#24511,#24512);
#20992=AXIS2_PLACEMENT_3D('',#48642,#24513,#24514);
#20993=AXIS2_PLACEMENT_3D('',#48644,#24515,#24516);
#20994=AXIS2_PLACEMENT_3D('',#48645,#24517,#24518);
#20995=AXIS2_PLACEMENT_3D('',#48646,#24519,#24520);
#20996=AXIS2_PLACEMENT_3D('',#48649,#24521,#24522);
#20997=AXIS2_PLACEMENT_3D('',#48652,#24525,#24526);
#20998=AXIS2_PLACEMENT_3D('',#48662,#24532,#24533);
#20999=AXIS2_PLACEMENT_3D('',#48665,#24535,#24536);
#21000=AXIS2_PLACEMENT_3D('',#48666,#24537,#24538);
#21001=AXIS2_PLACEMENT_3D('',#48669,#24539,#24540);
#21002=AXIS2_PLACEMENT_3D('',#48673,#24542,#24543);
#21003=AXIS2_PLACEMENT_3D('',#48675,#24544,#24545);
#21004=AXIS2_PLACEMENT_3D('',#48678,#24547,#24548);
#21005=AXIS2_PLACEMENT_3D('',#48679,#24549,#24550);
#21006=AXIS2_PLACEMENT_3D('',#48683,#24552,#24553);
#21007=AXIS2_PLACEMENT_3D('',#48686,#24555,#24556);
#21008=AXIS2_PLACEMENT_3D('',#48687,#24557,#24558);
#21009=AXIS2_PLACEMENT_3D('',#48691,#24561,#24562);
#21010=AXIS2_PLACEMENT_3D('',#48693,#24563,#24564);
#21011=AXIS2_PLACEMENT_3D('',#48696,#24566,#24567);
#21012=AXIS2_PLACEMENT_3D('',#48697,#24568,#24569);
#21013=AXIS2_PLACEMENT_3D('',#48698,#24570,#24571);
#21014=AXIS2_PLACEMENT_3D('',#48699,#24572,#24573);
#21015=AXIS2_PLACEMENT_3D('',#48700,#24574,#24575);
#21016=AXIS2_PLACEMENT_3D('',#48706,#24579,#24580);
#21017=AXIS2_PLACEMENT_3D('',#48710,#24582,#24583);
#21018=AXIS2_PLACEMENT_3D('',#48712,#24585,#24586);
#21019=AXIS2_PLACEMENT_3D('',#48716,#24588,#24589);
#21020=AXIS2_PLACEMENT_3D('',#48723,#24590,#24591);
#21021=AXIS2_PLACEMENT_3D('',#48724,#24592,#24593);
#21022=AXIS2_PLACEMENT_3D('',#48725,#24594,#24595);
#21023=AXIS2_PLACEMENT_3D('',#48726,#24596,#24597);
#21024=AXIS2_PLACEMENT_3D('',#48728,#24598,#24599);
#21025=AXIS2_PLACEMENT_3D('',#48729,#24600,#24601);
#21026=AXIS2_PLACEMENT_3D('',#48731,#24602,#24603);
#21027=AXIS2_PLACEMENT_3D('',#48732,#24604,#24605);
#21028=AXIS2_PLACEMENT_3D('',#48733,#24606,#24607);
#21029=AXIS2_PLACEMENT_3D('',#48737,#24609,#24610);
#21030=AXIS2_PLACEMENT_3D('',#48738,#24611,#24612);
#21031=AXIS2_PLACEMENT_3D('',#48739,#24613,#24614);
#21032=AXIS2_PLACEMENT_3D('',#48741,#24615,#24616);
#21033=AXIS2_PLACEMENT_3D('',#48743,#24617,#24618);
#21034=AXIS2_PLACEMENT_3D('',#48745,#24620,#24621);
#21035=AXIS2_PLACEMENT_3D('',#48746,#24622,#24623);
#21036=AXIS2_PLACEMENT_3D('',#48747,#24624,#24625);
#21037=AXIS2_PLACEMENT_3D('',#48749,#24626,#24627);
#21038=AXIS2_PLACEMENT_3D('',#48751,#24629,#24630);
#21039=AXIS2_PLACEMENT_3D('',#48752,#24631,#24632);
#21040=AXIS2_PLACEMENT_3D('',#48753,#24633,#24634);
#21041=AXIS2_PLACEMENT_3D('',#48756,#24636,#24637);
#21042=AXIS2_PLACEMENT_3D('',#48757,#24638,#24639);
#21043=AXIS2_PLACEMENT_3D('',#48760,#24640,#24641);
#21044=AXIS2_PLACEMENT_3D('',#48761,#24642,#24643);
#21045=AXIS2_PLACEMENT_3D('',#48762,#24644,#24645);
#21046=AXIS2_PLACEMENT_3D('',#48763,#24646,#24647);
#21047=AXIS2_PLACEMENT_3D('',#48767,#24649,#24650);
#21048=AXIS2_PLACEMENT_3D('',#48769,#24652,#24653);
#21049=AXIS2_PLACEMENT_3D('',#48771,#24655,#24656);
#21050=AXIS2_PLACEMENT_3D('',#48773,#24657,#24658);
#21051=AXIS2_PLACEMENT_3D('',#48775,#24660,#24661);
#21052=AXIS2_PLACEMENT_3D('',#48778,#24663,#24664);
#21053=AXIS2_PLACEMENT_3D('',#48779,#24665,#24666);
#21054=AXIS2_PLACEMENT_3D('',#48780,#24667,#24668);
#21055=AXIS2_PLACEMENT_3D('',#48781,#24669,#24670);
#21056=AXIS2_PLACEMENT_3D('',#48783,#24672,#24673);
#21057=AXIS2_PLACEMENT_3D('',#48786,#24675,#24676);
#21058=AXIS2_PLACEMENT_3D('',#48787,#24677,#24678);
#21059=AXIS2_PLACEMENT_3D('',#48791,#24681,#24682);
#21060=AXIS2_PLACEMENT_3D('',#48794,#24683,#24684);
#21061=AXIS2_PLACEMENT_3D('',#48796,#24685,#24686);
#21062=AXIS2_PLACEMENT_3D('',#48797,#24687,#24688);
#21063=AXIS2_PLACEMENT_3D('',#48798,#24689,#24690);
#21064=AXIS2_PLACEMENT_3D('',#48799,#24691,#24692);
#21065=AXIS2_PLACEMENT_3D('',#48802,#24693,#24694);
#21066=AXIS2_PLACEMENT_3D('',#48804,#24696,#24697);
#21067=AXIS2_PLACEMENT_3D('',#48805,#24698,#24699);
#21068=AXIS2_PLACEMENT_3D('',#48807,#24700,#24701);
#21069=AXIS2_PLACEMENT_3D('',#48808,#24702,#24703);
#21070=AXIS2_PLACEMENT_3D('',#48811,#24704,#24705);
#21071=AXIS2_PLACEMENT_3D('',#48812,#24706,#24707);
#21072=AXIS2_PLACEMENT_3D('',#48813,#24708,#24709);
#21073=AXIS2_PLACEMENT_3D('',#48814,#24710,#24711);
#21074=AXIS2_PLACEMENT_3D('',#48817,#24712,#24713);
#21075=AXIS2_PLACEMENT_3D('',#48819,#24715,#24716);
#21076=AXIS2_PLACEMENT_3D('',#48820,#24717,#24718);
#21077=AXIS2_PLACEMENT_3D('',#48821,#24719,#24720);
#21078=AXIS2_PLACEMENT_3D('',#48822,#24721,#24722);
#21079=AXIS2_PLACEMENT_3D('',#48823,#24723,#24724);
#21080=AXIS2_PLACEMENT_3D('',#48825,#24725,#24726);
#21081=AXIS2_PLACEMENT_3D('',#48826,#24727,#24728);
#21082=AXIS2_PLACEMENT_3D('',#48827,#24729,#24730);
#21083=AXIS2_PLACEMENT_3D('',#48828,#24731,#24732);
#21084=AXIS2_PLACEMENT_3D('',#48830,#24733,#24734);
#21085=AXIS2_PLACEMENT_3D('',#48831,#24735,#24736);
#21086=AXIS2_PLACEMENT_3D('',#48833,#24737,#24738);
#21087=AXIS2_PLACEMENT_3D('',#48834,#24739,#24740);
#21088=AXIS2_PLACEMENT_3D('',#48835,#24741,#24742);
#21089=AXIS2_PLACEMENT_3D('',#48837,#24744,#24745);
#21090=AXIS2_PLACEMENT_3D('',#48841,#24748,#24749);
#21091=AXIS2_PLACEMENT_3D('',#48844,#24751,#24752);
#21092=AXIS2_PLACEMENT_3D('',#48845,#24753,#24754);
#21093=AXIS2_PLACEMENT_3D('',#48846,#24755,#24756);
#21094=AXIS2_PLACEMENT_3D('',#48847,#24757,#24758);
#21095=AXIS2_PLACEMENT_3D('',#48855,#24763,#24764);
#21096=AXIS2_PLACEMENT_3D('',#48856,#24765,#24766);
#21097=AXIS2_PLACEMENT_3D('',#48857,#24767,#24768);
#21098=AXIS2_PLACEMENT_3D('',#48859,#24769,#24770);
#21099=AXIS2_PLACEMENT_3D('',#48860,#24771,#24772);
#21100=AXIS2_PLACEMENT_3D('',#48861,#24773,#24774);
#21101=AXIS2_PLACEMENT_3D('',#48865,#24776,#24777);
#21102=AXIS2_PLACEMENT_3D('',#48866,#24778,#24779);
#21103=AXIS2_PLACEMENT_3D('',#48867,#24780,#24781);
#21104=AXIS2_PLACEMENT_3D('',#48869,#24782,#24783);
#21105=AXIS2_PLACEMENT_3D('',#48870,#24784,#24785);
#21106=AXIS2_PLACEMENT_3D('',#48871,#24786,#24787);
#21107=AXIS2_PLACEMENT_3D('',#48875,#24789,#24790);
#21108=AXIS2_PLACEMENT_3D('',#48876,#24791,#24792);
#21109=AXIS2_PLACEMENT_3D('',#48877,#24793,#24794);
#21110=AXIS2_PLACEMENT_3D('',#48879,#24795,#24796);
#21111=AXIS2_PLACEMENT_3D('',#48881,#24797,#24798);
#21112=AXIS2_PLACEMENT_3D('',#48883,#24799,#24800);
#21113=AXIS2_PLACEMENT_3D('',#48884,#24801,#24802);
#21114=AXIS2_PLACEMENT_3D('',#48885,#24803,#24804);
#21115=AXIS2_PLACEMENT_3D('',#48887,#24805,#24806);
#21116=AXIS2_PLACEMENT_3D('',#48889,#24807,#24808);
#21117=AXIS2_PLACEMENT_3D('',#48891,#24809,#24810);
#21118=AXIS2_PLACEMENT_3D('',#48893,#24811,#24812);
#21119=AXIS2_PLACEMENT_3D('',#48895,#24813,#24814);
#21120=AXIS2_PLACEMENT_3D('',#48897,#24815,#24816);
#21121=AXIS2_PLACEMENT_3D('',#48899,#24817,#24818);
#21122=AXIS2_PLACEMENT_3D('',#48901,#24819,#24820);
#21123=AXIS2_PLACEMENT_3D('',#48903,#24821,#24822);
#21124=AXIS2_PLACEMENT_3D('',#48905,#24823,#24824);
#21125=AXIS2_PLACEMENT_3D('',#48907,#24825,#24826);
#21126=AXIS2_PLACEMENT_3D('',#48908,#24827,#24828);
#21127=AXIS2_PLACEMENT_3D('',#48910,#24829,#24830);
#21128=AXIS2_PLACEMENT_3D('',#48912,#24832,#24833);
#21129=AXIS2_PLACEMENT_3D('',#48914,#24834,#24835);
#21130=AXIS2_PLACEMENT_3D('',#48916,#24836,#24837);
#21131=AXIS2_PLACEMENT_3D('',#48917,#24838,#24839);
#21132=AXIS2_PLACEMENT_3D('',#48918,#24840,#24841);
#21133=AXIS2_PLACEMENT_3D('',#48920,#24842,#24843);
#21134=AXIS2_PLACEMENT_3D('',#48922,#24845,#24846);
#21135=AXIS2_PLACEMENT_3D('',#48923,#24847,#24848);
#21136=AXIS2_PLACEMENT_3D('',#48924,#24849,#24850);
#21137=AXIS2_PLACEMENT_3D('',#48925,#24851,#24852);
#21138=AXIS2_PLACEMENT_3D('',#48926,#24853,#24854);
#21139=AXIS2_PLACEMENT_3D('',#48927,#24855,#24856);
#21140=AXIS2_PLACEMENT_3D('',#48928,#24857,#24858);
#21141=AXIS2_PLACEMENT_3D('',#48930,#24859,#24860);
#21142=AXIS2_PLACEMENT_3D('',#48932,#24861,#24862);
#21143=AXIS2_PLACEMENT_3D('',#48933,#24863,#24864);
#21144=AXIS2_PLACEMENT_3D('',#48934,#24865,#24866);
#21145=AXIS2_PLACEMENT_3D('',#48936,#24867,#24868);
#21146=AXIS2_PLACEMENT_3D('',#48938,#24870,#24871);
#21147=AXIS2_PLACEMENT_3D('',#48939,#24872,#24873);
#21148=AXIS2_PLACEMENT_3D('',#48940,#24874,#24875);
#21149=AXIS2_PLACEMENT_3D('',#48941,#24876,#24877);
#21150=AXIS2_PLACEMENT_3D('',#48942,#24878,#24879);
#21151=AXIS2_PLACEMENT_3D('',#48944,#24880,#24881);
#21152=AXIS2_PLACEMENT_3D('',#48946,#24882,#24883);
#21153=AXIS2_PLACEMENT_3D('',#48947,#24884,#24885);
#21154=AXIS2_PLACEMENT_3D('',#48948,#24886,#24887);
#21155=AXIS2_PLACEMENT_3D('',#48950,#24888,#24889);
#21156=AXIS2_PLACEMENT_3D('',#48952,#24891,#24892);
#21157=AXIS2_PLACEMENT_3D('',#48954,#24893,#24894);
#21158=AXIS2_PLACEMENT_3D('',#48955,#24895,#24896);
#21159=AXIS2_PLACEMENT_3D('',#48957,#24897,#24898);
#21160=AXIS2_PLACEMENT_3D('',#48959,#24899,#24900);
#21161=AXIS2_PLACEMENT_3D('',#48960,#24901,#24902);
#21162=AXIS2_PLACEMENT_3D('',#48961,#24903,#24904);
#21163=AXIS2_PLACEMENT_3D('',#48963,#24905,#24906);
#21164=AXIS2_PLACEMENT_3D('',#48965,#24908,#24909);
#21165=AXIS2_PLACEMENT_3D('',#48967,#24910,#24911);
#21166=AXIS2_PLACEMENT_3D('',#48968,#24912,#24913);
#21167=AXIS2_PLACEMENT_3D('',#48970,#24914,#24915);
#21168=AXIS2_PLACEMENT_3D('',#48972,#24916,#24917);
#21169=AXIS2_PLACEMENT_3D('',#48973,#24918,#24919);
#21170=AXIS2_PLACEMENT_3D('',#48974,#24920,#24921);
#21171=AXIS2_PLACEMENT_3D('',#48976,#24922,#24923);
#21172=AXIS2_PLACEMENT_3D('',#48978,#24925,#24926);
#21173=AXIS2_PLACEMENT_3D('',#48980,#24927,#24928);
#21174=AXIS2_PLACEMENT_3D('',#48981,#24929,#24930);
#21175=AXIS2_PLACEMENT_3D('',#48985,#24932,#24933);
#21176=AXIS2_PLACEMENT_3D('',#48987,#24935,#24936);
#21177=AXIS2_PLACEMENT_3D('',#48988,#24937,#24938);
#21178=AXIS2_PLACEMENT_3D('',#48990,#24940,#24941);
#21179=AXIS2_PLACEMENT_3D('',#48991,#24942,#24943);
#21180=AXIS2_PLACEMENT_3D('',#48992,#24944,#24945);
#21181=AXIS2_PLACEMENT_3D('',#49016,#24949,#24950);
#21182=AXIS2_PLACEMENT_3D('',#49018,#24951,#24952);
#21183=AXIS2_PLACEMENT_3D('',#49030,#24953,#24954);
#21184=AXIS2_PLACEMENT_3D('',#49033,#24955,#24956);
#21185=AXIS2_PLACEMENT_3D('',#49034,#24957,#24958);
#21186=AXIS2_PLACEMENT_3D('',#49036,#24959,#24960);
#21187=AXIS2_PLACEMENT_3D('',#49038,#24961,#24962);
#21188=AXIS2_PLACEMENT_3D('',#49039,#24963,#24964);
#21189=AXIS2_PLACEMENT_3D('',#49040,#24965,#24966);
#21190=AXIS2_PLACEMENT_3D('',#49044,#24968,#24969);
#21191=AXIS2_PLACEMENT_3D('',#49045,#24970,#24971);
#21192=AXIS2_PLACEMENT_3D('',#49046,#24972,#24973);
#21193=AXIS2_PLACEMENT_3D('',#49049,#24974,#24975);
#21194=AXIS2_PLACEMENT_3D('',#49051,#24977,#24978);
#21195=AXIS2_PLACEMENT_3D('',#49052,#24979,#24980);
#21196=AXIS2_PLACEMENT_3D('',#49054,#24981,#24982);
#21197=AXIS2_PLACEMENT_3D('',#49055,#24983,#24984);
#21198=AXIS2_PLACEMENT_3D('',#49056,#24985,#24986);
#21199=AXIS2_PLACEMENT_3D('',#49058,#24987,#24988);
#21200=AXIS2_PLACEMENT_3D('',#49060,#24989,#24990);
#21201=AXIS2_PLACEMENT_3D('',#49062,#24991,#24992);
#21202=AXIS2_PLACEMENT_3D('',#49064,#24993,#24994);
#21203=AXIS2_PLACEMENT_3D('',#49066,#24995,#24996);
#21204=AXIS2_PLACEMENT_3D('',#49068,#24997,#24998);
#21205=AXIS2_PLACEMENT_3D('',#49070,#24999,#25000);
#21206=AXIS2_PLACEMENT_3D('',#49071,#25001,#25002);
#21207=AXIS2_PLACEMENT_3D('',#49072,#25003,#25004);
#21208=AXIS2_PLACEMENT_3D('',#49073,#25005,#25006);
#21209=AXIS2_PLACEMENT_3D('',#49074,#25007,#25008);
#21210=AXIS2_PLACEMENT_3D('',#49075,#25009,#25010);
#21211=AXIS2_PLACEMENT_3D('',#49076,#25011,#25012);
#21212=AXIS2_PLACEMENT_3D('',#49077,#25013,#25014);
#21213=AXIS2_PLACEMENT_3D('',#49080,#25015,#25016);
#21214=AXIS2_PLACEMENT_3D('',#49081,#25017,#25018);
#21215=AXIS2_PLACEMENT_3D('',#49082,#25019,#25020);
#21216=AXIS2_PLACEMENT_3D('',#49083,#25021,#25022);
#21217=AXIS2_PLACEMENT_3D('',#49087,#25024,#25025);
#21218=AXIS2_PLACEMENT_3D('',#49088,#25026,#25027);
#21219=AXIS2_PLACEMENT_3D('',#49089,#25028,#25029);
#21220=AXIS2_PLACEMENT_3D('',#49092,#25030,#25031);
#21221=AXIS2_PLACEMENT_3D('',#49093,#25032,#25033);
#21222=AXIS2_PLACEMENT_3D('',#49094,#25034,#25035);
#21223=AXIS2_PLACEMENT_3D('',#49095,#25036,#25037);
#21224=AXIS2_PLACEMENT_3D('',#49099,#25039,#25040);
#21225=AXIS2_PLACEMENT_3D('',#49100,#25041,#25042);
#21226=AXIS2_PLACEMENT_3D('',#49101,#25043,#25044);
#21227=AXIS2_PLACEMENT_3D('',#49102,#25045,#25046);
#21228=AXIS2_PLACEMENT_3D('',#49103,#25047,#25048);
#21229=AXIS2_PLACEMENT_3D('',#49105,#25049,#25050);
#21230=AXIS2_PLACEMENT_3D('',#49107,#25051,#25052);
#21231=AXIS2_PLACEMENT_3D('',#49108,#25053,#25054);
#21232=AXIS2_PLACEMENT_3D('',#49109,#25055,#25056);
#21233=AXIS2_PLACEMENT_3D('',#49112,#25057,#25058);
#21234=AXIS2_PLACEMENT_3D('',#49114,#25060,#25061);
#21235=AXIS2_PLACEMENT_3D('',#49115,#25062,#25063);
#21236=AXIS2_PLACEMENT_3D('',#49118,#25064,#25065);
#21237=AXIS2_PLACEMENT_3D('',#49119,#25066,#25067);
#21238=AXIS2_PLACEMENT_3D('',#49120,#25068,#25069);
#21239=AXIS2_PLACEMENT_3D('',#49121,#25070,#25071);
#21240=AXIS2_PLACEMENT_3D('',#49123,#25072,#25073);
#21241=AXIS2_PLACEMENT_3D('',#49126,#25075,#25076);
#21242=AXIS2_PLACEMENT_3D('',#49131,#25077,#25078);
#21243=AXIS2_PLACEMENT_3D('',#49132,#25079,#25080);
#21244=AXIS2_PLACEMENT_3D('',#49133,#25081,#25082);
#21245=AXIS2_PLACEMENT_3D('',#49134,#25083,#25084);
#21246=AXIS2_PLACEMENT_3D('',#49135,#25085,#25086);
#21247=AXIS2_PLACEMENT_3D('',#49136,#25087,#25088);
#21248=AXIS2_PLACEMENT_3D('',#49137,#25089,#25090);
#21249=AXIS2_PLACEMENT_3D('',#49144,#25091,#25092);
#21250=AXIS2_PLACEMENT_3D('',#49153,#25093,#25094);
#21251=AXIS2_PLACEMENT_3D('',#49154,#25095,#25096);
#21252=AXIS2_PLACEMENT_3D('',#49156,#25097,#25098);
#21253=AXIS2_PLACEMENT_3D('',#49158,#25099,#25100);
#21254=AXIS2_PLACEMENT_3D('',#49160,#25101,#25102);
#21255=AXIS2_PLACEMENT_3D('',#49161,#25103,#25104);
#21256=AXIS2_PLACEMENT_3D('',#49162,#25105,#25106);
#21257=AXIS2_PLACEMENT_3D('',#49166,#25109,#25110);
#21258=AXIS2_PLACEMENT_3D('',#49168,#25111,#25112);
#21259=AXIS2_PLACEMENT_3D('',#49170,#25113,#25114);
#21260=AXIS2_PLACEMENT_3D('',#49171,#25115,#25116);
#21261=AXIS2_PLACEMENT_3D('',#49173,#25118,#25119);
#21262=AXIS2_PLACEMENT_3D('',#49175,#25120,#25121);
#21263=AXIS2_PLACEMENT_3D('',#49177,#25122,#25123);
#21264=AXIS2_PLACEMENT_3D('',#49178,#25124,#25125);
#21265=AXIS2_PLACEMENT_3D('',#49179,#25126,#25127);
#21266=AXIS2_PLACEMENT_3D('',#49181,#25129,#25130);
#21267=AXIS2_PLACEMENT_3D('',#49183,#25131,#25132);
#21268=AXIS2_PLACEMENT_3D('',#49185,#25133,#25134);
#21269=AXIS2_PLACEMENT_3D('',#49186,#25135,#25136);
#21270=AXIS2_PLACEMENT_3D('',#49187,#25137,#25138);
#21271=AXIS2_PLACEMENT_3D('',#49189,#25140,#25141);
#21272=AXIS2_PLACEMENT_3D('',#49192,#25142,#25143);
#21273=AXIS2_PLACEMENT_3D('',#49193,#25144,#25145);
#21274=AXIS2_PLACEMENT_3D('',#49194,#25146,#25147);
#21275=AXIS2_PLACEMENT_3D('',#49195,#25148,#25149);
#21276=AXIS2_PLACEMENT_3D('',#49199,#25151,#25152);
#21277=AXIS2_PLACEMENT_3D('',#49200,#25153,#25154);
#21278=AXIS2_PLACEMENT_3D('',#49201,#25155,#25156);
#21279=AXIS2_PLACEMENT_3D('',#49202,#25157,#25158);
#21280=AXIS2_PLACEMENT_3D('',#49203,#25159,#25160);
#21281=AXIS2_PLACEMENT_3D('',#49205,#25162,#25163);
#21282=AXIS2_PLACEMENT_3D('',#49206,#25164,#25165);
#21283=AXIS2_PLACEMENT_3D('',#49207,#25166,#25167);
#21284=AXIS2_PLACEMENT_3D('',#49208,#25168,#25169);
#21285=AXIS2_PLACEMENT_3D('',#49209,#25170,#25171);
#21286=AXIS2_PLACEMENT_3D('',#49210,#25172,#25173);
#21287=AXIS2_PLACEMENT_3D('',#49211,#25174,#25175);
#21288=AXIS2_PLACEMENT_3D('',#49213,#25177,#25178);
#21289=AXIS2_PLACEMENT_3D('',#49214,#25179,#25180);
#21290=AXIS2_PLACEMENT_3D('',#49215,#25181,#25182);
#21291=AXIS2_PLACEMENT_3D('',#49216,#25183,#25184);
#21292=AXIS2_PLACEMENT_3D('',#49217,#25185,#25186);
#21293=AXIS2_PLACEMENT_3D('',#49218,#25187,#25188);
#21294=AXIS2_PLACEMENT_3D('',#49219,#25189,#25190);
#21295=AXIS2_PLACEMENT_3D('',#49221,#25192,#25193);
#21296=AXIS2_PLACEMENT_3D('',#49223,#25195,#25196);
#21297=AXIS2_PLACEMENT_3D('',#49225,#25198,#25199);
#23433=DIRECTION('axis',(0.,0.,1.));
#23434=DIRECTION('refdir',(1.,0.,0.));
#23435=DIRECTION('center_axis',(0.,-0.707106781186548,-0.707106781186547));
#23436=DIRECTION('ref_axis',(0.38268343236509,-0.653281482438183,0.653281482438193));
#23437=DIRECTION('center_axis',(-8.8931018167636E-15,0.707106781186548,
0.707106781186548));
#23438=DIRECTION('ref_axis',(2.22044604925032E-15,-0.707106781186548,0.707106781186548));
#23439=DIRECTION('',(0.,0.707106781186548,0.707106781186547));
#23440=DIRECTION('center_axis',(-3.6799042000401E-15,-0.707106781186556,
-0.707106781186539));
#23441=DIRECTION('ref_axis',(0.707106781186546,-0.499999999999997,0.500000000000005));
#23442=DIRECTION('',(0.,-0.707106781186548,-0.707106781186547));
#23443=DIRECTION('center_axis',(-3.5527136788005E-15,-1.,-7.105427357601E-15));
#23444=DIRECTION('ref_axis',(0.505449465124414,-7.10542735760101E-15,0.862856209461022));
#23445=DIRECTION('center_axis',(0.,-0.707106781186547,0.707106781186548));
#23446=DIRECTION('ref_axis',(0.382683432365091,0.653281482438193,0.653281482438184));
#23447=DIRECTION('center_axis',(1.,0.,0.));
#23448=DIRECTION('ref_axis',(0.,0.,1.));
#23449=DIRECTION('center_axis',(-0.577350269189627,4.48691293489498E-16,
0.816496580927725));
#23450=DIRECTION('ref_axis',(0.816496580927726,0.,0.577350269189626));
#23451=DIRECTION('center_axis',(0.577350269189627,0.816496580927725,0.));
#23452=DIRECTION('ref_axis',(0.816496580927726,-0.577350269189625,0.));
#23453=DIRECTION('center_axis',(-0.577350269189625,-0.816496580927727,1.25192883228097E-15));
#23454=DIRECTION('ref_axis',(0.707106781186548,-0.5,-0.5));
#23455=DIRECTION('',(-0.577350269189627,-0.816496580927725,-2.7755575615629E-17));
#23456=DIRECTION('center_axis',(-0.577350269189627,-0.816496580927725,1.25192883228098E-15));
#23457=DIRECTION('ref_axis',(0.707106781186547,-0.5,-0.5));
#23458=DIRECTION('',(0.577350269189627,0.816496580927725,-2.7755575615629E-17));
#23459=DIRECTION('center_axis',(0.,-0.707106781186548,0.707106781186547));
#23460=DIRECTION('ref_axis',(0.923879532511285,-0.270598050073102,-0.270598050073102));
#23461=DIRECTION('center_axis',(0.,-0.707106781186548,0.707106781186548));
#23462=DIRECTION('ref_axis',(0.707106781186546,-0.500000000000001,-0.500000000000001));
#23463=DIRECTION('',(0.,-0.707106781186548,0.707106781186547));
#23464=DIRECTION('center_axis',(0.,0.707106781186548,-0.707106781186548));
#23465=DIRECTION('ref_axis',(1.,0.,0.));
#23466=DIRECTION('',(0.,0.707106781186548,-0.707106781186547));
#23467=DIRECTION('center_axis',(0.,0.,1.));
#23468=DIRECTION('ref_axis',(1.,0.,0.));
#23469=DIRECTION('center_axis',(0.,-0.707106781186548,-0.707106781186547));
#23470=DIRECTION('ref_axis',(0.923879532511286,-0.270598050073101,0.270598050073101));
#23471=DIRECTION('center_axis',(0.,0.,1.));
#23472=DIRECTION('ref_axis',(1.,0.,0.));
#23473=DIRECTION('center_axis',(0.,-0.707106781186547,0.707106781186548));
#23474=DIRECTION('ref_axis',(0.382683432365089,0.653281482438189,0.653281482438189));
#23475=DIRECTION('center_axis',(-0.577350269189627,0.816496580927725,-1.92296268638356E-16));
#23476=DIRECTION('ref_axis',(0.816496580927725,0.577350269189628,0.));
#23477=DIRECTION('center_axis',(0.,0.707106781186548,0.707106781186548));
#23478=DIRECTION('ref_axis',(0.707106781186548,0.5,-0.5));
#23479=DIRECTION('center_axis',(1.,0.,0.));
#23480=DIRECTION('ref_axis',(0.,1.,0.));
#23481=DIRECTION('center_axis',(0.,0.707106781186548,0.707106781186548));
#23482=DIRECTION('ref_axis',(0.382683432365087,0.653281482438192,-0.653281482438187));
#23483=DIRECTION('center_axis',(3.12791857003412E-15,0.707106781186545,
0.70710678118655));
#23484=DIRECTION('ref_axis',(0.707106781186547,0.5,-0.5));
#23485=DIRECTION('',(0.,0.707106781186547,0.707106781186547));
#23486=DIRECTION('',(0.,-0.707106781186547,-0.707106781186547));
#23487=DIRECTION('center_axis',(0.577350269189627,-1.92296268638356E-16,
0.816496580927725));
#23488=DIRECTION('ref_axis',(0.816496580927726,0.,-0.577350269189626));
#23489=DIRECTION('center_axis',(-0.577350269189628,4.90756102254141E-15,
-0.816496580927725));
#23490=DIRECTION('ref_axis',(0.707106781186548,0.5,-0.5));
#23491=DIRECTION('',(-0.577350269189627,1.92296268638356E-16,-0.816496580927725));
#23492=DIRECTION('center_axis',(-0.577350269189625,0.,-0.816496580927726));
#23493=DIRECTION('ref_axis',(0.707106781186548,0.5,-0.5));
#23494=DIRECTION('',(0.577350269189627,-1.92296268638356E-16,0.816496580927725));
#23495=DIRECTION('center_axis',(0.,0.,1.));
#23496=DIRECTION('ref_axis',(1.,0.,0.));
#23497=DIRECTION('center_axis',(0.,-0.707106781186548,-0.707106781186548));
#23498=DIRECTION('ref_axis',(0.92387953251129,0.270598050073092,-0.270598050073092));
#23499=DIRECTION('center_axis',(-0.577350269189627,4.48691293489498E-16,
0.816496580927725));
#23500=DIRECTION('ref_axis',(0.816496580927726,0.,0.577350269189626));
#23501=DIRECTION('',(0.577350269189627,-4.76446869105127E-16,-0.816496580927725));
#23502=DIRECTION('center_axis',(-0.577350269189626,0.,0.816496580927726));
#23503=DIRECTION('ref_axis',(0.707106781186547,-0.5,0.5));
#23504=DIRECTION('',(-0.577350269189627,4.20935717873869E-16,0.816496580927725));
#23505=DIRECTION('center_axis',(0.707106781186546,-0.5,0.500000000000001));
#23506=DIRECTION('ref_axis',(0.577350269189627,0.,-0.816496580927725));
#23507=DIRECTION('',(0.,-0.707106781186548,-0.707106781186547));
#23508=DIRECTION('center_axis',(0.,0.707106781186548,0.707106781186547));
#23509=DIRECTION('ref_axis',(0.923879532511287,-0.270598050073103,0.270598050073094));
#23510=DIRECTION('',(0.,0.707106781186548,0.707106781186547));
#23511=DIRECTION('center_axis',(0.,-0.707106781186548,-0.707106781186548));
#23512=DIRECTION('ref_axis',(1.,0.,0.));
#23513=DIRECTION('center_axis',(1.,0.,0.));
#23514=DIRECTION('ref_axis',(0.,0.,-1.));
#23515=DIRECTION('',(0.,-0.707106781186548,-0.707106781186548));
#23516=DIRECTION('',(0.,0.707106781186547,-0.707106781186548));
#23517=DIRECTION('center_axis',(0.,-0.707106781186548,-0.707106781186548));
#23518=DIRECTION('ref_axis',(0.923879532511289,0.270598050073094,-0.270598050073094));
#23519=DIRECTION('',(0.,0.707106781186548,0.707106781186548));
#23520=DIRECTION('center_axis',(0.,0.707106781186548,0.707106781186548));
#23521=DIRECTION('ref_axis',(0.92387953251129,0.270598050073092,-0.270598050073092));
#23522=DIRECTION('center_axis',(0.707106781186547,0.500000000000001,-0.500000000000001));
#23523=DIRECTION('ref_axis',(-0.577350269189627,0.,-0.816496580927725));
#23524=DIRECTION('',(-0.577350269189627,0.816496580927725,-1.99733352710025E-16));
#23525=DIRECTION('center_axis',(0.,-0.707106781186547,0.707106781186548));
#23526=DIRECTION('ref_axis',(0.38268343236509,0.653281482438193,0.653281482438183));
#23527=DIRECTION('',(0.,0.707106781186547,-0.707106781186548));
#23528=DIRECTION('',(0.,-0.707106781186547,0.707106781186548));
#23529=DIRECTION('center_axis',(-0.577350269189627,0.816496580927725,-1.92296268638356E-16));
#23530=DIRECTION('ref_axis',(0.816496580927726,0.577350269189626,0.));
#23531=DIRECTION('',(0.577350269189627,-0.816496580927725,1.99733352710025E-16));
#23532=DIRECTION('center_axis',(-0.577350269189624,0.816496580927727,-2.55393481785316E-15));
#23533=DIRECTION('ref_axis',(0.707106781186548,0.5,0.5));
#23534=DIRECTION('center_axis',(0.,0.,1.));
#23535=DIRECTION('ref_axis',(1.,0.,0.));
#23536=DIRECTION('center_axis',(0.,-0.707106781186547,0.707106781186548));
#23537=DIRECTION('ref_axis',(0.923879532511285,0.270598050073101,0.270598050073101));
#23538=DIRECTION('center_axis',(0.707106781186547,0.500000000000001,0.500000000000001));
#23539=DIRECTION('ref_axis',(0.577350269189627,0.,-0.816496580927725));
#23540=DIRECTION('',(0.,-0.707106781186547,0.707106781186548));
#23541=DIRECTION('center_axis',(0.,0.707106781186547,-0.707106781186548));
#23542=DIRECTION('ref_axis',(0.923879532511286,0.270598050073098,0.270598050073103));
#23543=DIRECTION('center_axis',(0.,-0.707106781186548,0.707106781186548));
#23544=DIRECTION('ref_axis',(1.,0.,0.));
#23545=DIRECTION('center_axis',(0.707106781186547,-0.500000000000001,-0.500000000000001));
#23546=DIRECTION('ref_axis',(-0.577350269189627,0.,-0.816496580927725));
#23547=DIRECTION('',(0.,-0.707106781186548,0.707106781186547));
#23548=DIRECTION('center_axis',(1.,0.,0.));
#23549=DIRECTION('ref_axis',(0.,-1.,0.));
#23550=DIRECTION('center_axis',(-0.707106781186547,0.5,0.5));
#23551=DIRECTION('ref_axis',(-0.707106781186548,-0.5,-0.5));
#23552=DIRECTION('center_axis',(-0.707106781186547,-0.500000000000001,0.500000000000001));
#23553=DIRECTION('ref_axis',(0.707106781186549,-0.499999999999999,0.499999999999999));
#23554=DIRECTION('',(1.,0.,0.));
#23555=DIRECTION('center_axis',(-1.,0.,0.));
#23556=DIRECTION('ref_axis',(0.,-0.707106781186548,-0.707106781186548));
#23557=DIRECTION('',(-1.,0.,0.));
#23558=DIRECTION('center_axis',(0.,0.,1.));
#23559=DIRECTION('ref_axis',(1.,0.,0.));
#23560=DIRECTION('center_axis',(0.,-0.707106781186548,0.707106781186547));
#23561=DIRECTION('ref_axis',(0.382683432365089,-0.653281482438189,-0.653281482438189));
#23562=DIRECTION('center_axis',(0.,-0.707106781186547,0.707106781186548));
#23563=DIRECTION('ref_axis',(0.,-0.707106781186548,-0.707106781186547));
#23564=DIRECTION('',(1.,0.,0.));
#23565=DIRECTION('center_axis',(0.,0.707106781186547,-0.707106781186548));
#23566=DIRECTION('ref_axis',(0.923879532511285,0.270598050073101,0.270598050073101));
#23567=DIRECTION('',(0.,-0.707106781186548,-0.707106781186547));
#23568=DIRECTION('center_axis',(0.,0.707106781186547,-0.707106781186548));
#23569=DIRECTION('ref_axis',(0.923879532511289,-0.270598050073094,-0.270598050073094));
#23570=DIRECTION('center_axis',(0.,0.707106781186548,-0.707106781186547));
#23571=DIRECTION('ref_axis',(0.38268343236509,-0.653281482438183,-0.653281482438193));
#23572=DIRECTION('',(0.,0.707106781186548,-0.707106781186547));
#23573=DIRECTION('center_axis',(0.,-0.707106781186548,0.707106781186548));
#23574=DIRECTION('ref_axis',(0.,-0.707106781186548,-0.707106781186548));
#23575=DIRECTION('center_axis',(-0.0824635143087527,-0.971269669085139,
0.223237538785696));
#23576=DIRECTION('ref_axis',(0.336556770590777,-0.237981574738982,-0.91109511592054));
#23577=DIRECTION('center_axis',(1.,0.,0.));
#23578=DIRECTION('ref_axis',(0.,0.,-1.));
#23579=DIRECTION('center_axis',(1.,0.,0.));
#23580=DIRECTION('ref_axis',(0.,0.,-1.));
#23581=DIRECTION('',(-1.,0.,0.));
#23582=DIRECTION('center_axis',(-1.,0.,0.));
#23583=DIRECTION('ref_axis',(0.,0.,-1.));
#23584=DIRECTION('',(1.,0.,0.));
#23585=DIRECTION('center_axis',(0.,-0.707106781186547,-0.707106781186548));
#23586=DIRECTION('ref_axis',(0.,0.707106781186548,-0.707106781186547));
#23587=DIRECTION('',(-7.85046229341888E-17,0.707106781186548,-0.707106781186547));
#23588=DIRECTION('',(1.,0.,0.));
#23589=DIRECTION('',(0.,-0.707106781186548,0.707106781186547));
#23590=DIRECTION('center_axis',(0.,0.,1.));
#23591=DIRECTION('ref_axis',(1.,0.,0.));
#23592=DIRECTION('center_axis',(0.,-0.707106781186547,-0.707106781186548));
#23593=DIRECTION('ref_axis',(0.382683432365089,-0.653281482438189,0.653281482438189));
#23594=DIRECTION('center_axis',(1.,0.,0.));
#23595=DIRECTION('ref_axis',(0.,-1.,0.));
#23596=DIRECTION('center_axis',(0.,-0.707106781186548,0.707106781186548));
#23597=DIRECTION('ref_axis',(0.,-0.707106781186548,-0.707106781186548));
#23598=DIRECTION('center_axis',(-0.577350269189626,-0.816496580927726,-3.20493781063927E-16));
#23599=DIRECTION('ref_axis',(0.816496580927727,-0.577350269189625,0.));
#23600=DIRECTION('center_axis',(-7.85046229341888E-17,0.707106781186548,
-0.707106781186547));
#23601=DIRECTION('ref_axis',(0.382683432365086,-0.653281482438194,-0.653281482438185));
#23602=DIRECTION('',(-7.85046229341888E-17,0.707106781186548,-0.707106781186547));
#23603=DIRECTION('center_axis',(1.,0.,0.));
#23604=DIRECTION('ref_axis',(0.,-1.,0.));
#23605=DIRECTION('',(-1.,0.,0.));
#23606=DIRECTION('center_axis',(-1.,0.,0.));
#23607=DIRECTION('ref_axis',(0.,-1.,0.));
#23608=DIRECTION('center_axis',(0.,-0.707106781186547,-0.707106781186548));
#23609=DIRECTION('ref_axis',(0.38268343236509,-0.653281482438193,0.653281482438183));
#23610=DIRECTION('',(-3.92523114670944E-17,0.707106781186547,0.707106781186548));
#23611=DIRECTION('center_axis',(0.,-0.707106781186548,-0.707106781186548));
#23612=DIRECTION('ref_axis',(0.707106781186548,-0.5,0.5));
#23613=DIRECTION('',(0.,-0.707106781186547,-0.707106781186548));
#23614=DIRECTION('center_axis',(-0.577350269189626,-0.816496580927726,-3.20493781063927E-16));
#23615=DIRECTION('ref_axis',(0.816496580927726,-0.577350269189626,0.));
#23616=DIRECTION('',(0.577350269189626,0.816496580927726,3.51392638260461E-16));
#23617=DIRECTION('center_axis',(-0.577350269189628,-0.816496580927725,0.));
#23618=DIRECTION('ref_axis',(0.707106781186546,-0.500000000000001,-0.500000000000001));
#23619=DIRECTION('',(-0.577350269189626,-0.816496580927726,-3.23637062644832E-16));
#23620=DIRECTION('center_axis',(0.,-0.707106781186548,0.707106781186547));
#23621=DIRECTION('ref_axis',(0.923879532511289,-0.270598050073094,-0.270598050073094));
#23622=DIRECTION('center_axis',(0.,0.707106781186548,-0.707106781186548));
#23623=DIRECTION('ref_axis',(1.,0.,0.));
#23624=DIRECTION('',(0.,0.707106781186548,-0.707106781186547));
#23625=DIRECTION('',(0.,-0.707106781186548,0.707106781186547));
#23626=DIRECTION('center_axis',(0.,0.,1.));
#23627=DIRECTION('ref_axis',(1.,0.,0.));
#23628=DIRECTION('center_axis',(0.,-0.707106781186547,-0.707106781186548));
#23629=DIRECTION('ref_axis',(0.92387953251129,-0.270598050073093,0.270598050073093));
#23630=DIRECTION('center_axis',(0.707106781186547,-0.5,0.5));
#23631=DIRECTION('ref_axis',(0.577350269189626,0.,-0.816496580927726));
#23632=DIRECTION('',(0.,-0.707106781186547,-0.707106781186548));
#23633=DIRECTION('',(0.577350269189623,-5.15565607263847E-15,-0.816496580927728));
#23634=DIRECTION('center_axis',(0.,0.707106781186547,0.707106781186548));
#23635=DIRECTION('ref_axis',(0.923879532511287,-0.270598050073094,0.270598050073103));
#23636=DIRECTION('',(0.,0.707106781186547,0.707106781186548));
#23637=DIRECTION('center_axis',(0.,0.707106781186547,0.707106781186548));
#23638=DIRECTION('ref_axis',(0.923879532511286,-0.270598050073101,0.270598050073101));
#23639=DIRECTION('center_axis',(1.,0.,0.));
#23640=DIRECTION('ref_axis',(0.,0.,-1.));
#23641=DIRECTION('',(0.,0.707106781186547,-0.707106781186548));
#23642=DIRECTION('center_axis',(0.,0.,1.));
#23643=DIRECTION('ref_axis',(1.,0.,0.));
#23644=DIRECTION('center_axis',(1.,0.,0.));
#23645=DIRECTION('ref_axis',(0.,1.,0.));
#23646=DIRECTION('',(-1.,0.,0.));
#23647=DIRECTION('center_axis',(-1.,0.,0.));
#23648=DIRECTION('ref_axis',(0.,1.,0.));
#23649=DIRECTION('',(1.,0.,0.));
#23650=DIRECTION('center_axis',(0.,0.707106781186548,0.707106781186547));
#23651=DIRECTION('ref_axis',(0.,-0.707106781186547,0.707106781186548));
#23652=DIRECTION('',(0.,0.707106781186547,-0.707106781186548));
#23653=DIRECTION('',(-1.,0.,0.));
#23654=DIRECTION('',(0.,-0.707106781186547,0.707106781186548));
#23655=DIRECTION('',(-1.,0.,0.));
#23656=DIRECTION('center_axis',(1.,0.,0.));
#23657=DIRECTION('ref_axis',(0.,0.,1.));
#23658=DIRECTION('center_axis',(-0.707106781186547,-0.500000000000001,0.500000000000001));
#23659=DIRECTION('ref_axis',(0.707106781186549,-0.499999999999999,0.499999999999999));
#23660=DIRECTION('center_axis',(-0.707106781186552,-0.499999999999997,-0.499999999999997));
#23661=DIRECTION('ref_axis',(-0.707106781186543,0.500000000000003,0.500000000000003));
#23662=DIRECTION('center_axis',(0.,0.707106781186547,-0.707106781186548));
#23663=DIRECTION('ref_axis',(0.923879532511285,0.270598050073101,0.270598050073101));
#23664=DIRECTION('center_axis',(0.,0.707106781186548,-0.707106781186548));
#23665=DIRECTION('ref_axis',(0.707106781186552,0.499999999999996,0.499999999999996));
#23666=DIRECTION('',(0.,0.707106781186547,-0.707106781186548));
#23667=DIRECTION('center_axis',(0.,0.,1.));
#23668=DIRECTION('ref_axis',(1.,0.,0.));
#23669=DIRECTION('center_axis',(0.577350269189624,-7.66180445355954E-15,
-0.816496580927727));
#23670=DIRECTION('ref_axis',(0.707106781186552,0.499999999999996,0.499999999999996));
#23671=DIRECTION('center_axis',(-0.577350269189623,5.12790049702284E-15,
0.816496580927728));
#23672=DIRECTION('ref_axis',(0.816496580927727,0.,0.577350269189624));
#23673=DIRECTION('center_axis',(-0.577350269189629,-7.26118722722956E-15,
0.816496580927724));
#23674=DIRECTION('ref_axis',(0.707106781186548,-0.5,0.5));
#23675=DIRECTION('',(-0.577350269189623,5.12790049702284E-15,0.816496580927728));
#23676=DIRECTION('center_axis',(0.,-0.707106781186548,0.707106781186547));
#23677=DIRECTION('ref_axis',(0.,-0.707106781186547,-0.707106781186548));
#23678=DIRECTION('',(1.,0.,0.));
#23679=DIRECTION('',(0.,0.707106781186547,0.707106781186548));
#23680=DIRECTION('center_axis',(0.707106781186547,-0.5,-0.5));
#23681=DIRECTION('ref_axis',(-0.577350269189626,0.,-0.816496580927726));
#23682=DIRECTION('center_axis',(0.,-0.707106781186547,0.707106781186548));
#23683=DIRECTION('ref_axis',(0.382683432365095,0.653281482438189,0.653281482438184));
#23684=DIRECTION('center_axis',(6.31716887673553E-15,0.707106781186543,
-0.707106781186552));
#23685=DIRECTION('ref_axis',(0.,0.707106781186552,0.707106781186543));
#23686=DIRECTION('',(7.85046229341892E-17,0.707106781186547,-0.707106781186548));
#23687=DIRECTION('center_axis',(0.0824635143087527,-0.971269669085139,0.223237538785696));
#23688=DIRECTION('ref_axis',(0.336556770590777,0.23798157473898,0.91109511592054));
#23689=DIRECTION('center_axis',(1.,0.,0.));
#23690=DIRECTION('ref_axis',(0.,0.,1.));
#23691=DIRECTION('center_axis',(1.,0.,0.));
#23692=DIRECTION('ref_axis',(0.,0.,1.));
#23693=DIRECTION('center_axis',(-1.,0.,0.));
#23694=DIRECTION('ref_axis',(0.,0.,1.));
#23695=DIRECTION('center_axis',(0.707106781186552,0.499999999999997,0.499999999999997));
#23696=DIRECTION('ref_axis',(0.577350269189621,0.,-0.816496580927729));
#23697=DIRECTION('center_axis',(1.,0.,0.));
#23698=DIRECTION('ref_axis',(0.,0.,-1.));
#23699=DIRECTION('center_axis',(-1.,0.,0.));
#23700=DIRECTION('ref_axis',(0.,0.707106781186548,-0.707106781186548));
#23701=DIRECTION('',(-1.,0.,0.));
#23702=DIRECTION('center_axis',(-1.,0.,0.));
#23703=DIRECTION('ref_axis',(0.,0.,-1.));
#23704=DIRECTION('',(1.,0.,0.));
#23705=DIRECTION('center_axis',(0.,0.707106781186547,0.707106781186548));
#23706=DIRECTION('ref_axis',(0.382683432365089,0.653281482438191,-0.653281482438186));
#23707=DIRECTION('center_axis',(0.,0.707106781186548,0.707106781186548));
#23708=DIRECTION('ref_axis',(0.707106781186544,0.500000000000003,-0.500000000000003));
#23709=DIRECTION('',(0.,0.707106781186547,0.707106781186548));
#23710=DIRECTION('center_axis',(0.,-0.707106781186548,-0.707106781186548));
#23711=DIRECTION('ref_axis',(0.,0.707106781186548,-0.707106781186548));
#23712=DIRECTION('',(0.,-0.707106781186547,-0.707106781186548));
#23713=DIRECTION('center_axis',(0.,0.,1.));
#23714=DIRECTION('ref_axis',(1.,0.,0.));
#23715=DIRECTION('center_axis',(0.,-0.707106781186548,0.707106781186548));
#23716=DIRECTION('ref_axis',(0.382683432365089,0.653281482438189,0.653281482438189));
#23717=DIRECTION('center_axis',(-0.577350269189627,0.816496580927725,3.84592537276713E-16));
#23718=DIRECTION('ref_axis',(0.816496580927727,0.577350269189625,0.));
#23719=DIRECTION('center_axis',(1.,0.,0.));
#23720=DIRECTION('ref_axis',(0.,1.,0.));
#23721=DIRECTION('center_axis',(0.,-0.707106781186548,-0.707106781186548));
#23722=DIRECTION('ref_axis',(0.,0.707106781186548,-0.707106781186548));
#23723=DIRECTION('',(0.,0.707106781186547,-0.707106781186547));
#23724=DIRECTION('',(1.,0.,0.));
#23725=DIRECTION('',(0.,-0.707106781186548,0.707106781186548));
#23726=DIRECTION('center_axis',(0.707106781186547,0.500000000000001,-0.5));
#23727=DIRECTION('ref_axis',(-0.577350269189626,0.,-0.816496580927726));
#23728=DIRECTION('',(-0.577350269189627,0.816496580927725,3.43955554188792E-16));
#23729=DIRECTION('',(0.,0.707106781186547,0.707106781186548));
#23730=DIRECTION('',(0.577350269189627,-4.76446869105127E-16,0.816496580927725));
#23731=DIRECTION('center_axis',(-0.577350269189627,4.48691293489498E-16,
-0.816496580927725));
#23732=DIRECTION('ref_axis',(0.816496580927726,0.,-0.577350269189626));
#23733=DIRECTION('center_axis',(0.577350269189626,2.55393481785319E-15,
0.816496580927726));
#23734=DIRECTION('ref_axis',(0.707106781186548,-0.5,-0.5));
#23735=DIRECTION('center_axis',(-0.577350269189625,-3.8559408034254E-15,
-0.816496580927727));
#23736=DIRECTION('ref_axis',(0.707106781186547,0.5,-0.5));
#23737=DIRECTION('',(-0.577350269189627,4.20935717873869E-16,-0.816496580927725));
#23738=DIRECTION('center_axis',(1.,0.,0.));
#23739=DIRECTION('ref_axis',(0.,-1.,0.));
#23740=DIRECTION('center_axis',(0.,0.707106781186548,-0.707106781186548));
#23741=DIRECTION('ref_axis',(0.382683432365087,-0.653281482438189,-0.653281482438189));
#23742=DIRECTION('center_axis',(0.,-0.707106781186547,-0.707106781186548));
#23743=DIRECTION('ref_axis',(0.923879532511286,0.270598050073102,-0.270598050073097));
#23744=DIRECTION('center_axis',(0.,-0.707106781186548,-0.707106781186548));
#23745=DIRECTION('ref_axis',(0.707106781186548,0.5,-0.5));
#23746=DIRECTION('',(0.,-0.707106781186547,-0.707106781186548));
#23747=DIRECTION('center_axis',(0.,0.707106781186548,0.707106781186548));
#23748=DIRECTION('ref_axis',(1.,0.,0.));
#23749=DIRECTION('center_axis',(0.,0.,1.));
#23750=DIRECTION('ref_axis',(1.,0.,0.));
#23751=DIRECTION('center_axis',(0.,0.707106781186548,-0.707106781186548));
#23752=DIRECTION('ref_axis',(0.92387953251129,-0.270598050073092,-0.270598050073092));
#23753=DIRECTION('center_axis',(-0.577350269189627,0.816496580927725,3.84592537276713E-16));
#23754=DIRECTION('ref_axis',(0.816496580927726,0.577350269189626,0.));
#23755=DIRECTION('',(0.577350269189627,-0.816496580927725,-4.27222281035679E-16));
#23756=DIRECTION('center_axis',(-0.577350269189625,0.816496580927726,2.55393481785319E-15));
#23757=DIRECTION('ref_axis',(0.707106781186549,0.499999999999999,0.499999999999999));
#23758=DIRECTION('center_axis',(0.,0.,1.));
#23759=DIRECTION('ref_axis',(1.,0.,0.));
#23760=DIRECTION('center_axis',(0.,0.707106781186548,-0.707106781186548));
#23761=DIRECTION('ref_axis',(0.923879532511286,0.270598050073101,0.270598050073101));
#23762=DIRECTION('center_axis',(0.,0.707106781186548,-0.707106781186548));
#23763=DIRECTION('ref_axis',(0.382683432365087,-0.653281482438187,-0.653281482438192));
#23764=DIRECTION('',(0.,-0.707106781186547,0.707106781186547));
#23765=DIRECTION('center_axis',(3.12791857003411E-15,0.70710678118655,-0.707106781186545));
#23766=DIRECTION('ref_axis',(0.707106781186547,-0.5,-0.5));
#23767=DIRECTION('center_axis',(0.707106781186547,-0.500000000000001,-0.500000000000001));
#23768=DIRECTION('ref_axis',(-0.577350269189627,0.,-0.816496580927725));
#23769=DIRECTION('',(0.,0.707106781186548,-0.707106781186548));
#23770=DIRECTION('',(0.577350269189627,0.816496580927725,-4.1978519696401E-16));
#23771=DIRECTION('center_axis',(0.,-0.707106781186548,0.707106781186548));
#23772=DIRECTION('ref_axis',(0.923879532511289,-0.270598050073094,-0.270598050073094));
#23773=DIRECTION('',(0.,-0.707106781186548,0.707106781186548));
#23774=DIRECTION('center_axis',(0.,-0.707106781186548,0.707106781186548));
#23775=DIRECTION('ref_axis',(0.92387953251129,-0.270598050073092,-0.270598050073092));
#23776=DIRECTION('center_axis',(1.,0.,0.));
#23777=DIRECTION('ref_axis',(0.,0.,-1.));
#23778=DIRECTION('',(0.,0.707106781186548,-0.707106781186548));
#23779=DIRECTION('',(0.,0.707106781186548,0.707106781186547));
#23780=DIRECTION('center_axis',(0.,0.707106781186548,-0.707106781186548));
#23781=DIRECTION('ref_axis',(0.923879532511287,0.270598050073094,0.270598050073103));
#23782=DIRECTION('',(0.,-0.707106781186548,0.707106781186548));
#23783=DIRECTION('center_axis',(0.,-0.707106781186548,0.707106781186548));
#23784=DIRECTION('ref_axis',(0.923879532511288,0.270598050073101,0.270598050073092));
#23785=DIRECTION('center_axis',(0.707106781186547,0.500000000000001,0.500000000000001));
#23786=DIRECTION('ref_axis',(0.577350269189627,0.,-0.816496580927725));
#23787=DIRECTION('',(0.,0.707106781186547,-0.707106781186547));
#23788=DIRECTION('',(-0.577350269189627,4.4010368850797E-16,0.816496580927725));
#23789=DIRECTION('center_axis',(0.,-0.707106781186548,0.707106781186548));
#23790=DIRECTION('ref_axis',(0.38268343236509,0.653281482438188,0.653281482438188));
#23791=DIRECTION('',(0.,-0.707106781186547,0.707106781186547));
#23792=DIRECTION('center_axis',(0.,0.707106781186548,-0.707106781186548));
#23793=DIRECTION('ref_axis',(-2.22044604925029E-15,0.707106781186548,0.707106781186548));
#23794=DIRECTION('center_axis',(0.,0.707106781186547,0.707106781186548));
#23795=DIRECTION('ref_axis',(0.707106781186547,0.5,-0.5));
#23796=DIRECTION('center_axis',(0.,-0.707106781186548,-0.707106781186548));
#23797=DIRECTION('ref_axis',(0.,0.707106781186548,-0.707106781186548));
#23798=DIRECTION('',(0.,-0.707106781186547,-0.707106781186548));
#23799=DIRECTION('center_axis',(0.707106781186547,-0.5,-0.5));
#23800=DIRECTION('ref_axis',(0.707106781186548,0.499999999999999,0.500000000000001));
#23801=DIRECTION('',(0.,0.707106781186547,0.707106781186548));
#23802=DIRECTION('center_axis',(1.,0.,0.));
#23803=DIRECTION('ref_axis',(0.,1.,0.));
#23804=DIRECTION('',(1.,0.,0.));
#23805=DIRECTION('center_axis',(-1.,0.,0.));
#23806=DIRECTION('ref_axis',(0.,0.707106781186548,0.707106781186548));
#23807=DIRECTION('',(-1.,0.,0.));
#23808=DIRECTION('center_axis',(-1.,0.,0.));
#23809=DIRECTION('ref_axis',(0.,1.,0.));
#23810=DIRECTION('center_axis',(0.,0.,1.));
#23811=DIRECTION('ref_axis',(1.,0.,0.));
#23812=DIRECTION('center_axis',(0.,0.707106781186548,-0.707106781186548));
#23813=DIRECTION('ref_axis',(0.707106781186548,0.5,0.5));
#23814=DIRECTION('center_axis',(1.,0.,0.));
#23815=DIRECTION('ref_axis',(0.,0.,-1.));
#23816=DIRECTION('',(0.,0.707106781186548,-0.707106781186548));
#23817=DIRECTION('',(0.,0.707106781186548,0.707106781186547));
#23818=DIRECTION('',(0.,-0.707106781186548,0.707106781186548));
#23819=DIRECTION('center_axis',(0.,-0.707106781186548,0.707106781186548));
#23820=DIRECTION('ref_axis',(0.707106781186547,0.5,0.5));
#23821=DIRECTION('',(0.,-0.707106781186548,0.707106781186548));
#23822=DIRECTION('center_axis',(0.,0.707106781186548,-0.707106781186548));
#23823=DIRECTION('ref_axis',(0.,0.707106781186548,0.707106781186548));
#23824=DIRECTION('center_axis',(0.,0.707106781186548,0.707106781186548));
#23825=DIRECTION('ref_axis',(0.,-0.707106781186548,0.707106781186548));
#23826=DIRECTION('',(0.,0.707106781186548,-0.707106781186548));
#23827=DIRECTION('',(-1.,0.,0.));
#23828=DIRECTION('center_axis',(0.,-1.,0.));
#23829=DIRECTION('ref_axis',(0.577350269189629,0.,0.816496580927724));
#23830=DIRECTION('center_axis',(1.,0.,0.));
#23831=DIRECTION('ref_axis',(0.,0.,1.));
#23832=DIRECTION('center_axis',(0.,0.707106781186548,0.707106781186547));
#23833=DIRECTION('ref_axis',(0.707106781186548,-0.5,0.5));
#23834=DIRECTION('center_axis',(0.,0.707106781186548,-0.707106781186547));
#23835=DIRECTION('ref_axis',(0.,0.707106781186547,0.707106781186548));
#23836=DIRECTION('',(0.,-0.707106781186547,-0.707106781186548));
#23837=DIRECTION('',(-1.,0.,0.));
#23838=DIRECTION('center_axis',(1.,0.,0.));
#23839=DIRECTION('ref_axis',(0.,0.,1.));
#23840=DIRECTION('center_axis',(-1.,0.,0.));
#23841=DIRECTION('ref_axis',(0.,0.,1.));
#23842=DIRECTION('',(1.,0.,0.));
#23843=DIRECTION('center_axis',(0.,-0.707106781186548,-0.707106781186547));
#23844=DIRECTION('ref_axis',(0.707106781186547,-0.5,0.5));
#23845=DIRECTION('',(0.,-0.707106781186548,-0.707106781186547));
#23846=DIRECTION('center_axis',(0.707106781186547,-0.5,-0.5));
#23847=DIRECTION('ref_axis',(0.707106781186548,0.500000000000001,0.499999999999999));
#23848=DIRECTION('center_axis',(0.577350269189627,-3.84592537276713E-16,
-0.816496580927725));
#23849=DIRECTION('ref_axis',(0.816496580927726,0.,0.577350269189626));
#23850=DIRECTION('center_axis',(-0.577350269189625,3.85594080342536E-15,
0.816496580927727));
#23851=DIRECTION('ref_axis',(0.707106781186547,-0.5,0.5));
#23852=DIRECTION('center_axis',(-0.57735026918963,7.26118722722964E-15,
0.816496580927723));
#23853=DIRECTION('ref_axis',(0.707106781186547,-0.499999999999992,0.500000000000009));
#23854=DIRECTION('',(0.577350269189627,-3.56836961661084E-16,-0.816496580927725));
#23855=DIRECTION('center_axis',(0.,0.707106781186548,0.707106781186547));
#23856=DIRECTION('ref_axis',(0.923879532511287,-0.270598050073094,0.270598050073103));
#23857=DIRECTION('center_axis',(0.,0.707106781186548,0.707106781186548));
#23858=DIRECTION('ref_axis',(0.707106781186546,-0.500000000000001,0.500000000000001));
#23859=DIRECTION('center_axis',(0.,-0.707106781186548,-0.707106781186548));
#23860=DIRECTION('ref_axis',(1.,0.,0.));
#23861=DIRECTION('',(0.,-0.707106781186548,-0.707106781186547));
#23862=DIRECTION('center_axis',(0.,0.,1.));
#23863=DIRECTION('ref_axis',(1.,0.,0.));
#23864=DIRECTION('center_axis',(0.577350269189627,0.816496580927725,-1.25192883228098E-15));
#23865=DIRECTION('ref_axis',(0.707106781186547,-0.5,0.5));
#23866=DIRECTION('center_axis',(-0.577350269189627,-0.816496580927725,4.48691293489498E-16));
#23867=DIRECTION('ref_axis',(0.816496580927725,-0.577350269189628,0.));
#23868=DIRECTION('center_axis',(0.577350269189625,0.816496580927727,-1.25192883228096E-15));
#23869=DIRECTION('ref_axis',(0.707106781186541,-0.499999999999993,0.500000000000016));
#23870=DIRECTION('',(-0.577350269189627,-0.816496580927725,4.75296348195268E-16));
#23871=DIRECTION('center_axis',(0.,0.,1.));
#23872=DIRECTION('ref_axis',(1.,0.,0.));
#23873=DIRECTION('center_axis',(0.707106781186547,-0.5,0.500000000000001));
#23874=DIRECTION('ref_axis',(0.577350269189627,0.,-0.816496580927725));
#23875=DIRECTION('',(0.,0.707106781186548,0.707106781186547));
#23876=DIRECTION('center_axis',(0.,0.707106781186548,0.707106781186548));
#23877=DIRECTION('ref_axis',(0.,-0.707106781186548,0.707106781186548));
#23878=DIRECTION('',(1.,0.,0.));
#23879=DIRECTION('',(-1.,0.,0.));
#23880=DIRECTION('center_axis',(1.,0.,0.));
#23881=DIRECTION('ref_axis',(0.,1.,0.));
#23882=DIRECTION('center_axis',(1.,0.,0.));
#23883=DIRECTION('ref_axis',(0.,0.,1.));
#23884=DIRECTION('center_axis',(-1.,0.,0.));
#23885=DIRECTION('ref_axis',(0.,-0.707106781186548,0.707106781186548));
#23886=DIRECTION('',(1.,0.,0.));
#23887=DIRECTION('center_axis',(-0.0824635143087543,-0.971269669085137,
-0.223237538785703));
#23888=DIRECTION('ref_axis',(0.336556770590775,-0.237981574738988,0.911095115920539));
#23889=DIRECTION('center_axis',(0.,0.707106781186548,0.707106781186547));
#23890=DIRECTION('ref_axis',(0.382683432365091,-0.653281482438184,0.653281482438192));
#23891=DIRECTION('center_axis',(0.,-0.707106781186548,-0.707106781186547));
#23892=DIRECTION('ref_axis',(0.38268343236509,-0.653281482438183,0.653281482438193));
#23893=DIRECTION('',(0.,-0.707106781186548,-0.707106781186547));
#23894=DIRECTION('center_axis',(-8.89310181676358E-15,0.707106781186548,
0.707106781186548));
#23895=DIRECTION('ref_axis',(0.,-0.707106781186548,0.707106781186548));
#23896=DIRECTION('center_axis',(0.,-0.707106781186547,0.707106781186548));
#23897=DIRECTION('ref_axis',(0.,-0.707106781186548,-0.707106781186547));
#23898=DIRECTION('',(0.,0.707106781186548,0.707106781186547));
#23899=DIRECTION('',(-1.,0.,0.));
#23900=DIRECTION('center_axis',(0.,0.,1.));
#23901=DIRECTION('ref_axis',(1.,0.,0.));
#23902=DIRECTION('center_axis',(1.,0.,0.));
#23903=DIRECTION('ref_axis',(0.,-1.,0.));
#23904=DIRECTION('center_axis',(1.,0.,0.));
#23905=DIRECTION('ref_axis',(0.,-1.,0.));
#23906=DIRECTION('center_axis',(-1.,0.,0.));
#23907=DIRECTION('ref_axis',(0.,-1.,0.));
#23908=DIRECTION('center_axis',(0.,-0.707106781186547,0.707106781186548));
#23909=DIRECTION('ref_axis',(0.923879532511289,-0.270598050073094,-0.270598050073094));
#23910=DIRECTION('',(0.,0.707106781186547,-0.707106781186548));
#23911=DIRECTION('center_axis',(0.,-0.707106781186548,0.707106781186548));
#23912=DIRECTION('ref_axis',(0.707106781186548,-0.5,-0.5));
#23913=DIRECTION('',(0.,-0.707106781186547,0.707106781186548));
#23914=DIRECTION('center_axis',(0.,-0.707106781186547,0.707106781186548));
#23915=DIRECTION('ref_axis',(0.923879532511289,-0.270598050073094,-0.270598050073094));
#23916=DIRECTION('center_axis',(-0.577350269189626,-1.92296268638356E-16,
-0.816496580927726));
#23917=DIRECTION('ref_axis',(0.816496580927725,0.,-0.577350269189628));
#23918=DIRECTION('center_axis',(0.627963030199555,-0.769094500660425,0.118979333316691));
#23919=DIRECTION('ref_axis',(-0.325057583671868,-0.398112608509064,-0.857813451890046));
#23920=DIRECTION('',(0.577350269189626,1.64540693022727E-16,0.816496580927726));
#23921=DIRECTION('center_axis',(-0.577350269189631,2.10324043823204E-15,
-0.816496580927722));
#23922=DIRECTION('ref_axis',(0.707106781186544,0.500000000000003,-0.500000000000003));
#23923=DIRECTION('',(-0.577350269189626,-1.92296268638356E-16,-0.816496580927726));
#23924=DIRECTION('center_axis',(0.888073833977113,0.,0.459700843380987));
#23925=DIRECTION('ref_axis',(0.459700843380987,-8.83987568720673E-17,-0.888073833977113));
#23926=DIRECTION('center_axis',(0.,0.,1.));
#23927=DIRECTION('ref_axis',(1.,0.,0.));
#23928=DIRECTION('center_axis',(0.,-0.707106781186548,-0.707106781186548));
#23929=DIRECTION('ref_axis',(0.923879532511288,0.270598050073101,-0.270598050073092));
#23930=DIRECTION('center_axis',(1.,0.,0.));
#23931=DIRECTION('ref_axis',(0.,0.,-1.));
#23932=DIRECTION('',(0.,-0.707106781186548,-0.707106781186548));
#23933=DIRECTION('',(0.,0.707106781186547,-0.707106781186548));
#23934=DIRECTION('',(0.,0.707106781186548,0.707106781186547));
#23935=DIRECTION('center_axis',(0.,-0.707106781186548,-0.707106781186548));
#23936=DIRECTION('ref_axis',(0.923879532511287,0.270598050073094,-0.270598050073103));
#23937=DIRECTION('',(0.,0.707106781186548,0.707106781186548));
#23938=DIRECTION('center_axis',(-0.499999999999998,0.853553390593274,0.146446609406731));
#23939=DIRECTION('ref_axis',(0.500000000000003,0.146446609406722,0.853553390593273));
#23940=DIRECTION('center_axis',(0.,0.,1.));
#23941=DIRECTION('ref_axis',(0.,-1.,0.));
#23942=DIRECTION('center_axis',(0.707106781186547,0.5,-0.5));
#23943=DIRECTION('ref_axis',(-0.577350269189626,0.,-0.816496580927726));
#23944=DIRECTION('',(0.,-0.707106781186548,-0.707106781186548));
#23945=DIRECTION('',(-0.707106781186548,0.5,-0.5));
#23946=DIRECTION('center_axis',(0.,0.707106781186548,0.707106781186548));
#23947=DIRECTION('ref_axis',(0.382683432365088,0.653281482438189,-0.653281482438189));
#23948=DIRECTION('center_axis',(-0.707106781186547,-0.500000000000001,-0.500000000000001));
#23949=DIRECTION('ref_axis',(0.707106781186549,-0.499999999999999,-0.499999999999999));
#23950=DIRECTION('',(0.,0.707106781186548,0.707106781186548));
#23951=DIRECTION('center_axis',(0.,-0.707106781186548,-0.707106781186548));
#23952=DIRECTION('ref_axis',(0.,0.707106781186548,-0.707106781186548));
#23953=DIRECTION('center_axis',(1.,0.,0.));
#23954=DIRECTION('ref_axis',(0.,0.,-1.));
#23955=DIRECTION('center_axis',(-0.707106781186547,0.5,0.5));
#23956=DIRECTION('ref_axis',(-0.707106781186548,-0.5,-0.5));
#23957=DIRECTION('',(-1.,0.,0.));
#23958=DIRECTION('center_axis',(-1.,0.,0.));
#23959=DIRECTION('ref_axis',(0.,0.,-1.));
#23960=DIRECTION('',(1.,0.,0.));
#23961=DIRECTION('center_axis',(7.85046229341889E-17,-0.707106781186548,
-0.707106781186547));
#23962=DIRECTION('ref_axis',(0.382683432365091,-0.653281482438185,0.65328148243819));
#23963=DIRECTION('center_axis',(0.,-0.707106781186548,-0.707106781186548));
#23964=DIRECTION('ref_axis',(0.707106781186548,-0.5,0.5));
#23965=DIRECTION('',(7.85046229341889E-17,-0.707106781186548,-0.707106781186547));
#23966=DIRECTION('center_axis',(-1.77862036335272E-14,0.707106781186548,
0.707106781186548));
#23967=DIRECTION('ref_axis',(-2.22044604925032E-15,-0.707106781186548,0.707106781186548));
#23968=DIRECTION('',(-7.85046229341889E-17,0.707106781186548,0.707106781186547));
#23969=DIRECTION('center_axis',(0.,0.,1.));
#23970=DIRECTION('ref_axis',(1.,0.,0.));
#23971=DIRECTION('center_axis',(7.85046229341887E-17,0.707106781186547,
-0.707106781186548));
#23972=DIRECTION('ref_axis',(0.382683432365087,-0.653281482438189,-0.653281482438189));
#23973=DIRECTION('center_axis',(-0.577350269189626,-0.816496580927726,-1.02558009940457E-15));
#23974=DIRECTION('ref_axis',(0.816496580927725,-0.577350269189627,-8.88178419700125E-15));
#23975=DIRECTION('center_axis',(1.,0.,0.));
#23976=DIRECTION('ref_axis',(0.,-1.,0.));
#23977=DIRECTION('center_axis',(0.,-1.,0.));
#23978=DIRECTION('ref_axis',(0.505449465124417,0.,0.862856209461021));
#23979=DIRECTION('center_axis',(7.85046229341889E-17,-0.707106781186547,
0.707106781186548));
#23980=DIRECTION('ref_axis',(0.382683432365089,0.653281482438189,0.653281482438189));
#23981=DIRECTION('center_axis',(1.,0.,0.));
#23982=DIRECTION('ref_axis',(0.,0.,1.));
#23983=DIRECTION('center_axis',(-0.577350269189627,2.56395024851142E-16,
0.816496580927725));
#23984=DIRECTION('ref_axis',(0.816496580927725,0.,0.577350269189628));
#23985=DIRECTION('center_axis',(1.,0.,0.));
#23986=DIRECTION('ref_axis',(0.,0.,1.));
#23987=DIRECTION('',(-1.,0.,0.));
#23988=DIRECTION('center_axis',(-1.,0.,0.));
#23989=DIRECTION('ref_axis',(0.,0.,1.));
#23990=DIRECTION('',(1.,0.,0.));
#23991=DIRECTION('center_axis',(7.85046229341889E-17,-0.707106781186547,
0.707106781186548));
#23992=DIRECTION('ref_axis',(0.38268343236509,0.653281482438188,0.653281482438188));
#23993=DIRECTION('',(-7.85046229341889E-17,0.707106781186547,-0.707106781186548));
#23994=DIRECTION('center_axis',(-7.85046229341889E-17,0.707106781186547,
-0.707106781186548));
#23995=DIRECTION('ref_axis',(0.382683432365089,0.653281482438189,0.653281482438189));
#23996=DIRECTION('',(7.85046229341889E-17,-0.707106781186547,0.707106781186548));
#23997=DIRECTION('center_axis',(-0.577350269189627,2.56395024851142E-16,
0.816496580927725));
#23998=DIRECTION('ref_axis',(0.816496580927726,0.,0.577350269189626));
#23999=DIRECTION('',(0.577350269189627,-2.28639449235513E-16,-0.816496580927725));
#24000=DIRECTION('center_axis',(-0.577350269189627,-1.25192883228098E-15,
0.816496580927725));
#24001=DIRECTION('ref_axis',(0.707106781186547,-0.5,0.5));
#24002=DIRECTION('',(-0.577350269189627,3.119061760824E-16,0.816496580927725));
#24003=DIRECTION('center_axis',(0.707106781186547,-0.500000000000001,0.500000000000001));
#24004=DIRECTION('ref_axis',(0.577350269189627,0.,-0.816496580927725));
#24005=DIRECTION('',(-0.577350269189626,-0.816496580927726,-9.91229679478456E-16));
#24006=DIRECTION('',(0.,-0.707106781186548,-0.707106781186547));
#24007=DIRECTION('center_axis',(-0.577350269189626,-0.816496580927726,-1.02558009940457E-15));
#24008=DIRECTION('ref_axis',(0.816496580927728,-0.577350269189623,-1.02558009940457E-14));
#24009=DIRECTION('',(0.577350269189626,0.816496580927726,1.01898525509409E-15));
#24010=DIRECTION('center_axis',(-0.577350269189626,-0.816496580927726,4.65717525608515E-15));
#24011=DIRECTION('ref_axis',(0.707106781186545,-0.500000000000002,-0.500000000000002));
#24012=DIRECTION('center_axis',(0.,-0.707106781186547,0.707106781186548));
#24013=DIRECTION('ref_axis',(0.923879532511289,-0.270598050073097,-0.270598050073093));
#24014=DIRECTION('center_axis',(0.,-0.707106781186548,0.707106781186548));
#24015=DIRECTION('ref_axis',(0.707106781186549,-0.499999999999999,-0.499999999999999));
#24016=DIRECTION('',(0.,-0.707106781186547,0.707106781186548));
#24017=DIRECTION('center_axis',(0.,0.707106781186548,-0.707106781186548));
#24018=DIRECTION('ref_axis',(1.,0.,0.));
#24019=DIRECTION('',(-3.92523114670944E-17,0.707106781186547,-0.707106781186548));
#24020=DIRECTION('center_axis',(0.,0.,1.));
#24021=DIRECTION('ref_axis',(1.,0.,0.));
#24022=DIRECTION('center_axis',(0.577350269189626,1.30200598557221E-15,
0.816496580927726));
#24023=DIRECTION('ref_axis',(0.707106781186548,-0.5,-0.5));
#24024=DIRECTION('center_axis',(0.,-0.707106781186548,-0.707106781186547));
#24025=DIRECTION('ref_axis',(0.923879532511286,0.270598050073101,-0.270598050073101));
#24026=DIRECTION('center_axis',(0.,0.,1.));
#24027=DIRECTION('ref_axis',(1.,0.,0.));
#24028=DIRECTION('center_axis',(0.,-0.707106781186548,-0.707106781186547));
#24029=DIRECTION('ref_axis',(0.923879532511288,-0.270598050073101,0.270598050073092));
#24030=DIRECTION('center_axis',(0.577350269189626,1.73066641774521E-15,
0.816496580927726));
#24031=DIRECTION('ref_axis',(0.707106781186549,-0.499999999999999,-0.499999999999999));
#24032=DIRECTION('center_axis',(0.673887338679049,-0.262323811637645,0.690696802233777));
#24033=DIRECTION('ref_axis',(0.214186495298063,-0.825340061942894,-0.522434615415204));
#24034=DIRECTION('',(0.577350269189626,1.73066641774521E-15,0.816496580927726));
#24035=DIRECTION('',(-0.577350269189626,-1.73066641774521E-15,-0.816496580927726));
#24036=DIRECTION('center_axis',(0.627963030199553,0.769094500660428,0.118979333316688));
#24037=DIRECTION('ref_axis',(-0.32505758367187,0.398112608509061,-0.857813451890046));
#24038=DIRECTION('center_axis',(0.,0.707106781186548,0.707106781186547));
#24039=DIRECTION('ref_axis',(0.923879532511287,-0.270598050073094,0.270598050073103));
#24040=DIRECTION('',(0.,0.707106781186548,0.707106781186547));
#24041=DIRECTION('center_axis',(0.,-0.707106781186548,-0.707106781186548));
#24042=DIRECTION('ref_axis',(1.,0.,0.));
#24043=DIRECTION('center_axis',(1.,0.,0.));
#24044=DIRECTION('ref_axis',(0.,0.,-1.));
#24045=DIRECTION('',(0.,-0.707106781186548,-0.707106781186547));
#24046=DIRECTION('',(0.,0.707106781186547,-0.707106781186548));
#24047=DIRECTION('center_axis',(0.,-0.707106781186548,-0.707106781186547));
#24048=DIRECTION('ref_axis',(0.923879532511287,0.270598050073094,-0.270598050073103));
#24049=DIRECTION('',(0.,0.707106781186548,0.707106781186547));
#24050=DIRECTION('center_axis',(0.,0.707106781186548,0.707106781186547));
#24051=DIRECTION('ref_axis',(0.92387953251129,0.270598050073093,-0.270598050073093));
#24052=DIRECTION('center_axis',(0.707106781186546,0.5,-0.500000000000001));
#24053=DIRECTION('ref_axis',(-0.577350269189627,0.,-0.816496580927725));
#24054=DIRECTION('',(0.,-0.707106781186548,-0.707106781186547));
#24055=DIRECTION('',(-0.577350269189627,0.816496580927725,-2.75562995485243E-16));
#24056=DIRECTION('center_axis',(-0.707106781186549,0.499999999999999,-0.499999999999999));
#24057=DIRECTION('ref_axis',(0.707106781186548,0.5,-0.5));
#24058=DIRECTION('center_axis',(0.382683432365087,-0.653281482438189,0.653281482438189));
#24059=DIRECTION('ref_axis',(0.923879532511288,0.270598050073096,-0.270598050073097));
#24060=DIRECTION('center_axis',(-0.707106781186547,0.5,-0.5));
#24061=DIRECTION('ref_axis',(0.707106781186546,0.500000000000001,-0.500000000000001));
#24062=DIRECTION('center_axis',(7.85046229341887E-17,0.707106781186547,
-0.707106781186548));
#24063=DIRECTION('ref_axis',(0.382683432365088,-0.653281482438189,-0.653281482438189));
#24064=DIRECTION('',(7.85046229341887E-17,0.707106781186547,-0.707106781186548));
#24065=DIRECTION('',(-7.85046229341887E-17,-0.707106781186547,0.707106781186548));
#24066=DIRECTION('center_axis',(0.707106781186548,-0.5,-0.5));
#24067=DIRECTION('ref_axis',(-0.577350269189626,0.,-0.816496580927726));
#24068=DIRECTION('center_axis',(1.,0.,0.));
#24069=DIRECTION('ref_axis',(0.,-1.,0.));
#24070=DIRECTION('',(-1.,0.,0.));
#24071=DIRECTION('center_axis',(-1.,0.,0.));
#24072=DIRECTION('ref_axis',(0.,-1.,0.));
#24073=DIRECTION('',(1.,0.,0.));
#24074=DIRECTION('center_axis',(0.,-0.707106781186547,0.707106781186548));
#24075=DIRECTION('ref_axis',(0.,-0.707106781186548,-0.707106781186547));
#24076=DIRECTION('',(0.,0.707106781186548,0.707106781186547));
#24077=DIRECTION('center_axis',(1.,0.,0.));
#24078=DIRECTION('ref_axis',(0.,0.,-1.));
#24079=DIRECTION('center_axis',(-1.,0.,0.));
#24080=DIRECTION('ref_axis',(0.,0.707106781186548,-0.707106781186548));
#24081=DIRECTION('',(-1.,0.,0.));
#24082=DIRECTION('center_axis',(-0.707106781186547,0.5,0.5));
#24083=DIRECTION('ref_axis',(-0.707106781186548,-0.5,-0.5));
#24084=DIRECTION('',(1.,0.,0.));
#24085=DIRECTION('center_axis',(0.0824635143087527,-0.971269669085139,-0.223237538785696));
#24086=DIRECTION('ref_axis',(0.336556770590777,0.237981574738982,-0.91109511592054));
#24087=DIRECTION('center_axis',(0.,-0.707106781186548,-0.707106781186547));
#24088=DIRECTION('ref_axis',(0.382683432365093,0.653281482438187,-0.653281482438187));
#24089=DIRECTION('center_axis',(0.,0.707106781186548,0.707106781186547));
#24090=DIRECTION('ref_axis',(0.38268343236509,0.653281482438183,-0.653281482438193));
#24091=DIRECTION('',(0.,0.707106781186548,0.707106781186547));
#24092=DIRECTION('center_axis',(0.,0.707106781186548,0.707106781186547));
#24093=DIRECTION('ref_axis',(0.382683432365093,0.653281482438187,-0.653281482438187));
#24094=DIRECTION('center_axis',(0.,0.707106781186547,-0.707106781186548));
#24095=DIRECTION('ref_axis',(0.,0.707106781186548,0.707106781186547));
#24096=DIRECTION('center_axis',(0.,-0.707106781186547,0.707106781186548));
#24097=DIRECTION('ref_axis',(0.923879532511285,0.270598050073102,0.270598050073102));
#24098=DIRECTION('',(-1.,0.,0.));
#24099=DIRECTION('center_axis',(0.,-0.707106781186548,-0.707106781186547));
#24100=DIRECTION('ref_axis',(0.,0.707106781186547,-0.707106781186548));
#24101=DIRECTION('',(0.,-0.707106781186547,0.707106781186548));
#24102=DIRECTION('',(0.,0.707106781186547,-0.707106781186548));
#24103=DIRECTION('center_axis',(0.707106781186547,-0.5,-0.5));
#24104=DIRECTION('ref_axis',(-0.577350269189626,0.,-0.816496580927726));
#24105=DIRECTION('center_axis',(0.,-0.707106781186547,0.707106781186548));
#24106=DIRECTION('ref_axis',(0.38268343236509,0.653281482438193,0.653281482438183));
#24107=DIRECTION('center_axis',(0.382683432365087,-0.653281482438189,0.653281482438189));
#24108=DIRECTION('ref_axis',(0.923879532511288,0.270598050073096,-0.270598050073097));
#24109=DIRECTION('',(0.,-0.707106781186547,0.707106781186548));
#24110=DIRECTION('center_axis',(0.707106781186547,-0.500000000000001,0.500000000000001));
#24111=DIRECTION('ref_axis',(0.707106781186549,0.499999999999999,-0.499999999999999));
#24112=DIRECTION('',(0.,0.707106781186547,-0.707106781186548));
#24113=DIRECTION('center_axis',(0.,0.707106781186548,0.707106781186547));
#24114=DIRECTION('ref_axis',(0.,-0.707106781186547,0.707106781186548));
#24115=DIRECTION('',(1.,0.,0.));
#24116=DIRECTION('',(1.,0.,0.));
#24117=DIRECTION('',(0.,0.707106781186547,-0.707106781186548));
#24118=DIRECTION('center_axis',(-0.707106781186548,0.5,-0.5));
#24119=DIRECTION('ref_axis',(0.,0.707106781186548,0.707106781186548));
#24120=DIRECTION('center_axis',(-0.707106781186547,-0.5,-0.5));
#24121=DIRECTION('ref_axis',(-0.408248290463863,0.866025403784438,-0.288675134594813));
#24122=DIRECTION('center_axis',(-0.707106781186547,0.5,-0.5));
#24123=DIRECTION('ref_axis',(0.,0.707106781186548,0.707106781186548));
#24124=DIRECTION('center_axis',(0.,0.,1.));
#24125=DIRECTION('ref_axis',(1.,0.,0.));
#24126=DIRECTION('center_axis',(1.,0.,0.));
#24127=DIRECTION('ref_axis',(0.,1.,0.));
#24128=DIRECTION('center_axis',(0.,0.707106781186547,-0.707106781186548));
#24129=DIRECTION('ref_axis',(0.923879532511285,0.270598050073102,0.270598050073102));
#24130=DIRECTION('',(0.,-0.707106781186547,0.707106781186548));
#24131=DIRECTION('center_axis',(0.,0.,1.));
#24132=DIRECTION('ref_axis',(1.,0.,0.));
#24133=DIRECTION('center_axis',(0.,-0.707106781186547,0.707106781186548));
#24134=DIRECTION('ref_axis',(0.923879532511285,0.270598050073101,0.270598050073101));
#24135=DIRECTION('center_axis',(1.,0.,0.));
#24136=DIRECTION('ref_axis',(0.,1.,0.));
#24137=DIRECTION('',(-1.,0.,0.));
#24138=DIRECTION('center_axis',(-1.,0.,0.));
#24139=DIRECTION('ref_axis',(0.,1.,0.));
#24140=DIRECTION('center_axis',(0.707106781186547,0.5,0.5));
#24141=DIRECTION('ref_axis',(0.577350269189626,0.,-0.816496580927726));
#24142=DIRECTION('center_axis',(-0.707106781186547,-0.5,-0.5));
#24143=DIRECTION('ref_axis',(-0.707106781186548,0.5,0.5));
#24144=DIRECTION('center_axis',(-0.577350269189627,0.816496580927725,-2.56395024851142E-16));
#24145=DIRECTION('ref_axis',(0.816496580927726,0.577350269189626,0.));
#24146=DIRECTION('center_axis',(-0.577350269189625,0.816496580927726,-2.55393481785319E-15));
#24147=DIRECTION('ref_axis',(0.707106781186547,0.5,0.5));
#24148=DIRECTION('center_axis',(0.577350269189627,-0.816496580927725,1.25192883228098E-15));
#24149=DIRECTION('ref_axis',(0.707106781186547,0.5,-0.5));
#24150=DIRECTION('',(0.577350269189627,-0.816496580927725,2.47807419869614E-16));
#24151=DIRECTION('center_axis',(0.,0.,1.));
#24152=DIRECTION('ref_axis',(1.,0.,0.));
#24153=DIRECTION('center_axis',(1.,-1.9721522630525E-29,3.14018491736754E-15));
#24154=DIRECTION('ref_axis',(2.22044604925032E-15,0.707106781186548,-0.707106781186548));
#24155=DIRECTION('center_axis',(1.,0.,0.));
#24156=DIRECTION('ref_axis',(0.,1.,0.));
#24157=DIRECTION('center_axis',(0.,0.707106781186547,-0.707106781186548));
#24158=DIRECTION('ref_axis',(0.923879532511285,0.270598050073102,0.270598050073102));
#24159=DIRECTION('center_axis',(0.,-0.707106781186548,0.707106781186548));
#24160=DIRECTION('ref_axis',(1.,0.,0.));
#24161=DIRECTION('',(0.,-0.707106781186547,0.707106781186548));
#24162=DIRECTION('center_axis',(0.,0.,1.));
#24163=DIRECTION('ref_axis',(1.,0.,0.));
#24164=DIRECTION('center_axis',(0.707106781186547,0.500000000000001,0.500000000000001));
#24165=DIRECTION('ref_axis',(0.577350269189627,0.,-0.816496580927725));
#24166=DIRECTION('center_axis',(-1.,0.,0.));
#24167=DIRECTION('ref_axis',(0.,0.,1.));
#24168=DIRECTION('center_axis',(1.,0.,0.));
#24169=DIRECTION('ref_axis',(0.,1.,0.));
#24170=DIRECTION('center_axis',(0.,-1.,1.22464679914735E-16));
#24171=DIRECTION('ref_axis',(0.,-1.22464679914735E-16,-1.));
#24172=DIRECTION('center_axis',(-1.,0.,0.));
#24173=DIRECTION('ref_axis',(0.,1.,0.));
#24174=DIRECTION('center_axis',(1.,0.,0.));
#24175=DIRECTION('ref_axis',(0.,1.,0.));
#24176=DIRECTION('center_axis',(1.,0.,0.));
#24177=DIRECTION('ref_axis',(0.,1.,0.));
#24178=DIRECTION('',(-1.,0.,0.));
#24179=DIRECTION('center_axis',(-1.,0.,0.));
#24180=DIRECTION('ref_axis',(0.,-0.97051674265181,-0.241033715966295));
#24181=DIRECTION('',(-1.,0.,0.));
#24182=DIRECTION('center_axis',(1.,0.,0.));
#24183=DIRECTION('ref_axis',(0.,1.,0.));
#24184=DIRECTION('',(1.,0.,0.));
#24185=DIRECTION('center_axis',(-1.,0.,0.));
#24186=DIRECTION('ref_axis',(0.,0.241033715966294,-0.97051674265181));
#24187=DIRECTION('',(-1.,0.,0.));
#24188=DIRECTION('center_axis',(1.,0.,0.));
#24189=DIRECTION('ref_axis',(0.,1.,0.));
#24190=DIRECTION('',(1.,0.,0.));
#24191=DIRECTION('center_axis',(-1.,0.,0.));
#24192=DIRECTION('ref_axis',(0.,0.969995350913823,0.24312346494234));
#24193=DIRECTION('',(-1.,0.,0.));
#24194=DIRECTION('center_axis',(1.,0.,0.));
#24195=DIRECTION('ref_axis',(0.,1.,0.));
#24196=DIRECTION('',(1.,0.,0.));
#24197=DIRECTION('center_axis',(-1.,0.,0.));
#24198=DIRECTION('ref_axis',(0.,-0.241033715966295,0.97051674265181));
#24199=DIRECTION('',(-1.,0.,0.));
#24200=DIRECTION('center_axis',(1.,0.,0.));
#24201=DIRECTION('ref_axis',(0.,1.,0.));
#24202=DIRECTION('',(1.,0.,0.));
#24203=DIRECTION('center_axis',(-1.,0.,0.));
#24204=DIRECTION('ref_axis',(0.,-0.97051674265181,-0.241033715966295));
#24205=DIRECTION('center_axis',(-1.,0.,0.));
#24206=DIRECTION('ref_axis',(0.,0.,1.));
#24207=DIRECTION('center_axis',(1.,0.,0.));
#24208=DIRECTION('ref_axis',(0.,0.,-1.));
#24209=DIRECTION('center_axis',(0.,0.418358158739791,-0.908282142847613));
#24210=DIRECTION('ref_axis',(-0.707106781186555,0.642252462438189,0.295823891009622));
#24211=DIRECTION('',(0.,0.418358158739791,-0.908282142847613));
#24212=DIRECTION('center_axis',(0.,-0.418358158739791,0.908282142847613));
#24213=DIRECTION('ref_axis',(0.,0.908282142847613,0.418358158739791));
#24214=DIRECTION('',(0.,-0.418358158739791,0.908282142847613));
#24215=DIRECTION('center_axis',(1.,0.,0.));
#24216=DIRECTION('ref_axis',(0.,0.,-1.));
#24217=DIRECTION('center_axis',(0.,0.418358158739791,-0.908282142847613));
#24218=DIRECTION('ref_axis',(0.,-0.908282142847613,-0.418358158739791));
#24219=DIRECTION('center_axis',(-1.,0.,0.));
#24220=DIRECTION('ref_axis',(0.,0.418358158739791,-0.908282142847613));
#24221=DIRECTION('center_axis',(1.,0.,0.));
#24222=DIRECTION('ref_axis',(0.,0.418358158739791,-0.908282142847613));
#24223=DIRECTION('center_axis',(0.,-0.418358158739791,0.908282142847613));
#24224=DIRECTION('ref_axis',(-0.707106781186553,-0.642252462438188,-0.295823891009627));
#24225=DIRECTION('center_axis',(1.17829328657438E-14,0.418358158739788,
-0.908282142847614));
#24226=DIRECTION('ref_axis',(0.,-0.908282142847615,-0.418358158739788));
#24227=DIRECTION('',(0.,0.418358158739791,-0.908282142847613));
#24228=DIRECTION('',(0.,-0.418358158739791,0.908282142847613));
#24229=DIRECTION('center_axis',(0.,0.,1.));
#24230=DIRECTION('ref_axis',(-0.882931989457712,-0.469500907339108,0.));
#24231=DIRECTION('center_axis',(-0.362122741649372,0.389964366236962,-0.846637415335365));
#24232=DIRECTION('ref_axis',(0.,-0.908282142847613,-0.418358158739791));
#24233=DIRECTION('center_axis',(0.,-0.738355409626738,0.674411809708973));
#24234=DIRECTION('ref_axis',(0.,0.674411809708973,0.738355409626738));
#24235=DIRECTION('center_axis',(-0.115099770040445,-0.983149096918184,0.142020759628991));
#24236=DIRECTION('ref_axis',(-0.619019837529353,0.182805506560833,0.763804024286447));
#24237=DIRECTION('center_axis',(0.381760244687915,-0.386672292982237,0.839490115138756));
#24238=DIRECTION('ref_axis',(-0.70710678118655,0.462718383602925,0.534688411578082));
#24239=DIRECTION('center_axis',(-1.,0.,0.));
#24240=DIRECTION('ref_axis',(0.,-0.600825752699094,0.799380019073261));
#24241=DIRECTION('center_axis',(0.776895413605824,-9.19403442267706E-16,
0.629629666008707));
#24242=DIRECTION('ref_axis',(0.619019837529357,-0.182805506560832,-0.763804024286444));
#24243=DIRECTION('center_axis',(-1.,0.,0.));
#24244=DIRECTION('ref_axis',(0.,-0.600825752699094,0.799380019073261));
#24245=DIRECTION('center_axis',(0.,-0.756163603297457,0.654382613650612));
#24246=DIRECTION('ref_axis',(0.,0.654382613650612,0.756163603297457));
#24247=DIRECTION('center_axis',(-1.,0.,0.));
#24248=DIRECTION('ref_axis',(0.,0.,1.));
#24249=DIRECTION('center_axis',(1.,0.,0.));
#24250=DIRECTION('ref_axis',(0.,0.975243650528983,0.221133041635355));
#24251=DIRECTION('',(0.,0.908282142847613,0.41835815873979));
#24252=DIRECTION('center_axis',(-1.,0.,0.));
#24253=DIRECTION('ref_axis',(0.,-0.908282142847614,-0.418358158739789));
#24254=DIRECTION('',(0.,-0.908282142847613,-0.41835815873979));
#24255=DIRECTION('center_axis',(1.,0.,0.));
#24256=DIRECTION('ref_axis',(0.,0.19866967435672,-0.980066508197783));
#24257=DIRECTION('',(0.,0.41835815873979,-0.908282142847613));
#24258=DIRECTION('center_axis',(-1.,0.,0.));
#24259=DIRECTION('ref_axis',(0.,-0.41835815873979,0.908282142847613));
#24260=DIRECTION('',(0.,-0.41835815873979,0.908282142847613));
#24261=DIRECTION('center_axis',(1.,0.,0.));
#24262=DIRECTION('ref_axis',(0.,-0.980066508197783,-0.198669674356721));
#24263=DIRECTION('',(0.,-0.908282142847613,-0.418358158739791));
#24264=DIRECTION('center_axis',(-1.,0.,0.));
#24265=DIRECTION('ref_axis',(0.,0.908282142847613,0.418358158739791));
#24266=DIRECTION('',(0.,0.908282142847613,0.418358158739791));
#24267=DIRECTION('center_axis',(1.,0.,0.));
#24268=DIRECTION('ref_axis',(0.,-0.210810429782021,0.977526962643548));
#24269=DIRECTION('center_axis',(-1.,0.,0.));
#24270=DIRECTION('ref_axis',(0.,-1.,0.));
#24271=DIRECTION('center_axis',(1.,0.,0.));
#24272=DIRECTION('ref_axis',(0.,0.,-1.));
#24273=DIRECTION('center_axis',(-1.,0.,0.));
#24274=DIRECTION('ref_axis',(0.,0.975243650528983,0.221133041635355));
#24275=DIRECTION('center_axis',(-4.03739704015074E-15,0.416488486990263,
0.909140990278494));
#24276=DIRECTION('ref_axis',(-0.707106781186543,0.64285975928058,-0.294501833436945));
#24277=DIRECTION('center_axis',(1.,0.,0.));
#24278=DIRECTION('ref_axis',(0.,1.,0.));
#24279=DIRECTION('center_axis',(1.,0.,0.));
#24280=DIRECTION('ref_axis',(0.,0.969995350913823,0.24312346494234));
#24281=DIRECTION('center_axis',(1.,0.,0.));
#24282=DIRECTION('ref_axis',(0.,0.,-1.));
#24283=DIRECTION('center_axis',(-1.77862036335276E-15,0.404205740461642,
0.914668092467347));
#24284=DIRECTION('ref_axis',(0.,0.914668092467347,-0.404205740461642));
#24285=DIRECTION('center_axis',(1.,0.,0.));
#24286=DIRECTION('ref_axis',(0.,-0.600825752699096,0.79938001907326));
#24287=DIRECTION('',(1.,0.,0.));
#24288=DIRECTION('center_axis',(1.,0.,0.));
#24289=DIRECTION('ref_axis',(0.,-0.600825752699096,0.79938001907326));
#24290=DIRECTION('center_axis',(0.,0.908282142847613,0.418358158739791));
#24291=DIRECTION('ref_axis',(-0.707106781186555,-0.295823891009622,0.642252462438189));
#24292=DIRECTION('',(0.,0.908282142847613,0.418358158739791));
#24293=DIRECTION('center_axis',(0.,-0.908282142847613,-0.418358158739791));
#24294=DIRECTION('ref_axis',(0.,-0.418358158739791,0.908282142847613));
#24295=DIRECTION('center_axis',(1.,0.,0.));
#24296=DIRECTION('ref_axis',(0.,0.908282142847613,0.418358158739792));
#24297=DIRECTION('center_axis',(0.,0.908282142847616,0.418358158739784));
#24298=DIRECTION('ref_axis',(0.,0.418358158739784,-0.908282142847616));
#24299=DIRECTION('center_axis',(1.,0.,0.));
#24300=DIRECTION('ref_axis',(0.,0.908282142847613,0.418358158739791));
#24301=DIRECTION('center_axis',(0.,-0.908282142847613,-0.418358158739791));
#24302=DIRECTION('ref_axis',(-0.707106781186548,0.295823891009625,-0.642252462438195));
#24303=DIRECTION('',(0.,-0.908282142847613,-0.418358158739791));
#24304=DIRECTION('center_axis',(-0.707106781186546,0.642252462438197,0.295823891009625));
#24305=DIRECTION('ref_axis',(-0.707106781186549,-0.642252462438194,-0.295823891009623));
#24306=DIRECTION('center_axis',(1.,0.,0.));
#24307=DIRECTION('ref_axis',(0.,0.,-1.));
#24308=DIRECTION('center_axis',(-5.98998015374409E-15,-0.738355409626737,
0.674411809708974));
#24309=DIRECTION('ref_axis',(-1.,0.,-8.88178419700113E-15));
#24310=DIRECTION('center_axis',(-1.,0.,0.));
#24311=DIRECTION('ref_axis',(0.,-0.980066508197783,-0.198669674356721));
#24312=DIRECTION('center_axis',(1.,0.,0.));
#24313=DIRECTION('ref_axis',(0.,-0.216171072508796,0.976355502575981));
#24314=DIRECTION('center_axis',(-1.,0.,0.));
#24315=DIRECTION('ref_axis',(0.,-0.210810429782021,0.977526962643547));
#24316=DIRECTION('center_axis',(0.,-0.908282142847613,-0.418358158739791));
#24317=DIRECTION('ref_axis',(0.,0.418358158739791,-0.908282142847613));
#24318=DIRECTION('',(-1.,0.,0.));
#24319=DIRECTION('',(0.,0.418358158739791,-0.908282142847613));
#24320=DIRECTION('',(1.,0.,0.));
#24321=DIRECTION('center_axis',(1.,0.,0.));
#24322=DIRECTION('ref_axis',(0.,1.,0.));
#24323=DIRECTION('center_axis',(1.,0.,0.));
#24324=DIRECTION('ref_axis',(0.,-0.241033715966295,0.97051674265181));
#24325=DIRECTION('center_axis',(1.,0.,0.));
#24326=DIRECTION('ref_axis',(0.,-0.799380019073275,-0.600825752699076));
#24327=DIRECTION('',(1.,0.,0.));
#24328=DIRECTION('center_axis',(1.,0.,0.));
#24329=DIRECTION('ref_axis',(0.,-0.799380019073275,-0.600825752699076));
#24330=DIRECTION('center_axis',(-0.381760244555379,-0.386672293005136,0.83949011518848));
#24331=DIRECTION('ref_axis',(0.,0.908282142847615,0.418358158739788));
#24332=DIRECTION('center_axis',(0.362122741649375,0.389964366236962,-0.846637415335364));
#24333=DIRECTION('ref_axis',(-0.707106781186545,-0.476881163957516,-0.522096117072833));
#24334=DIRECTION('center_axis',(0.,0.,1.));
#24335=DIRECTION('ref_axis',(-0.882931989457715,0.469500907339103,0.));
#24336=DIRECTION('center_axis',(0.,0.41835815873979,-0.908282142847613));
#24337=DIRECTION('ref_axis',(-0.707106781186547,0.642252462438196,0.295823891009626));
#24338=DIRECTION('center_axis',(1.,0.,0.));
#24339=DIRECTION('ref_axis',(0.,0.600825752699123,-0.79938001907324));
#24340=DIRECTION('center_axis',(1.,0.,0.));
#24341=DIRECTION('ref_axis',(0.,-0.654382613650613,-0.756163603297456));
#24342=DIRECTION('center_axis',(1.,0.,0.));
#24343=DIRECTION('ref_axis',(0.,-0.654382613650613,-0.756163603297456));
#24344=DIRECTION('',(1.,0.,0.));
#24345=DIRECTION('center_axis',(1.,0.,0.));
#24346=DIRECTION('ref_axis',(0.,0.600825752699123,-0.79938001907324));
#24347=DIRECTION('center_axis',(0.115099770900997,-0.983149096632188,0.142020760911393));
#24348=DIRECTION('ref_axis',(-0.619019836769066,-0.18280550809895,-0.763804024534489));
#24349=DIRECTION('center_axis',(0.,0.756163603307808,-0.654382613638651));
#24350=DIRECTION('ref_axis',(0.,-0.654382613638651,-0.756163603307808));
#24351=DIRECTION('center_axis',(-0.776895414084112,1.7867651802561E-15,
0.62962966541855));
#24352=DIRECTION('ref_axis',(0.619019836769075,0.182805508098944,0.763804024534484));
#24353=DIRECTION('center_axis',(0.,0.418358158739791,-0.908282142847613));
#24354=DIRECTION('ref_axis',(0.,0.908282142847613,0.418358158739791));
#24355=DIRECTION('',(-1.,0.,0.));
#24356=DIRECTION('',(0.,0.908282142847613,0.418358158739791));
#24357=DIRECTION('',(1.,0.,0.));
#24358=DIRECTION('center_axis',(1.,0.,0.));
#24359=DIRECTION('ref_axis',(0.,-0.977546692794496,-0.210718920381021));
#24360=DIRECTION('center_axis',(1.,0.,0.));
#24361=DIRECTION('ref_axis',(0.,-0.97051674265181,-0.241033715966295));
#24362=DIRECTION('center_axis',(1.,0.,0.));
#24363=DIRECTION('ref_axis',(0.,0.,-1.));
#24364=DIRECTION('center_axis',(-1.,0.,0.));
#24365=DIRECTION('ref_axis',(0.,-0.712574909369129,0.701596036574878));
#24366=DIRECTION('center_axis',(0.,-0.418358158739791,0.908282142847613));
#24367=DIRECTION('ref_axis',(0.,-0.908282142847613,-0.418358158739791));
#24368=DIRECTION('',(1.,0.,0.));
#24369=DIRECTION('',(0.,-0.908282142847613,-0.418358158739791));
#24370=DIRECTION('center_axis',(1.,0.,0.));
#24371=DIRECTION('ref_axis',(0.,-0.218855045483687,0.975757382276113));
#24372=DIRECTION('center_axis',(-1.,0.,0.));
#24373=DIRECTION('ref_axis',(0.,0.701596036574878,0.712574909369129));
#24374=DIRECTION('center_axis',(0.,0.908282142847613,0.418358158739791));
#24375=DIRECTION('ref_axis',(0.,-0.418358158739791,0.908282142847613));
#24376=DIRECTION('',(1.,0.,0.));
#24377=DIRECTION('',(0.,-0.418358158739791,0.908282142847613));
#24378=DIRECTION('center_axis',(0.545880488382889,0.761016047468252,0.350526843335369));
#24379=DIRECTION('ref_axis',(0.,0.418358158739799,-0.90828214284761));
#24380=DIRECTION('center_axis',(-0.551814247024938,-0.757477375369894,-0.348896922576048));
#24381=DIRECTION('ref_axis',(-0.70710678118655,0.64676801069249,-0.285816620134091));
#24382=DIRECTION('center_axis',(0.,0.,1.));
#24383=DIRECTION('ref_axis',(1.,0.,0.));
#24384=DIRECTION('center_axis',(0.,0.908282142847613,0.41835815873979));
#24385=DIRECTION('ref_axis',(-0.707106781186551,0.295823891009619,-0.642252462438195));
#24386=DIRECTION('center_axis',(0.,0.,1.));
#24387=DIRECTION('ref_axis',(1.,0.,0.));
#24388=DIRECTION('center_axis',(-1.,0.,0.));
#24389=DIRECTION('ref_axis',(0.,0.712574909369127,-0.70159603657488));
#24390=DIRECTION('center_axis',(0.,-0.908282142847613,-0.41835815873979));
#24391=DIRECTION('ref_axis',(-0.707106781186552,0.295823891009633,-0.642252462438187));
#24392=DIRECTION('',(0.,-0.908282142847613,-0.41835815873979));
#24393=DIRECTION('center_axis',(0.,0.908282142847613,0.418358158739791));
#24394=DIRECTION('ref_axis',(0.,0.418358158739791,-0.908282142847613));
#24395=DIRECTION('center_axis',(0.,-0.41835815873979,0.908282142847613));
#24396=DIRECTION('ref_axis',(0.,-0.908282142847613,-0.41835815873979));
#24397=DIRECTION('',(-1.,0.,0.));
#24398=DIRECTION('',(0.,-0.908282142847613,-0.41835815873979));
#24399=DIRECTION('',(1.,0.,0.));
#24400=DIRECTION('center_axis',(-1.,0.,0.));
#24401=DIRECTION('ref_axis',(0.,0.712574909369129,-0.701596036574878));
#24402=DIRECTION('center_axis',(-1.,0.,0.));
#24403=DIRECTION('ref_axis',(0.,-0.701596036574868,-0.712574909369139));
#24404=DIRECTION('center_axis',(1.,0.,0.));
#24405=DIRECTION('ref_axis',(0.,-0.908282142847615,-0.418358158739787));
#24406=DIRECTION('',(-1.,0.,0.));
#24407=DIRECTION('center_axis',(0.545880488382904,0.35052684333534,-0.761016047468255));
#24408=DIRECTION('ref_axis',(-3.55271367880051E-14,-0.908282142847614,-0.41835815873979));
#24409=DIRECTION('center_axis',(-0.551814249371486,-0.348896917908686,0.757477375810264));
#24410=DIRECTION('ref_axis',(-0.70710678118654,-0.285816620074966,-0.646768010718629));
#24411=DIRECTION('center_axis',(0.,0.,1.));
#24412=DIRECTION('ref_axis',(1.,0.,0.));
#24413=DIRECTION('center_axis',(0.,0.41835815873979,-0.908282142847613));
#24414=DIRECTION('ref_axis',(-0.707106781186553,-0.642252462438192,-0.295823891009619));
#24415=DIRECTION('center_axis',(0.,-0.909140990278493,0.416488486990267));
#24416=DIRECTION('ref_axis',(0.,-0.416488486990267,-0.909140990278493));
#24417=DIRECTION('center_axis',(0.,0.,1.));
#24418=DIRECTION('ref_axis',(1.,0.,0.));
#24419=DIRECTION('center_axis',(0.,-0.914668092467346,0.404205740461645));
#24420=DIRECTION('ref_axis',(0.,-0.404205740461645,-0.914668092467346));
#24421=DIRECTION('center_axis',(1.,0.,0.));
#24422=DIRECTION('ref_axis',(0.,0.,-1.));
#24423=DIRECTION('center_axis',(1.,0.,0.));
#24424=DIRECTION('ref_axis',(0.,0.241033715966294,-0.97051674265181));
#24425=DIRECTION('center_axis',(7.50087139441506E-14,0.654382613650666,
0.75616360329741));
#24426=DIRECTION('ref_axis',(-0.707106781186547,0.534688411578089,-0.462718383602923));
#24427=DIRECTION('center_axis',(1.,0.,0.));
#24428=DIRECTION('ref_axis',(0.,1.,0.));
#24429=DIRECTION('center_axis',(-1.,0.,0.));
#24430=DIRECTION('ref_axis',(0.,0.19866967435672,-0.980066508197783));
#24431=DIRECTION('center_axis',(1.,0.,0.));
#24432=DIRECTION('ref_axis',(0.,0.,-1.));
#24433=DIRECTION('center_axis',(1.,0.,0.));
#24434=DIRECTION('ref_axis',(0.,-0.515822394929815,-0.856695545038533));
#24435=DIRECTION('center_axis',(1.,0.,0.));
#24436=DIRECTION('ref_axis',(0.,0.,-1.));
#24437=DIRECTION('',(0.,0.41835815873979,-0.908282142847613));
#24438=DIRECTION('center_axis',(1.,0.,0.));
#24439=DIRECTION('ref_axis',(0.,0.,-1.));
#24440=DIRECTION('',(0.,-0.41835815873979,0.908282142847613));
#24441=DIRECTION('center_axis',(-1.,0.,0.));
#24442=DIRECTION('ref_axis',(0.,0.,-1.));
#24443=DIRECTION('center_axis',(-0.785375350227634,-0.602017675855261,0.144084271218794));
#24444=DIRECTION('ref_axis',(-0.619019837529315,0.763804024286477,-0.182805506560837));
#24445=DIRECTION('center_axis',(0.381760244688023,0.839490115138715,0.386672292982221));
#24446=DIRECTION('ref_axis',(0.,-0.418358158739795,0.908282142847611));
#24447=DIRECTION('center_axis',(-1.,0.,0.));
#24448=DIRECTION('ref_axis',(0.,0.75616360329746,-0.654382613650609));
#24449=DIRECTION('center_axis',(0.36212274164936,0.846637415335364,0.389964366236975));
#24450=DIRECTION('ref_axis',(-0.707106781186551,0.522096117072829,-0.476881163957511));
#24451=DIRECTION('center_axis',(1.,0.,0.));
#24452=DIRECTION('ref_axis',(0.,0.79938001907329,0.600825752699055));
#24453=DIRECTION('',(1.,0.,0.));
#24454=DIRECTION('center_axis',(1.,0.,0.));
#24455=DIRECTION('ref_axis',(0.,0.79938001907329,0.600825752699055));
#24456=DIRECTION('center_axis',(1.,0.,0.));
#24457=DIRECTION('ref_axis',(0.,0.,-1.));
#24458=DIRECTION('center_axis',(0.,-0.674411809708971,-0.73835540962674));
#24459=DIRECTION('ref_axis',(-1.,0.,0.));
#24460=DIRECTION('center_axis',(0.,-0.41835815873979,0.908282142847613));
#24461=DIRECTION('ref_axis',(-0.707106781186555,-0.642252462438189,-0.295823891009622));
#24462=DIRECTION('',(0.,-0.41835815873979,0.908282142847613));
#24463=DIRECTION('center_axis',(0.,0.418358158739791,-0.908282142847613));
#24464=DIRECTION('ref_axis',(0.,-0.908282142847613,-0.418358158739791));
#24465=DIRECTION('center_axis',(1.,0.,0.));
#24466=DIRECTION('ref_axis',(0.,-0.418358158739791,0.908282142847613));
#24467=DIRECTION('center_axis',(0.,-0.418358158739791,0.908282142847613));
#24468=DIRECTION('ref_axis',(0.,0.908282142847613,0.418358158739791));
#24469=DIRECTION('center_axis',(1.,0.,0.));
#24470=DIRECTION('ref_axis',(0.,-0.418358158739791,0.908282142847613));
#24471=DIRECTION('center_axis',(0.,0.41835815873979,-0.908282142847613));
#24472=DIRECTION('ref_axis',(-0.707106781186546,0.642252462438194,0.295823891009631));
#24473=DIRECTION('',(0.,0.41835815873979,-0.908282142847613));
#24474=DIRECTION('center_axis',(0.,0.,1.));
#24475=DIRECTION('ref_axis',(-0.892745142068122,-0.450561994972688,0.));
#24476=DIRECTION('center_axis',(0.,0.908282142847613,0.41835815873979));
#24477=DIRECTION('ref_axis',(-0.707106781186553,-0.295823891009619,0.642252462438192));
#24478=DIRECTION('center_axis',(0.,0.908282142847613,0.41835815873979));
#24479=DIRECTION('ref_axis',(0.,-0.41835815873979,0.908282142847613));
#24480=DIRECTION('',(1.,0.,0.));
#24481=DIRECTION('center_axis',(0.,0.41835815873979,-0.908282142847613));
#24482=DIRECTION('ref_axis',(0.,0.908282142847613,0.41835815873979));
#24483=DIRECTION('',(0.,0.908282142847613,0.41835815873979));
#24484=DIRECTION('',(1.,0.,0.));
#24485=DIRECTION('',(0.,0.908282142847613,0.41835815873979));
#24486=DIRECTION('center_axis',(0.,0.908282142847613,0.41835815873979));
#24487=DIRECTION('ref_axis',(-0.707106781186552,-0.295823891009608,0.642252462438199));
#24488=DIRECTION('center_axis',(0.,-0.908282142847614,-0.418358158739788));
#24489=DIRECTION('ref_axis',(0.,-0.418358158739788,0.908282142847615));
#24490=DIRECTION('center_axis',(1.,0.,0.));
#24491=DIRECTION('ref_axis',(0.,0.,-1.));
#24492=DIRECTION('center_axis',(1.,0.,0.));
#24493=DIRECTION('ref_axis',(0.,-0.908282142847614,-0.418358158739789));
#24494=DIRECTION('center_axis',(1.,0.,0.));
#24495=DIRECTION('ref_axis',(0.,0.,-1.));
#24496=DIRECTION('center_axis',(1.,0.,0.));
#24497=DIRECTION('ref_axis',(0.,0.,-1.));
#24498=DIRECTION('center_axis',(1.,0.,0.));
#24499=DIRECTION('ref_axis',(0.,0.,-1.));
#24500=DIRECTION('center_axis',(0.,-1.,0.));
#24501=DIRECTION('ref_axis',(0.,0.,1.));
#24502=DIRECTION('center_axis',(1.,0.,0.));
#24503=DIRECTION('ref_axis',(0.,0.,-1.));
#24504=DIRECTION('center_axis',(1.,0.,0.));
#24505=DIRECTION('ref_axis',(0.,0.,-1.));
#24506=DIRECTION('',(1.,0.,0.));
#24507=DIRECTION('center_axis',(-1.,0.,0.));
#24508=DIRECTION('ref_axis',(0.,0.,-1.));
#24509=DIRECTION('center_axis',(-1.,0.,0.));
#24510=DIRECTION('ref_axis',(0.,0.,-1.));
#24511=DIRECTION('center_axis',(-7.105427357601E-15,-1.,1.4210854715202E-14));
#24512=DIRECTION('ref_axis',(0.577350269189629,-7.10542735760104E-15,-0.816496580927724));
#24513=DIRECTION('center_axis',(0.,-0.707106781186552,-0.707106781186543));
#24514=DIRECTION('ref_axis',(0.,0.707106781186543,-0.707106781186552));
#24515=DIRECTION('center_axis',(0.,0.707106781186548,-0.707106781186547));
#24516=DIRECTION('ref_axis',(0.707106781186548,-0.5,-0.5));
#24517=DIRECTION('center_axis',(1.,0.,0.));
#24518=DIRECTION('ref_axis',(0.,0.,-1.));
#24519=DIRECTION('center_axis',(0.,0.707106781186547,0.707106781186548));
#24520=DIRECTION('ref_axis',(0.707106781186547,0.5,-0.5));
#24521=DIRECTION('center_axis',(0.707106781186545,0.500000000000002,0.500000000000002));
#24522=DIRECTION('ref_axis',(0.70710678118655,-0.499999999999998,-0.499999999999999));
#24523=DIRECTION('',(0.,-0.707106781186547,-0.707106781186548));
#24524=DIRECTION('',(0.,0.707106781186547,0.707106781186548));
#24525=DIRECTION('center_axis',(0.,0.707106781186548,-0.707106781186547));
#24526=DIRECTION('ref_axis',(0.,0.707106781186547,0.707106781186548));
#24527=DIRECTION('',(1.,0.,0.));
#24528=DIRECTION('',(1.,0.,0.));
#24529=DIRECTION('',(0.,-0.707106781186547,-0.707106781186548));
#24530=DIRECTION('',(-1.,0.,0.));
#24531=DIRECTION('',(-1.57009245868378E-16,0.707106781186547,0.707106781186548));
#24532=DIRECTION('center_axis',(1.,0.,0.));
#24533=DIRECTION('ref_axis',(0.,0.,-1.));
#24534=DIRECTION('',(-1.,0.,0.));
#24535=DIRECTION('center_axis',(-1.,0.,0.));
#24536=DIRECTION('ref_axis',(0.,0.,-1.));
#24537=DIRECTION('center_axis',(0.,-0.707106781186547,-0.707106781186548));
#24538=DIRECTION('ref_axis',(0.923879532511287,0.270598050073103,-0.270598050073094));
#24539=DIRECTION('center_axis',(0.32505758367186,0.398112608509073,0.857813451890045));
#24540=DIRECTION('ref_axis',(0.627963030199558,-0.769094500660421,0.118979333316701));
#24541=DIRECTION('',(-3.92523114670943E-17,0.707106781186547,0.707106781186548));
#24542=DIRECTION('center_axis',(0.325057583671865,-0.857813451890045,-0.398112608509066));
#24543=DIRECTION('ref_axis',(0.627963030199555,-0.118979333316694,0.769094500660424));
#24544=DIRECTION('center_axis',(0.,0.,-1.));
#24545=DIRECTION('ref_axis',(-1.47196168001604E-16,1.,0.));
#24546=DIRECTION('',(0.,-0.707106781186547,-0.707106781186548));
#24547=DIRECTION('center_axis',(0.,1.,6.28036983473511E-15));
#24548=DIRECTION('ref_axis',(-1.47196168001605E-16,6.35971014366111E-15,
-1.));
#24549=DIRECTION('center_axis',(-0.577350269189628,0.816496580927725,-1.02558009940457E-15));
#24550=DIRECTION('ref_axis',(0.707106781186546,0.500000000000001,0.500000000000001));
#24551=DIRECTION('',(-0.577350269189628,0.816496580927725,-1.02558009940457E-15));
#24552=DIRECTION('center_axis',(-0.577350269189625,0.816496580927727,3.85594080342543E-15));
#24553=DIRECTION('ref_axis',(0.707106781186545,0.500000000000004,0.499999999999999));
#24554=DIRECTION('',(0.577350269189628,-0.816496580927725,1.02558009940457E-15));
#24555=DIRECTION('center_axis',(-0.325057583671864,0.857813451890046,-0.398112608509065));
#24556=DIRECTION('ref_axis',(0.627963030199557,-0.118979333316692,-0.769094500660423));
#24557=DIRECTION('center_axis',(0.707106781186546,0.500000000000001,-0.500000000000001));
#24558=DIRECTION('ref_axis',(-0.577350269189627,0.,-0.816496580927725));
#24559=DIRECTION('',(0.577350269189624,5.25609800944841E-15,0.816496580927727));
#24560=DIRECTION('',(1.57009245868378E-16,-0.707106781186547,-0.707106781186548));
#24561=DIRECTION('center_axis',(-0.577350269189624,-5.25609800944841E-15,
-0.816496580927727));
#24562=DIRECTION('ref_axis',(0.707106781186548,0.5,-0.5));
#24563=DIRECTION('center_axis',(-0.325057583671868,0.398112608509056,-0.857813451890049));
#24564=DIRECTION('ref_axis',(0.627963030199554,0.769094500660427,0.118979333316684));
#24565=DIRECTION('',(-0.577350269189624,-5.25609800944841E-15,-0.816496580927727));
#24566=DIRECTION('center_axis',(-0.577350269189631,9.81512204508276E-15,
-0.816496580927722));
#24567=DIRECTION('ref_axis',(0.707106781186547,0.5,-0.5));
#24568=DIRECTION('center_axis',(-1.57009245868378E-16,0.707106781186547,
0.707106781186548));
#24569=DIRECTION('ref_axis',(0.382683432365086,0.65328148243819,-0.65328148243819));
#24570=DIRECTION('center_axis',(0.,0.707106781186548,0.707106781186548));
#24571=DIRECTION('ref_axis',(0.707106781186546,0.500000000000001,-0.500000000000001));
#24572=DIRECTION('center_axis',(0.,-0.707106781186548,-0.707106781186548));
#24573=DIRECTION('ref_axis',(-2.22044604925032E-15,0.707106781186548,-0.707106781186548));
#24574=DIRECTION('center_axis',(0.707106781186545,0.500000000000001,0.500000000000002));
#24575=DIRECTION('ref_axis',(0.577350269189628,0.,-0.816496580927724));
#24576=DIRECTION('',(7.8504622934189E-17,0.707106781186548,-0.707106781186547));
#24577=DIRECTION('',(-0.577350269189628,-1.18153318744577E-15,0.816496580927725));
#24578=DIRECTION('',(-3.92523114670943E-17,-0.707106781186548,0.707106781186547));
#24579=DIRECTION('center_axis',(0.707106781186551,-0.499999999999998,-0.499999999999997));
#24580=DIRECTION('ref_axis',(-0.577350269189622,0.,-0.816496580927729));
#24581=DIRECTION('',(-3.92523114670946E-17,0.707106781186547,-0.707106781186548));
#24582=DIRECTION('center_axis',(-0.707106781186551,0.499999999999998,0.499999999999997));
#24583=DIRECTION('ref_axis',(-0.40824829046386,-0.86602540378444,0.288675134594813));
#24584=DIRECTION('',(7.85046229341884E-17,-0.707106781186547,0.707106781186548));
#24585=DIRECTION('center_axis',(0.,-0.707106781186547,0.707106781186548));
#24586=DIRECTION('ref_axis',(0.92387953251129,-0.270598050073093,-0.270598050073093));
#24587=DIRECTION('',(0.,-0.707106781186547,0.707106781186548));
#24588=DIRECTION('center_axis',(0.,-6.28036983473511E-15,-1.));
#24589=DIRECTION('ref_axis',(-4.90653893338677E-17,-1.,6.35971014366104E-15));
#24590=DIRECTION('center_axis',(1.,0.,0.));
#24591=DIRECTION('ref_axis',(0.,0.,-1.));
#24592=DIRECTION('center_axis',(1.,0.,0.));
#24593=DIRECTION('ref_axis',(0.,0.515822394929815,0.856695545038534));
#24594=DIRECTION('center_axis',(1.,0.,0.));
#24595=DIRECTION('ref_axis',(0.,0.,-1.));
#24596=DIRECTION('center_axis',(1.,0.,0.));
#24597=DIRECTION('ref_axis',(0.,0.,-1.));
#24598=DIRECTION('center_axis',(-1.,0.,0.));
#24599=DIRECTION('ref_axis',(0.,0.,-1.));
#24600=DIRECTION('center_axis',(1.,0.,0.));
#24601=DIRECTION('ref_axis',(0.,0.,-1.));
#24602=DIRECTION('center_axis',(0.,-1.,0.));
#24603=DIRECTION('ref_axis',(0.,0.,1.));
#24604=DIRECTION('center_axis',(1.,0.,0.));
#24605=DIRECTION('ref_axis',(0.,0.,-1.));
#24606=DIRECTION('center_axis',(1.,0.,0.));
#24607=DIRECTION('ref_axis',(0.,0.,-1.));
#24608=DIRECTION('',(1.,0.,0.));
#24609=DIRECTION('center_axis',(-1.,0.,0.));
#24610=DIRECTION('ref_axis',(0.,0.,-1.));
#24611=DIRECTION('center_axis',(-1.,0.,0.));
#24612=DIRECTION('ref_axis',(0.,0.,-1.));
#24613=DIRECTION('center_axis',(1.,0.,0.));
#24614=DIRECTION('ref_axis',(0.,1.,0.));
#24615=DIRECTION('center_axis',(-1.,0.,0.));
#24616=DIRECTION('ref_axis',(0.,0.707106781186545,0.70710678118655));
#24617=DIRECTION('center_axis',(-1.,0.,0.));
#24618=DIRECTION('ref_axis',(0.,1.,0.));
#24619=DIRECTION('',(1.,0.,0.));
#24620=DIRECTION('center_axis',(0.,0.,1.));
#24621=DIRECTION('ref_axis',(1.,0.,0.));
#24622=DIRECTION('center_axis',(7.8504622934189E-17,0.707106781186548,-0.707106781186547));
#24623=DIRECTION('ref_axis',(0.382683432365092,0.653281482438186,0.65328148243819));
#24624=DIRECTION('center_axis',(1.,0.,0.));
#24625=DIRECTION('ref_axis',(0.,0.,-1.));
#24626=DIRECTION('center_axis',(-1.,0.,0.));
#24627=DIRECTION('ref_axis',(0.,0.707106781186552,-0.707106781186543));
#24628=DIRECTION('',(-1.,0.,0.));
#24629=DIRECTION('center_axis',(-0.082463514308756,-0.971269669085137,0.223237538785703));
#24630=DIRECTION('ref_axis',(0.336556770590781,-0.237981574738988,-0.911095115920536));
#24631=DIRECTION('center_axis',(-7.85046229341884E-17,0.707106781186547,
-0.707106781186548));
#24632=DIRECTION('ref_axis',(0.382683432365094,-0.653281482438187,-0.653281482438187));
#24633=DIRECTION('center_axis',(-7.8504622934189E-17,-0.707106781186548,
0.707106781186547));
#24634=DIRECTION('ref_axis',(0.382683432365091,0.65328148243819,0.653281482438185));
#24635=DIRECTION('',(-7.8504622934189E-17,-0.707106781186548,0.707106781186547));
#24636=DIRECTION('center_axis',(-1.77862036335272E-14,0.707106781186548,
-0.707106781186548));
#24637=DIRECTION('ref_axis',(2.22044604925032E-15,0.707106781186548,0.707106781186548));
#24638=DIRECTION('center_axis',(-3.5527136788005E-15,-1.,-7.105427357601E-15));
#24639=DIRECTION('ref_axis',(0.50544946512442,-7.10542735760098E-15,0.862856209461019));
#24640=DIRECTION('center_axis',(0.,-0.707106781186548,-0.707106781186547));
#24641=DIRECTION('ref_axis',(0.382683432365087,-0.653281482438187,0.653281482438191));
#24642=DIRECTION('center_axis',(-0.577350269189628,-1.15377761183014E-15,
0.816496580927725));
#24643=DIRECTION('ref_axis',(0.816496580927725,0.,0.577350269189628));
#24644=DIRECTION('center_axis',(1.,0.,0.));
#24645=DIRECTION('ref_axis',(0.,0.,1.));
#24646=DIRECTION('center_axis',(1.,0.,0.));
#24647=DIRECTION('ref_axis',(0.,0.,1.));
#24648=DIRECTION('',(-1.,0.,0.));
#24649=DIRECTION('center_axis',(-1.,0.,0.));
#24650=DIRECTION('ref_axis',(0.,0.,1.));
#24651=DIRECTION('',(1.,0.,0.));
#24652=DIRECTION('center_axis',(0.,0.707106781186547,0.707106781186548));
#24653=DIRECTION('ref_axis',(0.,-0.707106781186548,0.707106781186547));
#24654=DIRECTION('',(0.,0.707106781186548,-0.707106781186547));
#24655=DIRECTION('center_axis',(0.,0.707106781186548,-0.707106781186547));
#24656=DIRECTION('ref_axis',(0.923879532511287,0.270598050073103,0.270598050073094));
#24657=DIRECTION('center_axis',(0.,0.707106781186548,-0.707106781186548));
#24658=DIRECTION('ref_axis',(0.707106781186546,0.500000000000001,0.500000000000001));
#24659=DIRECTION('',(0.,0.707106781186548,-0.707106781186547));
#24660=DIRECTION('center_axis',(-0.577350269189628,-1.15377761183014E-15,
0.816496580927725));
#24661=DIRECTION('ref_axis',(0.816496580927726,0.,0.577350269189625));
#24662=DIRECTION('',(0.577350269189628,1.12602203621451E-15,-0.816496580927725));
#24663=DIRECTION('center_axis',(-0.577350269189629,4.70725240937645E-15,
0.816496580927724));
#24664=DIRECTION('ref_axis',(0.707106781186546,-0.499999999999997,0.500000000000005));
#24665=DIRECTION('center_axis',(0.,0.,1.));
#24666=DIRECTION('ref_axis',(1.,0.,0.));
#24667=DIRECTION('center_axis',(0.,0.707106781186548,0.707106781186547));
#24668=DIRECTION('ref_axis',(0.923879532511286,-0.270598050073101,0.270598050073101));
#24669=DIRECTION('center_axis',(1.,0.,0.));
#24670=DIRECTION('ref_axis',(0.,0.,-1.));
#24671=DIRECTION('',(0.,0.707106781186548,0.707106781186547));
#24672=DIRECTION('center_axis',(0.,0.707106781186548,0.707106781186547));
#24673=DIRECTION('ref_axis',(0.923879532511286,-0.270598050073102,0.270598050073097));
#24674=DIRECTION('',(0.,-0.707106781186548,-0.707106781186547));
#24675=DIRECTION('center_axis',(0.499999999999999,0.853553390593275,0.146446609406727));
#24676=DIRECTION('ref_axis',(0.5,-0.146446609406725,-0.853553390593274));
#24677=DIRECTION('center_axis',(0.707106781186547,-0.500000000000001,0.500000000000001));
#24678=DIRECTION('ref_axis',(0.577350269189627,0.,-0.816496580927725));
#24679=DIRECTION('',(0.,0.707106781186548,0.707106781186547));
#24680=DIRECTION('',(-0.707106781186549,-0.499999999999999,0.5));
#24681=DIRECTION('center_axis',(1.,0.,0.));
#24682=DIRECTION('ref_axis',(0.,0.,-1.));
#24683=DIRECTION('center_axis',(-1.,0.,0.));
#24684=DIRECTION('ref_axis',(0.,1.,0.));
#24685=DIRECTION('center_axis',(0.,-1.,-1.22464679914735E-16));
#24686=DIRECTION('ref_axis',(0.,-1.22464679914735E-16,1.));
#24687=DIRECTION('center_axis',(1.,0.,0.));
#24688=DIRECTION('ref_axis',(0.,1.,0.));
#24689=DIRECTION('center_axis',(-1.,0.,0.));
#24690=DIRECTION('ref_axis',(0.,1.,0.));
#24691=DIRECTION('center_axis',(1.,0.,0.));
#24692=DIRECTION('ref_axis',(0.,1.,0.));
#24693=DIRECTION('center_axis',(1.,0.,0.));
#24694=DIRECTION('ref_axis',(0.,-1.,1.83697019872103E-16));
#24695=DIRECTION('',(-1.,0.,0.));
#24696=DIRECTION('center_axis',(1.,0.,0.));
#24697=DIRECTION('ref_axis',(0.,-1.,1.83697019872103E-16));
#24698=DIRECTION('center_axis',(1.,0.,0.));
#24699=DIRECTION('ref_axis',(0.,0.,-1.));
#24700=DIRECTION('center_axis',(1.,0.,0.));
#24701=DIRECTION('ref_axis',(0.,0.,-1.));
#24702=DIRECTION('center_axis',(1.,0.,0.));
#24703=DIRECTION('ref_axis',(0.,0.,-1.));
#24704=DIRECTION('center_axis',(-1.,0.,0.));
#24705=DIRECTION('ref_axis',(0.,-1.,3.06161699786838E-17));
#24706=DIRECTION('center_axis',(-1.,0.,0.));
#24707=DIRECTION('ref_axis',(0.,-1.,3.06161699786838E-17));
#24708=DIRECTION('center_axis',(0.,-1.,-1.22464679914735E-16));
#24709=DIRECTION('ref_axis',(0.,-1.22464679914735E-16,1.));
#24710=DIRECTION('center_axis',(-1.,0.,0.));
#24711=DIRECTION('ref_axis',(0.,1.,0.));
#24712=DIRECTION('center_axis',(1.,0.,0.));
#24713=DIRECTION('ref_axis',(0.,-1.,3.06161699786838E-17));
#24714=DIRECTION('',(-0.707106781186544,-0.707106781186551,-8.65956056235498E-17));
#24715=DIRECTION('center_axis',(1.,0.,0.));
#24716=DIRECTION('ref_axis',(0.,-1.,3.06161699786838E-17));
#24717=DIRECTION('center_axis',(1.,0.,0.));
#24718=DIRECTION('ref_axis',(0.,0.,-1.));
#24719=DIRECTION('center_axis',(1.,0.,0.));
#24720=DIRECTION('ref_axis',(0.,-0.856695545038534,0.515822394929815));
#24721=DIRECTION('center_axis',(1.,0.,0.));
#24722=DIRECTION('ref_axis',(0.,0.,-1.));
#24723=DIRECTION('center_axis',(1.,0.,0.));
#24724=DIRECTION('ref_axis',(0.,0.,-1.));
#24725=DIRECTION('center_axis',(-1.,0.,0.));
#24726=DIRECTION('ref_axis',(0.,0.,-1.));
#24727=DIRECTION('center_axis',(1.,0.,0.));
#24728=DIRECTION('ref_axis',(0.,0.,-1.));
#24729=DIRECTION('center_axis',(1.,0.,0.));
#24730=DIRECTION('ref_axis',(0.,0.856695545038533,-0.515822394929815));
#24731=DIRECTION('center_axis',(1.,0.,0.));
#24732=DIRECTION('ref_axis',(0.,0.,-1.));
#24733=DIRECTION('center_axis',(-1.,0.,0.));
#24734=DIRECTION('ref_axis',(0.,0.,-1.));
#24735=DIRECTION('center_axis',(-0.707106781186549,-0.499999999999999,0.5));
#24736=DIRECTION('ref_axis',(0.,-0.70710678118655,-0.707106781186545));
#24737=DIRECTION('center_axis',(-0.707106781186548,-0.5,0.5));
#24738=DIRECTION('ref_axis',(0.,-0.707106781186548,-0.707106781186548));
#24739=DIRECTION('center_axis',(0.382683432365078,0.653281482438192,-0.653281482438192));
#24740=DIRECTION('ref_axis',(0.923879532511292,-0.270598050073089,0.270598050073091));
#24741=DIRECTION('center_axis',(-7.85046229341884E-17,0.707106781186547,
-0.707106781186548));
#24742=DIRECTION('ref_axis',(0.382683432365097,-0.653281482438186,-0.653281482438186));
#24743=DIRECTION('',(-7.85046229341884E-17,0.707106781186547,-0.707106781186548));
#24744=DIRECTION('center_axis',(0.,-0.707106781186548,-0.707106781186547));
#24745=DIRECTION('ref_axis',(0.,0.707106781186547,-0.707106781186548));
#24746=DIRECTION('',(1.,0.,0.));
#24747=DIRECTION('',(0.,0.707106781186547,-0.707106781186548));
#24748=DIRECTION('center_axis',(0.,-0.707106781186548,-0.707106781186547));
#24749=DIRECTION('ref_axis',(0.382683432365089,-0.653281482438186,0.653281482438191));
#24750=DIRECTION('',(0.,-0.707106781186548,-0.707106781186547));
#24751=DIRECTION('center_axis',(0.,0.707106781186548,0.707106781186548));
#24752=DIRECTION('ref_axis',(0.,-0.707106781186548,0.707106781186548));
#24753=DIRECTION('center_axis',(0.,0.,1.));
#24754=DIRECTION('ref_axis',(1.,0.,0.));
#24755=DIRECTION('center_axis',(1.,0.,0.));
#24756=DIRECTION('ref_axis',(0.,-1.,0.));
#24757=DIRECTION('center_axis',(0.,-0.707106781186547,0.707106781186548));
#24758=DIRECTION('ref_axis',(0.,-0.707106781186548,-0.707106781186547));
#24759=DIRECTION('',(0.,0.707106781186548,0.707106781186547));
#24760=DIRECTION('',(-1.,0.,0.));
#24761=DIRECTION('',(0.,-0.707106781186548,-0.707106781186547));
#24762=DIRECTION('',(-1.,0.,0.));
#24763=DIRECTION('center_axis',(1.,0.,0.));
#24764=DIRECTION('ref_axis',(0.,-1.,0.));
#24765=DIRECTION('center_axis',(-0.707106781186547,-0.500000000000001,-0.500000000000001));
#24766=DIRECTION('ref_axis',(0.707106781186549,-0.499999999999999,-0.499999999999999));
#24767=DIRECTION('center_axis',(1.,0.,0.));
#24768=DIRECTION('ref_axis',(0.,0.,-1.));
#24769=DIRECTION('center_axis',(0.,-1.,0.));
#24770=DIRECTION('ref_axis',(0.,0.,1.));
#24771=DIRECTION('center_axis',(1.,0.,0.));
#24772=DIRECTION('ref_axis',(0.,0.,-1.));
#24773=DIRECTION('center_axis',(1.,0.,0.));
#24774=DIRECTION('ref_axis',(0.,0.,-1.));
#24775=DIRECTION('',(1.,0.,0.));
#24776=DIRECTION('center_axis',(-1.,0.,0.));
#24777=DIRECTION('ref_axis',(0.,0.,-1.));
#24778=DIRECTION('center_axis',(-1.,0.,0.));
#24779=DIRECTION('ref_axis',(0.,0.,-1.));
#24780=DIRECTION('center_axis',(1.,0.,0.));
#24781=DIRECTION('ref_axis',(0.,0.,-1.));
#24782=DIRECTION('center_axis',(0.,-1.,0.));
#24783=DIRECTION('ref_axis',(0.,0.,1.));
#24784=DIRECTION('center_axis',(1.,0.,0.));
#24785=DIRECTION('ref_axis',(0.,0.,-1.));
#24786=DIRECTION('center_axis',(1.,0.,0.));
#24787=DIRECTION('ref_axis',(0.,0.,-1.));
#24788=DIRECTION('',(1.,0.,0.));
#24789=DIRECTION('center_axis',(-1.,0.,0.));
#24790=DIRECTION('ref_axis',(0.,0.,-1.));
#24791=DIRECTION('center_axis',(-1.,0.,0.));
#24792=DIRECTION('ref_axis',(0.,0.,-1.));
#24793=DIRECTION('center_axis',(-1.,0.,0.));
#24794=DIRECTION('ref_axis',(0.,0.,1.));
#24795=DIRECTION('center_axis',(1.,0.,0.));
#24796=DIRECTION('ref_axis',(0.,0.,-1.));
#24797=DIRECTION('center_axis',(0.,-1.,0.));
#24798=DIRECTION('ref_axis',(0.,0.,-1.));
#24799=DIRECTION('center_axis',(-1.,0.,0.));
#24800=DIRECTION('ref_axis',(0.,0.,-1.));
#24801=DIRECTION('center_axis',(-1.,0.,0.));
#24802=DIRECTION('ref_axis',(0.,0.,-1.));
#24803=DIRECTION('center_axis',(1.,0.,0.));
#24804=DIRECTION('ref_axis',(0.,0.,-1.));
#24805=DIRECTION('center_axis',(-1.,0.,0.));
#24806=DIRECTION('ref_axis',(0.,-1.,1.83697019872103E-16));
#24807=DIRECTION('center_axis',(1.,0.,0.));
#24808=DIRECTION('ref_axis',(0.,0.,-1.));
#24809=DIRECTION('center_axis',(1.,0.,0.));
#24810=DIRECTION('ref_axis',(0.,0.,-1.));
#24811=DIRECTION('center_axis',(1.,0.,0.));
#24812=DIRECTION('ref_axis',(0.,0.,-1.));
#24813=DIRECTION('center_axis',(1.,0.,0.));
#24814=DIRECTION('ref_axis',(0.,0.,-1.));
#24815=DIRECTION('center_axis',(-1.,0.,0.));
#24816=DIRECTION('ref_axis',(0.,0.,-1.));
#24817=DIRECTION('center_axis',(-1.,0.,0.));
#24818=DIRECTION('ref_axis',(0.,0.,-1.));
#24819=DIRECTION('center_axis',(-1.,0.,0.));
#24820=DIRECTION('ref_axis',(0.,0.,-1.));
#24821=DIRECTION('center_axis',(1.,0.,0.));
#24822=DIRECTION('ref_axis',(0.,-1.,1.83697019872103E-16));
#24823=DIRECTION('center_axis',(1.,0.,0.));
#24824=DIRECTION('ref_axis',(0.,0.,-1.));
#24825=DIRECTION('center_axis',(1.,0.,0.));
#24826=DIRECTION('ref_axis',(0.,0.,-1.));
#24827=DIRECTION('center_axis',(1.,0.,0.));
#24828=DIRECTION('ref_axis',(0.,0.,-1.));
#24829=DIRECTION('center_axis',(1.,0.,0.));
#24830=DIRECTION('ref_axis',(0.,0.,-1.));
#24831=DIRECTION('',(1.,0.,0.));
#24832=DIRECTION('center_axis',(-1.,0.,0.));
#24833=DIRECTION('ref_axis',(0.,0.,1.));
#24834=DIRECTION('center_axis',(0.,-1.,0.));
#24835=DIRECTION('ref_axis',(0.,0.,-1.));
#24836=DIRECTION('center_axis',(-1.,0.,0.));
#24837=DIRECTION('ref_axis',(0.,0.,-1.));
#24838=DIRECTION('center_axis',(-1.,0.,0.));
#24839=DIRECTION('ref_axis',(0.,0.,-1.));
#24840=DIRECTION('center_axis',(1.,0.,0.));
#24841=DIRECTION('ref_axis',(0.,0.,-1.));
#24842=DIRECTION('center_axis',(1.,0.,0.));
#24843=DIRECTION('ref_axis',(0.,0.,-1.));
#24844=DIRECTION('',(1.,0.,0.));
#24845=DIRECTION('center_axis',(1.,0.,0.));
#24846=DIRECTION('ref_axis',(0.,0.,-1.));
#24847=DIRECTION('center_axis',(0.,-1.,-1.22464679914735E-16));
#24848=DIRECTION('ref_axis',(0.,-1.22464679914735E-16,1.));
#24849=DIRECTION('center_axis',(-1.,0.,0.));
#24850=DIRECTION('ref_axis',(0.,0.,1.));
#24851=DIRECTION('center_axis',(0.,-1.,0.));
#24852=DIRECTION('ref_axis',(0.,0.,-1.));
#24853=DIRECTION('center_axis',(-1.,0.,0.));
#24854=DIRECTION('ref_axis',(0.,0.,1.));
#24855=DIRECTION('center_axis',(0.,-1.,0.));
#24856=DIRECTION('ref_axis',(0.,0.,-1.));
#24857=DIRECTION('center_axis',(-1.,0.,0.));
#24858=DIRECTION('ref_axis',(0.,0.,1.));
#24859=DIRECTION('center_axis',(0.,-1.,0.));
#24860=DIRECTION('ref_axis',(0.,0.,-1.));
#24861=DIRECTION('center_axis',(-1.,0.,0.));
#24862=DIRECTION('ref_axis',(0.,0.,-1.));
#24863=DIRECTION('center_axis',(-1.,0.,0.));
#24864=DIRECTION('ref_axis',(0.,0.,-1.));
#24865=DIRECTION('center_axis',(1.,0.,0.));
#24866=DIRECTION('ref_axis',(0.,0.,-1.));
#24867=DIRECTION('center_axis',(1.,0.,0.));
#24868=DIRECTION('ref_axis',(0.,0.,-1.));
#24869=DIRECTION('',(1.,0.,0.));
#24870=DIRECTION('center_axis',(-1.,0.,0.));
#24871=DIRECTION('ref_axis',(0.,0.,1.));
#24872=DIRECTION('center_axis',(0.,-1.,0.));
#24873=DIRECTION('ref_axis',(0.,0.,-1.));
#24874=DIRECTION('center_axis',(-1.,0.,0.));
#24875=DIRECTION('ref_axis',(0.,0.,1.));
#24876=DIRECTION('center_axis',(0.,-1.,0.));
#24877=DIRECTION('ref_axis',(0.,0.,-1.));
#24878=DIRECTION('center_axis',(1.,0.,0.));
#24879=DIRECTION('ref_axis',(0.,0.,-1.));
#24880=DIRECTION('center_axis',(-1.,0.,0.));
#24881=DIRECTION('ref_axis',(0.,0.,-1.));
#24882=DIRECTION('center_axis',(0.,-1.,0.));
#24883=DIRECTION('ref_axis',(0.,0.,1.));
#24884=DIRECTION('center_axis',(1.,0.,0.));
#24885=DIRECTION('ref_axis',(0.,0.,-1.));
#24886=DIRECTION('center_axis',(1.,0.,0.));
#24887=DIRECTION('ref_axis',(0.,0.,-1.));
#24888=DIRECTION('center_axis',(1.,0.,0.));
#24889=DIRECTION('ref_axis',(0.,0.,-1.));
#24890=DIRECTION('',(1.,0.,0.));
#24891=DIRECTION('center_axis',(1.,0.,0.));
#24892=DIRECTION('ref_axis',(0.,0.,-1.));
#24893=DIRECTION('center_axis',(1.,0.,0.));
#24894=DIRECTION('ref_axis',(0.,0.,-1.));
#24895=DIRECTION('center_axis',(1.,0.,0.));
#24896=DIRECTION('ref_axis',(0.,0.,-1.));
#24897=DIRECTION('center_axis',(-1.,0.,0.));
#24898=DIRECTION('ref_axis',(0.,0.,-1.));
#24899=DIRECTION('center_axis',(0.,-1.,0.));
#24900=DIRECTION('ref_axis',(0.,0.,1.));
#24901=DIRECTION('center_axis',(1.,0.,0.));
#24902=DIRECTION('ref_axis',(0.,0.,-1.));
#24903=DIRECTION('center_axis',(1.,0.,0.));
#24904=DIRECTION('ref_axis',(0.,0.,-1.));
#24905=DIRECTION('center_axis',(1.,0.,0.));
#24906=DIRECTION('ref_axis',(0.,0.,-1.));
#24907=DIRECTION('',(1.,0.,0.));
#24908=DIRECTION('center_axis',(1.,0.,0.));
#24909=DIRECTION('ref_axis',(0.,0.,-1.));
#24910=DIRECTION('center_axis',(1.,0.,0.));
#24911=DIRECTION('ref_axis',(0.,0.,-1.));
#24912=DIRECTION('center_axis',(1.,0.,0.));
#24913=DIRECTION('ref_axis',(0.,0.,-1.));
#24914=DIRECTION('center_axis',(-1.,0.,0.));
#24915=DIRECTION('ref_axis',(0.,0.,-1.));
#24916=DIRECTION('center_axis',(0.,-1.,0.));
#24917=DIRECTION('ref_axis',(0.,0.,1.));
#24918=DIRECTION('center_axis',(1.,0.,0.));
#24919=DIRECTION('ref_axis',(0.,0.,-1.));
#24920=DIRECTION('center_axis',(1.,0.,0.));
#24921=DIRECTION('ref_axis',(0.,0.,-1.));
#24922=DIRECTION('center_axis',(1.,0.,0.));
#24923=DIRECTION('ref_axis',(0.,0.,-1.));
#24924=DIRECTION('',(1.,0.,0.));
#24925=DIRECTION('center_axis',(1.,0.,0.));
#24926=DIRECTION('ref_axis',(0.,0.,-1.));
#24927=DIRECTION('center_axis',(1.,0.,0.));
#24928=DIRECTION('ref_axis',(0.,0.,-1.));
#24929=DIRECTION('center_axis',(0.,0.707106781186548,-0.707106781186547));
#24930=DIRECTION('ref_axis',(0.707106781186547,-0.5,-0.5));
#24931=DIRECTION('',(0.,-0.707106781186548,0.707106781186547));
#24932=DIRECTION('center_axis',(0.,0.707106781186548,-0.707106781186548));
#24933=DIRECTION('ref_axis',(1.,0.,0.));
#24934=DIRECTION('',(0.,0.707106781186548,-0.707106781186547));
#24935=DIRECTION('center_axis',(0.,-0.707106781186548,-0.707106781186547));
#24936=DIRECTION('ref_axis',(0.707106781186547,-0.5,0.5));
#24937=DIRECTION('center_axis',(0.,0.707106781186548,0.707106781186548));
#24938=DIRECTION('ref_axis',(0.,-0.707106781186548,0.707106781186548));
#24939=DIRECTION('',(0.,0.707106781186548,0.707106781186547));
#24940=DIRECTION('center_axis',(0.,0.,1.));
#24941=DIRECTION('ref_axis',(1.,0.,0.));
#24942=DIRECTION('center_axis',(1.,0.,0.));
#24943=DIRECTION('ref_axis',(0.,-1.,0.));
#24944=DIRECTION('center_axis',(0.,-0.707106781186547,-0.707106781186548));
#24945=DIRECTION('ref_axis',(0.,0.707106781186548,-0.707106781186547));
#24946=DIRECTION('',(0.,0.707106781186548,-0.707106781186547));
#24947=DIRECTION('',(1.,0.,0.));
#24948=DIRECTION('',(0.,-0.707106781186548,0.707106781186547));
#24949=DIRECTION('center_axis',(1.,0.,0.));
#24950=DIRECTION('ref_axis',(0.,-1.,0.));
#24951=DIRECTION('center_axis',(-1.,0.,0.));
#24952=DIRECTION('ref_axis',(0.,-1.,0.));
#24953=DIRECTION('center_axis',(1.,0.,0.));
#24954=DIRECTION('ref_axis',(0.,0.,-1.));
#24955=DIRECTION('center_axis',(-1.,0.,0.));
#24956=DIRECTION('ref_axis',(0.,-1.,1.83697019872103E-16));
#24957=DIRECTION('center_axis',(-1.,0.,0.));
#24958=DIRECTION('ref_axis',(0.,-1.,1.83697019872103E-16));
#24959=DIRECTION('center_axis',(0.,-1.,-1.22464679914735E-16));
#24960=DIRECTION('ref_axis',(0.,-1.22464679914735E-16,1.));
#24961=DIRECTION('center_axis',(1.,0.,0.));
#24962=DIRECTION('ref_axis',(0.,-1.,3.06161699786838E-17));
#24963=DIRECTION('center_axis',(1.,0.,0.));
#24964=DIRECTION('ref_axis',(0.,-1.,3.06161699786838E-17));
#24965=DIRECTION('center_axis',(1.,0.,0.));
#24966=DIRECTION('ref_axis',(0.,1.,0.));
#24967=DIRECTION('',(-0.707106781186545,0.70710678118655,8.65956056235496E-17));
#24968=DIRECTION('center_axis',(-1.,0.,0.));
#24969=DIRECTION('ref_axis',(0.,-1.,3.06161699786838E-17));
#24970=DIRECTION('center_axis',(-1.,0.,0.));
#24971=DIRECTION('ref_axis',(0.,-1.,3.06161699786838E-17));
#24972=DIRECTION('center_axis',(1.,0.,0.));
#24973=DIRECTION('ref_axis',(0.,1.,0.));
#24974=DIRECTION('center_axis',(1.,0.,0.));
#24975=DIRECTION('ref_axis',(0.,-1.,1.83697019872103E-16));
#24976=DIRECTION('',(-1.,0.,0.));
#24977=DIRECTION('center_axis',(1.,0.,0.));
#24978=DIRECTION('ref_axis',(0.,-1.,1.83697019872103E-16));
#24979=DIRECTION('center_axis',(1.,0.,0.));
#24980=DIRECTION('ref_axis',(0.,0.,-1.));
#24981=DIRECTION('center_axis',(0.,-1.,-1.22464679914735E-16));
#24982=DIRECTION('ref_axis',(0.,-1.22464679914735E-16,1.));
#24983=DIRECTION('center_axis',(1.,0.,0.));
#24984=DIRECTION('ref_axis',(0.,-1.,1.83697019872103E-16));
#24985=DIRECTION('center_axis',(-1.,0.,0.));
#24986=DIRECTION('ref_axis',(0.,0.,1.));
#24987=DIRECTION('center_axis',(-1.,0.,0.));
#24988=DIRECTION('ref_axis',(0.,0.,-1.));
#24989=DIRECTION('center_axis',(-1.,0.,0.));
#24990=DIRECTION('ref_axis',(0.,0.,-1.));
#24991=DIRECTION('center_axis',(1.,0.,0.));
#24992=DIRECTION('ref_axis',(0.,0.,-1.));
#24993=DIRECTION('center_axis',(1.,0.,0.));
#24994=DIRECTION('ref_axis',(0.,0.,-1.));
#24995=DIRECTION('center_axis',(1.,0.,0.));
#24996=DIRECTION('ref_axis',(0.,0.,-1.));
#24997=DIRECTION('center_axis',(-1.,0.,0.));
#24998=DIRECTION('ref_axis',(0.,-1.,1.83697019872103E-16));
#24999=DIRECTION('center_axis',(-1.,0.,0.));
#25000=DIRECTION('ref_axis',(0.,0.,-1.));
#25001=DIRECTION('center_axis',(1.,0.,0.));
#25002=DIRECTION('ref_axis',(0.,0.,-1.));
#25003=DIRECTION('center_axis',(0.,-1.,0.));
#25004=DIRECTION('ref_axis',(0.,0.,1.));
#25005=DIRECTION('center_axis',(1.,0.,0.));
#25006=DIRECTION('ref_axis',(0.,0.,-1.));
#25007=DIRECTION('center_axis',(0.,-1.,0.));
#25008=DIRECTION('ref_axis',(0.,0.,1.));
#25009=DIRECTION('center_axis',(1.,0.,0.));
#25010=DIRECTION('ref_axis',(0.,0.,-1.));
#25011=DIRECTION('center_axis',(0.,-1.,0.));
#25012=DIRECTION('ref_axis',(0.,0.,1.));
#25013=DIRECTION('center_axis',(1.,0.,0.));
#25014=DIRECTION('ref_axis',(0.,0.,-1.));
#25015=DIRECTION('center_axis',(-1.,0.,0.));
#25016=DIRECTION('ref_axis',(0.,-1.,1.83697019872103E-16));
#25017=DIRECTION('center_axis',(-1.,0.,0.));
#25018=DIRECTION('ref_axis',(0.,-1.,1.83697019872103E-16));
#25019=DIRECTION('center_axis',(0.,-1.,-1.22464679914735E-16));
#25020=DIRECTION('ref_axis',(0.,-1.22464679914735E-16,1.));
#25021=DIRECTION('center_axis',(1.,0.,0.));
#25022=DIRECTION('ref_axis',(0.,1.,0.));
#25023=DIRECTION('',(-1.,0.,0.));
#25024=DIRECTION('center_axis',(1.,0.,0.));
#25025=DIRECTION('ref_axis',(0.,-1.,0.));
#25026=DIRECTION('center_axis',(1.,0.,0.));
#25027=DIRECTION('ref_axis',(0.,-1.,0.));
#25028=DIRECTION('center_axis',(-1.,0.,0.));
#25029=DIRECTION('ref_axis',(0.,0.,1.));
#25030=DIRECTION('center_axis',(1.,0.,0.));
#25031=DIRECTION('ref_axis',(0.,-1.,6.12323399573677E-17));
#25032=DIRECTION('center_axis',(0.,-1.,1.22464679914735E-16));
#25033=DIRECTION('ref_axis',(0.,-1.22464679914735E-16,-1.));
#25034=DIRECTION('center_axis',(1.,0.,0.));
#25035=DIRECTION('ref_axis',(0.,-1.,6.12323399573677E-17));
#25036=DIRECTION('center_axis',(-1.,0.,0.));
#25037=DIRECTION('ref_axis',(0.,-1.,0.));
#25038=DIRECTION('',(0.707106781186552,-0.707106781186543,8.65956056235488E-17));
#25039=DIRECTION('center_axis',(-1.,0.,0.));
#25040=DIRECTION('ref_axis',(0.,-1.,6.12323399573677E-17));
#25041=DIRECTION('center_axis',(-1.,0.,0.));
#25042=DIRECTION('ref_axis',(0.,-1.,6.12323399573677E-17));
#25043=DIRECTION('center_axis',(1.,0.,0.));
#25044=DIRECTION('ref_axis',(0.,0.,-1.));
#25045=DIRECTION('center_axis',(0.,-1.,-1.22464679914735E-16));
#25046=DIRECTION('ref_axis',(0.,-1.22464679914735E-16,1.));
#25047=DIRECTION('center_axis',(1.,0.,0.));
#25048=DIRECTION('ref_axis',(0.,0.,-1.));
#25049=DIRECTION('center_axis',(0.,-1.,-1.22464679914735E-16));
#25050=DIRECTION('ref_axis',(0.,-1.22464679914735E-16,1.));
#25051=DIRECTION('center_axis',(1.,0.,0.));
#25052=DIRECTION('ref_axis',(0.,-1.,1.83697019872103E-16));
#25053=DIRECTION('center_axis',(1.,0.,0.));
#25054=DIRECTION('ref_axis',(0.,-1.,1.83697019872103E-16));
#25055=DIRECTION('center_axis',(1.,0.,0.));
#25056=DIRECTION('ref_axis',(0.,1.,0.));
#25057=DIRECTION('center_axis',(-1.,0.,0.));
#25058=DIRECTION('ref_axis',(0.,-1.,0.));
#25059=DIRECTION('',(-1.,0.,0.));
#25060=DIRECTION('center_axis',(-1.,0.,0.));
#25061=DIRECTION('ref_axis',(0.,-1.,0.));
#25062=DIRECTION('center_axis',(1.,0.,0.));
#25063=DIRECTION('ref_axis',(0.,0.,-1.));
#25064=DIRECTION('center_axis',(-1.,0.,0.));
#25065=DIRECTION('ref_axis',(0.,-1.,3.06161699786838E-17));
#25066=DIRECTION('center_axis',(-1.,0.,0.));
#25067=DIRECTION('ref_axis',(0.,-1.,3.06161699786838E-17));
#25068=DIRECTION('center_axis',(0.,-1.,-1.22464679914735E-16));
#25069=DIRECTION('ref_axis',(0.,-1.22464679914735E-16,1.));
#25070=DIRECTION('center_axis',(-1.,0.,0.));
#25071=DIRECTION('ref_axis',(0.,1.,0.));
#25072=DIRECTION('center_axis',(1.,-3.60555815900857E-17,-3.60555815900857E-17));
#25073=DIRECTION('ref_axis',(-5.09902924839489E-17,-0.707106781186547,-0.707106781186548));
#25074=DIRECTION('',(-0.707106781186545,-0.70710678118655,-8.65956056235496E-17));
#25075=DIRECTION('center_axis',(1.,-3.60555815900857E-17,-3.60555815900857E-17));
#25076=DIRECTION('ref_axis',(-5.09902924839489E-17,-0.707106781186547,-0.707106781186548));
#25077=DIRECTION('center_axis',(1.,0.,0.));
#25078=DIRECTION('ref_axis',(0.,0.,-1.));
#25079=DIRECTION('center_axis',(1.,0.,0.));
#25080=DIRECTION('ref_axis',(0.,3.89573857868908E-14,1.));
#25081=DIRECTION('center_axis',(1.,0.,0.));
#25082=DIRECTION('ref_axis',(0.,0.,-1.));
#25083=DIRECTION('center_axis',(-1.,0.,0.));
#25084=DIRECTION('ref_axis',(0.,-0.707106781186547,0.707106781186548));
#25085=DIRECTION('center_axis',(1.,0.,0.));
#25086=DIRECTION('ref_axis',(0.,0.,-1.));
#25087=DIRECTION('center_axis',(-1.,0.,0.));
#25088=DIRECTION('ref_axis',(0.,0.707106781186547,0.707106781186547));
#25089=DIRECTION('center_axis',(1.,0.,0.));
#25090=DIRECTION('ref_axis',(0.,0.,-1.));
#25091=DIRECTION('center_axis',(-1.,0.,0.));
#25092=DIRECTION('ref_axis',(0.,0.707106781186547,-0.707106781186547));
#25093=DIRECTION('center_axis',(-1.,0.,0.));
#25094=DIRECTION('ref_axis',(0.,-0.707106781186547,-0.707106781186548));
#25095=DIRECTION('center_axis',(-1.,0.,0.));
#25096=DIRECTION('ref_axis',(0.,0.,1.));
#25097=DIRECTION('center_axis',(1.,0.,0.));
#25098=DIRECTION('ref_axis',(0.,0.,-1.));
#25099=DIRECTION('center_axis',(0.,-1.,0.));
#25100=DIRECTION('ref_axis',(0.,0.,-1.));
#25101=DIRECTION('center_axis',(-1.,0.,0.));
#25102=DIRECTION('ref_axis',(0.,0.,-1.));
#25103=DIRECTION('center_axis',(-1.,0.,0.));
#25104=DIRECTION('ref_axis',(0.,0.,-1.));
#25105=DIRECTION('center_axis',(1.,0.,0.));
#25106=DIRECTION('ref_axis',(0.,0.,-1.));
#25107=DIRECTION('',(0.,0.707106781186548,0.707106781186548));
#25108=DIRECTION('',(0.,-0.707106781186548,-0.707106781186548));
#25109=DIRECTION('center_axis',(1.,0.,0.));
#25110=DIRECTION('ref_axis',(0.,0.,-1.));
#25111=DIRECTION('center_axis',(1.,0.,0.));
#25112=DIRECTION('ref_axis',(0.,-1.,0.));
#25113=DIRECTION('center_axis',(1.,0.,0.));
#25114=DIRECTION('ref_axis',(0.,0.,-1.));
#25115=DIRECTION('center_axis',(1.,0.,0.));
#25116=DIRECTION('ref_axis',(0.,0.,-1.));
#25117=DIRECTION('',(1.,0.,0.));
#25118=DIRECTION('center_axis',(-1.,0.,0.));
#25119=DIRECTION('ref_axis',(0.,0.,1.));
#25120=DIRECTION('center_axis',(0.,-1.,0.));
#25121=DIRECTION('ref_axis',(0.,0.,-1.));
#25122=DIRECTION('center_axis',(-1.,0.,0.));
#25123=DIRECTION('ref_axis',(0.,0.,-1.));
#25124=DIRECTION('center_axis',(-1.,0.,0.));
#25125=DIRECTION('ref_axis',(0.,0.,-1.));
#25126=DIRECTION('center_axis',(1.,0.,0.));
#25127=DIRECTION('ref_axis',(0.,0.,-1.));
#25128=DIRECTION('',(1.,0.,0.));
#25129=DIRECTION('center_axis',(-1.,0.,0.));
#25130=DIRECTION('ref_axis',(0.,0.,1.));
#25131=DIRECTION('center_axis',(0.,-1.,0.));
#25132=DIRECTION('ref_axis',(0.,0.,-1.));
#25133=DIRECTION('center_axis',(-1.,0.,0.));
#25134=DIRECTION('ref_axis',(0.,0.,-1.));
#25135=DIRECTION('center_axis',(-1.,0.,0.));
#25136=DIRECTION('ref_axis',(0.,0.,-1.));
#25137=DIRECTION('center_axis',(1.,0.,0.));
#25138=DIRECTION('ref_axis',(0.,0.,-1.));
#25139=DIRECTION('',(1.,0.,0.));
#25140=DIRECTION('center_axis',(-1.,0.,0.));
#25141=DIRECTION('ref_axis',(0.,0.,1.));
#25142=DIRECTION('center_axis',(1.,0.,0.));
#25143=DIRECTION('ref_axis',(0.,-1.,6.12323399573676E-17));
#25144=DIRECTION('center_axis',(0.,-1.,1.22464679914735E-16));
#25145=DIRECTION('ref_axis',(0.,-1.22464679914735E-16,-1.));
#25146=DIRECTION('center_axis',(1.,0.,0.));
#25147=DIRECTION('ref_axis',(0.,-1.,6.12323399573676E-17));
#25148=DIRECTION('center_axis',(1.,0.,0.));
#25149=DIRECTION('ref_axis',(0.,-1.,0.));
#25150=DIRECTION('',(0.707106781186548,0.707106781186548,-8.65956056235493E-17));
#25151=DIRECTION('center_axis',(-1.,0.,0.));
#25152=DIRECTION('ref_axis',(0.,-1.,6.12323399573676E-17));
#25153=DIRECTION('center_axis',(-1.,0.,0.));
#25154=DIRECTION('ref_axis',(0.,-1.,6.12323399573676E-17));
#25155=DIRECTION('center_axis',(1.,0.,0.));
#25156=DIRECTION('ref_axis',(0.,0.,-1.));
#25157=DIRECTION('center_axis',(0.,-1.,-1.22464679914735E-16));
#25158=DIRECTION('ref_axis',(0.,-1.22464679914735E-16,1.));
#25159=DIRECTION('center_axis',(0.,-0.908282142847613,-0.41835815873979));
#25160=DIRECTION('ref_axis',(0.,0.41835815873979,-0.908282142847613));
#25161=DIRECTION('',(1.,0.,0.));
#25162=DIRECTION('center_axis',(1.,0.,0.));
#25163=DIRECTION('ref_axis',(0.,-0.41835815873979,0.908282142847614));
#25164=DIRECTION('center_axis',(1.,0.,0.));
#25165=DIRECTION('ref_axis',(0.,0.908282142847613,0.418358158739791));
#25166=DIRECTION('center_axis',(1.,0.,0.));
#25167=DIRECTION('ref_axis',(0.,0.,-1.));
#25168=DIRECTION('center_axis',(1.,0.,0.));
#25169=DIRECTION('ref_axis',(0.,0.,-1.));
#25170=DIRECTION('center_axis',(1.,0.,0.));
#25171=DIRECTION('ref_axis',(0.,0.,-1.));
#25172=DIRECTION('center_axis',(1.,0.,0.));
#25173=DIRECTION('ref_axis',(0.,0.,-1.));
#25174=DIRECTION('center_axis',(0.,0.707106781186548,-0.707106781186548));
#25175=DIRECTION('ref_axis',(0.,0.707106781186548,0.707106781186548));
#25176=DIRECTION('',(0.,-0.707106781186548,-0.707106781186548));
#25177=DIRECTION('center_axis',(1.,0.,0.));
#25178=DIRECTION('ref_axis',(0.,0.,-1.));
#25179=DIRECTION('center_axis',(1.,0.,0.));
#25180=DIRECTION('ref_axis',(0.,0.,-1.));
#25181=DIRECTION('center_axis',(1.,0.,0.));
#25182=DIRECTION('ref_axis',(0.,0.,-1.));
#25183=DIRECTION('center_axis',(1.,0.,0.));
#25184=DIRECTION('ref_axis',(0.,0.,-1.));
#25185=DIRECTION('center_axis',(1.,0.,0.));
#25186=DIRECTION('ref_axis',(0.,0.,-1.));
#25187=DIRECTION('center_axis',(0.,0.707106781186548,-0.707106781186548));
#25188=DIRECTION('ref_axis',(0.,0.707106781186548,0.707106781186548));
#25189=DIRECTION('center_axis',(1.,0.,0.));
#25190=DIRECTION('ref_axis',(0.,1.,0.));
#25191=DIRECTION('',(1.,0.,0.));
#25192=DIRECTION('center_axis',(1.,0.,0.));
#25193=DIRECTION('ref_axis',(0.,0.,-1.));
#25194=DIRECTION('',(-1.,0.,0.));
#25195=DIRECTION('center_axis',(1.,0.,0.));
#25196=DIRECTION('ref_axis',(0.,0.,-1.));
#25197=DIRECTION('',(-1.,0.,0.));
#25198=DIRECTION('center_axis',(1.,0.,0.));
#25199=DIRECTION('ref_axis',(0.,0.,-1.));
#25200=DIRECTION('',(-1.,0.,0.));
#47239=CARTESIAN_POINT('',(0.,0.,0.));
#47240=CARTESIAN_POINT('Origin',(-6.70710678118655,-22.7688383542068,29.1327993848858));
#47241=CARTESIAN_POINT('',(-6.70710678118655,-30.1934595566656,22.4152849636136));
#47242=CARTESIAN_POINT('',(-6.35355339059327,-30.0899061660723,22.3117315730203));
#47243=CARTESIAN_POINT('Origin',(-6.70710678118655,-29.8399061660723,22.0617315730203));
#47244=CARTESIAN_POINT('',(-6.35355339059327,-22.3117315730203,30.0899061660723));
#47245=CARTESIAN_POINT('',(-6.35355339059327,-23.0188383542068,29.3827993848858));
#47246=CARTESIAN_POINT('',(-6.70710678118655,-22.4152849636136,30.1934595566656));
#47247=CARTESIAN_POINT('Origin',(-6.70710678118655,-22.0617315730203,29.8399061660723));
#47248=CARTESIAN_POINT('',(-6.70710678118655,-23.1223917448001,29.486352775479));
#47249=CARTESIAN_POINT('Origin',(-6.70710678118654,-22.0617315730203,29.8399061660723));
#47250=CARTESIAN_POINT('',(-6.35355339059327,-21.8117315730203,30.0899061660723));
#47251=CARTESIAN_POINT('',(-6.70710678118655,-21.708178182427,30.1934595566656));
#47252=CARTESIAN_POINT('Origin',(-6.70710678118655,-22.0617315730203,29.8399061660723));
#47253=CARTESIAN_POINT('Origin',(-6.70710678118654,-22.0617315730203,29.8399061660723));
#47254=CARTESIAN_POINT('Origin',(-6.70710678118654,-22.0617315730203,29.8399061660723));
#47255=CARTESIAN_POINT('Origin',(-5.04640452079103,-27.4913185063573,22.0617315730203));
#47256=CARTESIAN_POINT('',(-6.14644660940673,-29.7970129472589,21.8117315730203));
#47257=CARTESIAN_POINT('',(-6.14644660940673,-29.7970129472589,22.3117315730203));
#47258=CARTESIAN_POINT('Origin',(-6.5,-29.5470129472589,22.0617315730203));
#47259=CARTESIAN_POINT('',(-4.69285113019775,-27.7413185063573,22.3117315730203));
#47260=CARTESIAN_POINT('',(-6.35355339059327,-30.0899061660723,21.8117315730203));
#47261=CARTESIAN_POINT('Origin',(-6.70710678118654,-29.8399061660723,22.0617315730203));
#47262=CARTESIAN_POINT('',(-4.69285113019775,-27.7413185063573,21.8117315730203));
#47263=CARTESIAN_POINT('Origin',(-6.5,-28.4029896810001,20.9177083067616));
#47264=CARTESIAN_POINT('',(-6.14644660940673,-26.4129509039023,18.4276695296637));
#47265=CARTESIAN_POINT('',(-6.,-26.1629509039023,18.6776695296637));
#47266=CARTESIAN_POINT('Origin',(-6.5,-26.1629509039023,18.6776695296637));
#47267=CARTESIAN_POINT('',(-6.,-29.5470129472589,22.0617315730203));
#47268=CARTESIAN_POINT('',(-6.,-28.4029896810001,20.9177083067616));
#47269=CARTESIAN_POINT('Origin',(-6.5,-29.5470129472589,22.0617315730203));
#47270=CARTESIAN_POINT('',(-6.14644660940673,-28.6529896810001,20.6677083067616));
#47271=CARTESIAN_POINT('Origin',(-6.5,-29.5470129472589,22.0617315730203));
#47272=CARTESIAN_POINT('Origin',(-6.5,-29.5470129472589,22.0617315730203));
#47273=CARTESIAN_POINT('Origin',(-6.70710678118655,-18.3847763108502,26.1629509039023));
#47274=CARTESIAN_POINT('',(-6.35355339059327,-18.1347763108502,26.4129509039023));
#47275=CARTESIAN_POINT('',(-6.70710678118655,-18.031222920257,26.5165042944955));
#47276=CARTESIAN_POINT('Origin',(-6.70710678118655,-18.3847763108502,26.1629509039023));
#47277=CARTESIAN_POINT('',(-6.35355339059327,-18.1347763108502,25.9129509039023));
#47278=CARTESIAN_POINT('Origin',(-6.70710678118655,-18.3847763108502,26.1629509039023));
#47279=CARTESIAN_POINT('',(-6.70710678118655,-18.031222920257,25.809397513309));
#47280=CARTESIAN_POINT('Origin',(-6.70710678118655,-18.3847763108502,26.1629509039023));
#47281=CARTESIAN_POINT('Origin',(-6.70710678118655,-18.3847763108502,26.1629509039023));
#47282=CARTESIAN_POINT('Origin',(-6.70710678118655,-25.4558441227157,19.0918830920368));
#47283=CARTESIAN_POINT('',(-6.35355339059327,-25.9129509039023,18.1347763108502));
#47284=CARTESIAN_POINT('',(-6.70710678118655,-25.809397513309,18.031222920257));
#47285=CARTESIAN_POINT('Origin',(-6.70710678118655,-26.1629509039023,18.3847763108502));
#47286=CARTESIAN_POINT('',(-6.70710678118655,-25.1022907321224,18.7383297014435));
#47287=CARTESIAN_POINT('',(-6.35355339059327,-25.2058441227157,18.8418830920368));
#47288=CARTESIAN_POINT('Origin',(-5.52973785412436,-26.1629509039023,20.0498274154182));
#47289=CARTESIAN_POINT('',(-6.14644660940673,-25.9129509039023,18.4276695296637));
#47290=CARTESIAN_POINT('Origin',(-6.5,-26.1629509039023,18.6776695296637));
#47291=CARTESIAN_POINT('',(-6.35355339059327,-26.4129509039023,18.1347763108502));
#47292=CARTESIAN_POINT('',(-5.17618446353109,-26.4129509039023,19.7998274154182));
#47293=CARTESIAN_POINT('Origin',(-6.70710678118655,-26.1629509039023,18.3847763108502));
#47294=CARTESIAN_POINT('',(-5.17618446353109,-25.9129509039023,19.7998274154182));
#47295=CARTESIAN_POINT('Origin',(-6.5,-26.1629509039022,18.6776695296637));
#47296=CARTESIAN_POINT('Origin',(-6.5,-26.1629509039022,18.6776695296637));
#47297=CARTESIAN_POINT('Origin',(-5.52973785412436,-22.0617315730203,28.1748550615043));
#47298=CARTESIAN_POINT('',(-6.14644660940673,-22.3117315730203,29.7970129472589));
#47299=CARTESIAN_POINT('',(-5.17618446353109,-22.3117315730203,28.4248550615043));
#47300=CARTESIAN_POINT('',(-6.14644660940673,-21.8117315730203,29.7970129472589));
#47301=CARTESIAN_POINT('Origin',(-6.5,-22.0617315730203,29.5470129472589));
#47302=CARTESIAN_POINT('',(-5.17618446353109,-21.8117315730203,28.4248550615043));
#47303=CARTESIAN_POINT('Origin',(-6.25,-24.0062752212833,28.2489159084026));
#47304=CARTESIAN_POINT('',(-6.14644660940673,-24.9937120883597,27.1150324319194));
#47305=CARTESIAN_POINT('Origin',(-6.5,-24.7437120883598,26.8650324319194));
#47306=CARTESIAN_POINT('',(-6.,-22.0617315730203,29.5470129472589));
#47307=CARTESIAN_POINT('',(-6.,-24.7437120883598,26.8650324319194));
#47308=CARTESIAN_POINT('Origin',(-6.5,-22.0617315730203,29.5470129472589));
#47309=CARTESIAN_POINT('Origin',(-6.,-24.1123412384613,24.1123412384613));
#47310=CARTESIAN_POINT('',(-6.,-18.6776695296637,26.1629509039023));
#47311=CARTESIAN_POINT('',(-6.,-23.4809703885628,21.3596500450031));
#47312=CARTESIAN_POINT('',(-6.,-19.8216927959224,27.306974170161));
#47313=CARTESIAN_POINT('Origin',(-6.5,-23.4809703885628,21.3596500450031));
#47314=CARTESIAN_POINT('',(-6.14644660940673,-18.4276695296637,25.9129509039023));
#47315=CARTESIAN_POINT('',(-6.14644660940673,-23.2309703885628,21.1096500450031));
#47316=CARTESIAN_POINT('Origin',(-6.5,-18.6776695296637,26.1629509039023));
#47317=CARTESIAN_POINT('Origin',(-6.25,-24.2184072556392,19.97576656852));
#47318=CARTESIAN_POINT('',(-4.69285113019775,-20.4833639705652,25.9129509039023));
#47319=CARTESIAN_POINT('Origin',(-6.70710678118655,-18.5792306756765,26.3574052687286));
#47320=CARTESIAN_POINT('',(-6.35355339059327,-18.3292306756765,26.6074052687286));
#47321=CARTESIAN_POINT('',(-6.70710678118655,-18.2256772850833,26.7109586593218));
#47322=CARTESIAN_POINT('Origin',(-5.04640452079103,-20.7333639705652,26.1629509039023));
#47323=CARTESIAN_POINT('',(-6.14644660940673,-18.4276695296637,26.4129509039023));
#47324=CARTESIAN_POINT('',(-4.69285113019775,-20.4833639705652,26.4129509039023));
#47325=CARTESIAN_POINT('Origin',(-6.5,-18.6776695296637,26.1629509039023));
#47326=CARTESIAN_POINT('Origin',(-6.5,-22.0617315730203,29.5470129472589));
#47327=CARTESIAN_POINT('Origin',(-6.5,-22.0617315730203,29.5470129472589));
#47328=CARTESIAN_POINT('Origin',(-6.25,-18.9504617357995,27.0821897194448));
#47329=CARTESIAN_POINT('',(-6.14644660940673,-19.5716927959224,27.556974170161));
#47330=CARTESIAN_POINT('Origin',(-6.5,-19.8216927959224,27.306974170161));
#47331=CARTESIAN_POINT('Origin',(-6.5,-18.6776695296637,26.1629509039023));
#47332=CARTESIAN_POINT('Origin',(-6.25,-29.2742207411231,21.1424927574778));
#47333=CARTESIAN_POINT('',(-6.35355339059327,-29.895451801246,21.617277208194));
#47334=CARTESIAN_POINT('Origin',(-14.,-29.8399061660723,22.0617315730203));
#47335=CARTESIAN_POINT('',(-10.0449101394378,-30.1934595566656,22.4152849636136));
#47336=CARTESIAN_POINT('',(-10.146446609406,-30.2815079190287,22.2962265447912));
#47337=CARTESIAN_POINT('Ctrl Pts',(-10.146446609406,-30.2815079190287,22.2962265447912));
#47338=CARTESIAN_POINT('Ctrl Pts',(-10.1126391838745,-30.264925350508,22.3274548959663));
#47339=CARTESIAN_POINT('Ctrl Pts',(-10.0811424950941,-30.2405707165373,
22.3636229983165));
#47340=CARTESIAN_POINT('Ctrl Pts',(-10.0542643495493,-30.2071640058445,
22.4011569393069));
#47341=CARTESIAN_POINT('Ctrl Pts',(-10.0494504338405,-30.200514147943,22.4082303723361));
#47342=CARTESIAN_POINT('Ctrl Pts',(-10.0449101394378,-30.1934595566656,
22.4152849636136));
#47343=CARTESIAN_POINT('',(-10.3535533905933,-30.3399061660723,22.0617315730203));
#47344=CARTESIAN_POINT('Origin',(-10.,-29.8399061660723,22.0617315730203));
#47345=CARTESIAN_POINT('',(-10.7071067811865,-30.1934595566656,21.708178182427));
#47346=CARTESIAN_POINT('Origin',(-10.7071067811865,-29.8399061660723,22.0617315730203));
#47347=CARTESIAN_POINT('',(-6.70710678118655,-30.1934595566656,21.708178182427));
#47348=CARTESIAN_POINT('',(-14.,-30.1934595566656,21.708178182427));
#47349=CARTESIAN_POINT('Origin',(-6.70710678118655,-29.8399061660723,22.0617315730203));
#47350=CARTESIAN_POINT('',(-14.,-30.1934595566656,22.4152849636136));
#47351=CARTESIAN_POINT('Origin',(-6.70710678118655,-29.8399061660723,22.0617315730203));
#47352=CARTESIAN_POINT('Origin',(-6.70710678118655,-29.8399061660723,22.0617315730203));
#47353=CARTESIAN_POINT('Origin',(-14.,-22.0617315730203,30.5470129472589));
#47354=CARTESIAN_POINT('',(-10.0449101394378,-22.4152849636135,30.1934595566656));
#47355=CARTESIAN_POINT('',(-14.,-22.4152849636136,30.1934595566656));
#47356=CARTESIAN_POINT('',(-10.,-22.5617315730203,30.0470129472588));
#47357=CARTESIAN_POINT('Origin',(-10.5,-22.5617315730203,30.0470129472588));
#47358=CARTESIAN_POINT('',(-10.,-30.0470129472589,22.5617315730203));
#47359=CARTESIAN_POINT('',(-10.,-24.1830519165799,28.4256926036992));
#47360=CARTESIAN_POINT('Origin',(-10.5,-30.0470129472588,22.5617315730203));
#47361=CARTESIAN_POINT('Origin',(-6.70710678118655,-29.645451801246,21.867277208194));
#47362=CARTESIAN_POINT('',(-6.70710678118655,-26.5165042944955,18.031222920257));
#47363=CARTESIAN_POINT('',(-6.70710678118655,-29.9990051918393,21.5137238176007));
#47364=CARTESIAN_POINT('Origin',(-6.70710678118655,-26.1629509039023,18.3847763108502));
#47365=CARTESIAN_POINT('Origin',(-6.70710678118655,-26.1629509039023,18.3847763108502));
#47366=CARTESIAN_POINT('Origin',(-6.70710678118655,-26.1629509039023,18.3847763108502));
#47367=CARTESIAN_POINT('Origin',(-14.,-26.1629509039023,18.3847763108502));
#47368=CARTESIAN_POINT('',(-14.,-26.5165042944955,18.031222920257));
#47369=CARTESIAN_POINT('',(-14.,-26.5165042944955,18.031222920257));
#47370=CARTESIAN_POINT('',(-14.,-25.809397513309,18.031222920257));
#47371=CARTESIAN_POINT('Origin',(-14.,-26.1629509039023,18.3847763108502));
#47372=CARTESIAN_POINT('',(-14.,-25.809397513309,18.031222920257));
#47373=CARTESIAN_POINT('Origin',(-14.,-30.5470129472589,22.0617315730203));
#47374=CARTESIAN_POINT('',(-10.7071067811865,-34.2946788875476,25.809397513309));
#47375=CARTESIAN_POINT('',(-10.7071067811865,-31.0419876940894,22.5567063198509));
#47376=CARTESIAN_POINT('',(-14.,-34.2946788875476,25.809397513309));
#47377=CARTESIAN_POINT('',(-14.,-34.2946788875476,25.809397513309));
#47378=CARTESIAN_POINT('',(-14.,-14.3948268171891,5.90954544295051));
#47379=CARTESIAN_POINT('Origin',(-10.7071067811865,-33.9411254969543,26.1629509039023));
#47380=CARTESIAN_POINT('',(-10.3535533905933,-34.1911254969543,26.4129509039023));
#47381=CARTESIAN_POINT('',(-10.7071067811865,-34.2946788875476,26.5165042944955));
#47382=CARTESIAN_POINT('Origin',(-10.7071067811865,-33.9411254969543,26.1629509039022));
#47383=CARTESIAN_POINT('Origin',(-10.7071067811865,-33.9411254969543,26.1629509039023));
#47384=CARTESIAN_POINT('',(-10.3535533905933,-34.1911254969543,25.9129509039023));
#47385=CARTESIAN_POINT('Origin',(-10.7071067811865,-33.9411254969543,26.1629509039023));
#47386=CARTESIAN_POINT('Origin',(-10.7071067811865,-33.9411254969543,26.1629509039023));
#47387=CARTESIAN_POINT('Origin',(-10.7071067811865,-30.6884343034962,22.9102597104441));
#47388=CARTESIAN_POINT('',(-10.3535533905933,-30.9384343034962,22.6602597104441));
#47389=CARTESIAN_POINT('Origin',(-14.,-33.9411254969543,26.1629509039023));
#47390=CARTESIAN_POINT('',(-14.025428935758,-34.2946788875476,26.5165042944955));
#47391=CARTESIAN_POINT('',(-14.,-34.2946788875476,26.5165042944955));
#47392=CARTESIAN_POINT('',(-14.,-34.4335120598975,26.0760286821578));
#47393=CARTESIAN_POINT('Ctrl Pts',(-14.,-34.4335120598975,26.0760286821577));
#47394=CARTESIAN_POINT('Ctrl Pts',(-14.,-34.439576740978,26.110383159214));
#47395=CARTESIAN_POINT('Ctrl Pts',(-14.0019573651892,-34.4420465318245,
26.1453834686124));
#47396=CARTESIAN_POINT('Ctrl Pts',(-14.0094015207423,-34.4388040888907,
26.2380233090204));
#47397=CARTESIAN_POINT('Ctrl Pts',(-14.0161612500453,-34.4268763441737,
26.2948454509909));
#47398=CARTESIAN_POINT('Ctrl Pts',(-14.0245143380439,-34.3882911628533,
26.3913434645052));
#47399=CARTESIAN_POINT('Ctrl Pts',(-14.026804427637,-34.3653919660536,26.4315414345033));
#47400=CARTESIAN_POINT('Ctrl Pts',(-14.026804427637,-34.3371305955527,26.4682048340719));
#47401=CARTESIAN_POINT('Ctrl Pts',(-14.026804427637,-34.3239946581065,26.4852460502184));
#47402=CARTESIAN_POINT('Ctrl Pts',(-14.0263298822064,-34.3098160327091,
26.501367149334));
#47403=CARTESIAN_POINT('Ctrl Pts',(-14.025428935758,-34.2946788875475,26.5165042944956));
#47404=CARTESIAN_POINT('Origin',(-14.,-33.9411254969543,26.1629509039023));
#47405=CARTESIAN_POINT('Origin',(-10.7071067811865,-26.8700576850888,33.2340187157677));
#47406=CARTESIAN_POINT('',(-10.3535533905933,-26.4129509039023,34.1911254969543));
#47407=CARTESIAN_POINT('',(-10.3535533905933,-27.1200576850888,33.4840187157677));
#47408=CARTESIAN_POINT('',(-10.7071067811866,-26.5165042944955,34.2946788875476));
#47409=CARTESIAN_POINT('Origin',(-10.7071067811865,-26.1629509039023,33.9411254969543));
#47410=CARTESIAN_POINT('',(-10.7071067811865,-27.2236110756821,33.587572106361));
#47411=CARTESIAN_POINT('Origin',(-8.57140452079103,-30.9207863951121,26.1629509039023));
#47412=CARTESIAN_POINT('',(-10.1464466094067,-33.8982322781408,25.9129509039023));
#47413=CARTESIAN_POINT('',(-8.21785113019776,-31.1707863951121,25.9129509039023));
#47414=CARTESIAN_POINT('',(-10.1464466094067,-33.8982322781408,26.4129509039023));
#47415=CARTESIAN_POINT('Origin',(-10.5,-33.6482322781408,26.1629509039023));
#47416=CARTESIAN_POINT('',(-8.21785113019776,-31.1707863951121,26.4129509039023));
#47417=CARTESIAN_POINT('Origin',(-10.5,-31.5319371877506,24.046655813512));
#47418=CARTESIAN_POINT('',(-10.,-33.6482322781408,26.1629509039023));
#47419=CARTESIAN_POINT('Origin',(-10.5,-33.6482322781408,26.1629509039023));
#47420=CARTESIAN_POINT('',(-10.1464466094067,-31.7819371877506,23.796655813512));
#47421=CARTESIAN_POINT('',(-10.,-31.5319371877506,24.046655813512));
#47422=CARTESIAN_POINT('Origin',(-10.5,-33.6482322781408,26.1629509039023));
#47423=CARTESIAN_POINT('Origin',(-10.5,-33.6482322781408,26.1629509039023));
#47424=CARTESIAN_POINT('Origin',(-10.25,-28.1074945521653,32.3501352392845));
#47425=CARTESIAN_POINT('',(-10.1464466094067,-26.4129509039023,33.8982322781408));
#47426=CARTESIAN_POINT('',(-10.1464466094067,-29.0949314192417,31.2162517628014));
#47427=CARTESIAN_POINT('',(-8.7011844635311,-26.4129509039023,31.8543229502591));
#47428=CARTESIAN_POINT('Origin',(-10.5,-28.8449314192417,30.9662517628014));
#47429=CARTESIAN_POINT('',(-10.,-26.1629509039023,33.6482322781408));
#47430=CARTESIAN_POINT('',(-10.,-28.8449314192417,30.9662517628014));
#47431=CARTESIAN_POINT('Origin',(-10.5,-26.1629509039023,33.6482322781408));
#47432=CARTESIAN_POINT('Origin',(-10.,-28.2842712474619,28.2842712474619));
#47433=CARTESIAN_POINT('',(-10.,-22.9506403026729,30.4359216769114));
#47434=CARTESIAN_POINT('Origin',(-6.5,-18.6776695296637,26.1629509039023));
#47435=CARTESIAN_POINT('Origin',(-14.,-18.3847763108502,26.1629509039023));
#47436=CARTESIAN_POINT('',(-14.,-18.031222920257,25.809397513309));
#47437=CARTESIAN_POINT('',(-14.,-18.031222920257,25.809397513309));
#47438=CARTESIAN_POINT('',(-14.,-18.031222920257,26.5165042944955));
#47439=CARTESIAN_POINT('Origin',(-14.,-18.3847763108502,26.1629509039023));
#47440=CARTESIAN_POINT('',(-14.,-18.031222920257,26.5165042944955));
#47441=CARTESIAN_POINT('Origin',(-14.,-17.6776695296637,26.1629509039023));
#47442=CARTESIAN_POINT('',(-14.,-25.809397513309,34.2946788875476));
#47443=CARTESIAN_POINT('',(-14.,-3.71751442127221,12.2027957955108));
#47444=CARTESIAN_POINT('',(-10.7071067811866,-25.809397513309,34.2946788875476));
#47445=CARTESIAN_POINT('',(-14.,-25.809397513309,34.2946788875476));
#47446=CARTESIAN_POINT('',(-10.7071067811866,-21.708178182427,30.1934595566656));
#47447=CARTESIAN_POINT('',(-10.7071067811866,-19.2686597873334,27.753941161572));
#47448=CARTESIAN_POINT('',(-14.,-21.708178182427,30.1934595566656));
#47449=CARTESIAN_POINT('Origin',(-14.,-22.0617315730203,29.8399061660723));
#47450=CARTESIAN_POINT('',(-10.3535533905933,-22.0617315730203,30.3399061660723));
#47451=CARTESIAN_POINT('Origin',(-10.7071067811866,-22.0617315730203,29.8399061660723));
#47452=CARTESIAN_POINT('',(-10.146446609406,-22.2962265447912,30.2815079190287));
#47453=CARTESIAN_POINT('Origin',(-10.,-22.0617315730203,29.8399061660723));
#47454=CARTESIAN_POINT('Ctrl Pts',(-10.0449101394378,-22.4152849636136,
30.1934595566656));
#47455=CARTESIAN_POINT('Ctrl Pts',(-10.0494504338405,-22.4082303723361,
30.200514147943));
#47456=CARTESIAN_POINT('Ctrl Pts',(-10.0542643495493,-22.4011569393069,
30.2071640058445));
#47457=CARTESIAN_POINT('Ctrl Pts',(-10.081142495094,-22.3636229983167,30.2405707165371));
#47458=CARTESIAN_POINT('Ctrl Pts',(-10.1126391838741,-22.3274548959667,
30.2649253505077));
#47459=CARTESIAN_POINT('Ctrl Pts',(-10.1464466094053,-22.2962265447918,
30.2815079190284));
#47460=CARTESIAN_POINT('Origin',(-10.5,-22.9506403026729,30.4359216769114));
#47461=CARTESIAN_POINT('',(-10.1464466094067,-25.9129509039023,33.8982322781408));
#47462=CARTESIAN_POINT('Origin',(-10.5,-26.1629509039023,33.6482322781408));
#47463=CARTESIAN_POINT('',(-10.1464466094067,-22.7006403026729,30.6859216769114));
#47464=CARTESIAN_POINT('Origin',(-10.5,-26.1629509039023,33.6482322781408));
#47465=CARTESIAN_POINT('Origin',(-10.5,-26.1629509039023,33.6482322781408));
#47466=CARTESIAN_POINT('Origin',(-9.05473785412437,-26.1629509039023,31.6043229502591));
#47467=CARTESIAN_POINT('',(-10.3535533905933,-25.9129509039023,34.1911254969543));
#47468=CARTESIAN_POINT('Origin',(-10.7071067811865,-26.1629509039023,33.9411254969543));
#47469=CARTESIAN_POINT('',(-8.70118446353109,-25.9129509039023,31.8543229502591));
#47470=CARTESIAN_POINT('Origin',(-14.,-26.1629509039023,34.6482322781408));
#47471=CARTESIAN_POINT('',(-14.025428935758,-26.5165042944955,34.2946788875476));
#47472=CARTESIAN_POINT('',(-14.,-26.5165042944955,34.2946788875476));
#47473=CARTESIAN_POINT('',(-14.,-27.5223620986102,33.2888210834329));
#47474=CARTESIAN_POINT('Ctrl Pts',(-14.025428935758,-26.5165042944955,34.2946788875476));
#47475=CARTESIAN_POINT('Ctrl Pts',(-14.0048893955981,-26.8615969484775,
33.9495862335655));
#47476=CARTESIAN_POINT('Ctrl Pts',(-14.,-27.2050511579839,33.6061320240592));
#47477=CARTESIAN_POINT('Ctrl Pts',(-14.,-27.5223620986102,33.2888210834329));
#47478=CARTESIAN_POINT('',(-14.,-33.2888210834329,27.5223620986102));
#47479=CARTESIAN_POINT('',(-14.,-25.2842712474619,35.5269119345812));
#47480=CARTESIAN_POINT('Ctrl Pts',(-14.,-33.2888210834329,27.5223620986102));
#47481=CARTESIAN_POINT('Ctrl Pts',(-14.,-33.6061320240592,27.2050511579839));
#47482=CARTESIAN_POINT('Ctrl Pts',(-14.0048893955981,-33.9495862335655,
26.8615969484775));
#47483=CARTESIAN_POINT('Ctrl Pts',(-14.025428935758,-34.2946788875476,26.5165042944955));
#47484=CARTESIAN_POINT('Origin',(-10.25,-31.3601857456234,23.2284577619781));
#47485=CARTESIAN_POINT('Origin',(-10.7071067811866,-19.6222131779267,27.4003877709787));
#47486=CARTESIAN_POINT('Origin',(-10.7071067811866,-26.1629509039023,33.9411254969543));
#47487=CARTESIAN_POINT('',(-10.3535533905933,-19.3722131779267,27.6503877709787));
#47488=CARTESIAN_POINT('Origin',(-10.7071067811866,-26.1629509039023,33.9411254969543));
#47489=CARTESIAN_POINT('Origin',(-10.7071067811866,-26.1629509039023,33.9411254969543));
#47490=CARTESIAN_POINT('Origin',(-14.,-26.1629509039023,33.9411254969543));
#47491=CARTESIAN_POINT('',(-14.,-26.0760286821578,34.4335120598975));
#47492=CARTESIAN_POINT('Origin',(-14.,-26.1629509039023,33.9411254969543));
#47493=CARTESIAN_POINT('Ctrl Pts',(-14.025428935758,-26.5165042944955,34.2946788875476));
#47494=CARTESIAN_POINT('Ctrl Pts',(-14.0263293530702,-26.501376039553,34.3098071424901));
#47495=CARTESIAN_POINT('Ctrl Pts',(-14.0268044276371,-26.4852549680463,
34.3239877839475));
#47496=CARTESIAN_POINT('Ctrl Pts',(-14.0268044276371,-26.4682048340719,
34.3371305955528));
#47497=CARTESIAN_POINT('Ctrl Pts',(-14.0268044276371,-26.4359460827031,
34.3619967163995));
#47498=CARTESIAN_POINT('Ctrl Pts',(-14.0250516964297,-26.4009212026149,
34.3827322393151));
#47499=CARTESIAN_POINT('Ctrl Pts',(-14.0179720411043,-26.3124348467826,
34.4215374836553));
#47500=CARTESIAN_POINT('Ctrl Pts',(-14.0115803121848,-26.2577402477616,
34.4352140696344));
#47501=CARTESIAN_POINT('Ctrl Pts',(-14.0028573458318,-26.1599875313315,
34.4429028780862));
#47502=CARTESIAN_POINT('Ctrl Pts',(-14.,-26.1175962104965,34.4408500788191));
#47503=CARTESIAN_POINT('Ctrl Pts',(-14.,-26.0760286821578,34.4335120598975));
#47504=CARTESIAN_POINT('Origin',(-10.25,-21.0364267402998,29.1681547239451));
#47505=CARTESIAN_POINT('Origin',(-14.,26.1629509039023,18.3847763108502));
#47506=CARTESIAN_POINT('',(-6.70710678118655,26.5165042944955,18.031222920257));
#47507=CARTESIAN_POINT('',(-6.70710678118655,25.809397513309,18.031222920257));
#47508=CARTESIAN_POINT('Origin',(-6.70710678118655,26.1629509039023,18.3847763108502));
#47509=CARTESIAN_POINT('',(-14.,25.809397513309,18.031222920257));
#47510=CARTESIAN_POINT('',(-14.,25.809397513309,18.031222920257));
#47511=CARTESIAN_POINT('',(-14.,26.5165042944955,18.031222920257));
#47512=CARTESIAN_POINT('Origin',(-14.,26.1629509039023,18.3847763108502));
#47513=CARTESIAN_POINT('',(-14.,26.5165042944955,18.031222920257));
#47514=CARTESIAN_POINT('Origin',(-6.70710678118654,26.3574052687286,18.5792306756765));
#47515=CARTESIAN_POINT('',(-6.35355339059328,26.4129509039023,18.1347763108502));
#47516=CARTESIAN_POINT('Origin',(-6.70710678118654,26.1629509039023,18.3847763108502));
#47517=CARTESIAN_POINT('',(-6.70710678118654,30.1934595566656,21.708178182427));
#47518=CARTESIAN_POINT('',(-6.70710678118654,26.7109586593218,18.2256772850833));
#47519=CARTESIAN_POINT('',(-6.35355339059327,30.0899061660723,21.8117315730203));
#47520=CARTESIAN_POINT('Origin',(-6.70710678118654,29.8399061660723,22.0617315730203));
#47521=CARTESIAN_POINT('',(-6.35355339059327,26.6074052687286,18.3292306756765));
#47522=CARTESIAN_POINT('Origin',(-6.70710678118654,29.8399061660723,22.0617315730203));
#47523=CARTESIAN_POINT('',(-6.35355339059327,30.0899061660723,22.3117315730203));
#47524=CARTESIAN_POINT('',(-6.70710678118655,30.1934595566656,22.4152849636136));
#47525=CARTESIAN_POINT('Origin',(-6.70710678118655,29.8399061660723,22.0617315730203));
#47526=CARTESIAN_POINT('Origin',(-6.70710678118654,29.8399061660723,22.0617315730203));
#47527=CARTESIAN_POINT('Origin',(-6.70710678118654,29.8399061660723,22.0617315730203));
#47528=CARTESIAN_POINT('Origin',(-14.,17.6776695296637,26.1629509039023));
#47529=CARTESIAN_POINT('',(-6.70710678118655,18.031222920257,25.809397513309));
#47530=CARTESIAN_POINT('',(-6.70710678118655,18.7383297014435,25.1022907321224));
#47531=CARTESIAN_POINT('',(-14.,18.031222920257,25.809397513309));
#47532=CARTESIAN_POINT('',(-14.,18.031222920257,25.809397513309));
#47533=CARTESIAN_POINT('',(-14.,22.7989898732233,21.0416305603426));
#47534=CARTESIAN_POINT('Origin',(-6.25,27.0821897194448,18.9504617357995));
#47535=CARTESIAN_POINT('',(-6.14644660940673,29.7970129472589,21.8117315730203));
#47536=CARTESIAN_POINT('',(-5.17618446353109,28.4248550615043,21.8117315730203));
#47537=CARTESIAN_POINT('',(-6.14644660940673,26.4129509039023,18.4276695296637));
#47538=CARTESIAN_POINT('',(-6.14644660940673,27.556974170161,19.5716927959224));
#47539=CARTESIAN_POINT('',(-4.69285113019775,26.4129509039023,20.4833639705652));
#47540=CARTESIAN_POINT('Origin',(-5.04640452079103,26.1629509039023,20.7333639705652));
#47541=CARTESIAN_POINT('',(-6.35355339059327,25.9129509039023,18.1347763108502));
#47542=CARTESIAN_POINT('Origin',(-6.70710678118655,26.1629509039023,18.3847763108502));
#47543=CARTESIAN_POINT('',(-6.14644660940673,25.9129509039023,18.4276695296637));
#47544=CARTESIAN_POINT('Origin',(-6.5,26.1629509039023,18.6776695296637));
#47545=CARTESIAN_POINT('',(-4.69285113019775,25.9129509039023,20.4833639705652));
#47546=CARTESIAN_POINT('Origin',(-6.70710678118655,26.1629509039023,18.3847763108502));
#47547=CARTESIAN_POINT('Origin',(-6.70710678118655,26.1629509039023,18.3847763108502));
#47548=CARTESIAN_POINT('Origin',(-6.5,27.306974170161,19.8216927959224));
#47549=CARTESIAN_POINT('',(-6.,29.5470129472589,22.0617315730203));
#47550=CARTESIAN_POINT('Origin',(-6.5,29.5470129472589,22.0617315730203));
#47551=CARTESIAN_POINT('',(-6.,26.1629509039023,18.6776695296637));
#47552=CARTESIAN_POINT('',(-6.,27.306974170161,19.8216927959224));
#47553=CARTESIAN_POINT('Origin',(-6.5,26.1629509039023,18.6776695296637));
#47554=CARTESIAN_POINT('Origin',(-6.5,26.1629509039023,18.6776695296637));
#47555=CARTESIAN_POINT('Origin',(-6.5,26.1629509039023,18.6776695296637));
#47556=CARTESIAN_POINT('Origin',(-5.52973785412436,28.1748550615043,22.0617315730203));
#47557=CARTESIAN_POINT('',(-6.14644660940673,29.7970129472589,22.3117315730203));
#47558=CARTESIAN_POINT('',(-5.17618446353109,28.4248550615043,22.3117315730203));
#47559=CARTESIAN_POINT('Origin',(-6.5,29.5470129472589,22.0617315730203));
#47560=CARTESIAN_POINT('Origin',(-6.5,29.5470129472589,22.0617315730203));
#47561=CARTESIAN_POINT('Origin',(-6.5,29.5470129472589,22.0617315730203));
#47562=CARTESIAN_POINT('Origin',(-6.70710678118655,19.0918830920368,25.4558441227157));
#47563=CARTESIAN_POINT('',(-6.35355339059327,18.1347763108502,25.9129509039023));
#47564=CARTESIAN_POINT('',(-6.35355339059327,18.8418830920368,25.2058441227157));
#47565=CARTESIAN_POINT('Origin',(-6.70710678118655,18.3847763108502,26.1629509039023));
#47566=CARTESIAN_POINT('Origin',(-6.25,19.97576656852,24.2184072556393));
#47567=CARTESIAN_POINT('',(-6.14644660940673,18.4276695296637,25.9129509039023));
#47568=CARTESIAN_POINT('',(-6.14644660940673,21.1096500450031,23.2309703885628));
#47569=CARTESIAN_POINT('',(-5.17618446353109,19.7998274154182,25.9129509039023));
#47570=CARTESIAN_POINT('Origin',(-6.5,21.3596500450031,23.4809703885628));
#47571=CARTESIAN_POINT('',(-6.,18.6776695296637,26.1629509039023));
#47572=CARTESIAN_POINT('',(-6.,21.3596500450031,23.4809703885628));
#47573=CARTESIAN_POINT('Origin',(-6.5,18.6776695296637,26.1629509039023));
#47574=CARTESIAN_POINT('Origin',(-6.,24.1123412384613,24.1123412384613));
#47575=CARTESIAN_POINT('',(-6.,22.0617315730203,29.5470129472589));
#47576=CARTESIAN_POINT('',(-6.,26.8650324319194,24.7437120883598));
#47577=CARTESIAN_POINT('',(-6.,20.9177083067616,28.4029896810001));
#47578=CARTESIAN_POINT('Origin',(-6.5,26.8650324319194,24.7437120883598));
#47579=CARTESIAN_POINT('',(-6.14644660940673,22.3117315730203,29.7970129472589));
#47580=CARTESIAN_POINT('',(-6.14644660940673,27.1150324319194,24.9937120883598));
#47581=CARTESIAN_POINT('Origin',(-6.5,22.0617315730203,29.5470129472589));
#47582=CARTESIAN_POINT('Origin',(-6.25,28.2489159084026,24.0062752212833));
#47583=CARTESIAN_POINT('',(-6.35355339059327,22.3117315730203,30.0899061660723));
#47584=CARTESIAN_POINT('',(-6.35355339059327,29.3827993848858,23.0188383542068));
#47585=CARTESIAN_POINT('',(-4.69285113019776,22.3117315730203,27.7413185063573));
#47586=CARTESIAN_POINT('Origin',(-6.70710678118655,29.1327993848858,22.7688383542068));
#47587=CARTESIAN_POINT('',(-6.70710678118655,22.4152849636136,30.1934595566656));
#47588=CARTESIAN_POINT('',(-6.70710678118655,29.486352775479,23.1223917448001));
#47589=CARTESIAN_POINT('Origin',(-6.70710678118655,22.0617315730203,29.8399061660723));
#47590=CARTESIAN_POINT('Origin',(-10.5,28.9913780286485,21.2132034355964));
#47591=CARTESIAN_POINT('',(-10.5,34.2946788875475,25.809397513309));
#47592=CARTESIAN_POINT('',(-10.,33.9411254969543,26.1629509039023));
#47593=CARTESIAN_POINT('Origin',(-10.5,33.9411254969543,26.1629509039023));
#47594=CARTESIAN_POINT('',(-10.,30.1934595566656,22.4152849636136));
#47595=CARTESIAN_POINT('',(-10.,28.9913780286485,21.2132034355964));
#47596=CARTESIAN_POINT('',(-10.5,30.1934595566656,21.708178182427));
#47597=CARTESIAN_POINT('Origin',(-10.5,29.8399061660723,22.0617315730203));
#47598=CARTESIAN_POINT('',(-10.5,29.3449314192417,20.8596500450032));
#47599=CARTESIAN_POINT('Origin',(-14.,33.9411254969543,26.1629509039023));
#47600=CARTESIAN_POINT('',(-14.025428935758,34.2946788875476,26.5165042944955));
#47601=CARTESIAN_POINT('',(-14.,34.4335120598975,26.0760286821578));
#47602=CARTESIAN_POINT('Ctrl Pts',(-14.025428935758,34.2946788875476,26.5165042944955));
#47603=CARTESIAN_POINT('Ctrl Pts',(-14.0263293530702,34.3098071424901,26.501376039553));
#47604=CARTESIAN_POINT('Ctrl Pts',(-14.026804427637,34.3239877839475,26.4852549680463));
#47605=CARTESIAN_POINT('Ctrl Pts',(-14.026804427637,34.3371305955527,26.4682048340719));
#47606=CARTESIAN_POINT('Ctrl Pts',(-14.026804427637,34.3619967163995,26.4359460827032));
#47607=CARTESIAN_POINT('Ctrl Pts',(-14.0250516964297,34.382732239315,26.4009212026149));
#47608=CARTESIAN_POINT('Ctrl Pts',(-14.0179720411043,34.4215374836553,26.3124348467826));
#47609=CARTESIAN_POINT('Ctrl Pts',(-14.0115803121848,34.4352140696344,26.2577402477615));
#47610=CARTESIAN_POINT('Ctrl Pts',(-14.0028573458318,34.4429028780862,26.1599875313316));
#47611=CARTESIAN_POINT('Ctrl Pts',(-14.,34.4408500788191,26.1175962104965));
#47612=CARTESIAN_POINT('Ctrl Pts',(-14.,34.4335120598975,26.0760286821578));
#47613=CARTESIAN_POINT('',(-10.5,34.2946788875475,26.5165042944955));
#47614=CARTESIAN_POINT('',(-14.,34.2946788875475,26.5165042944955));
#47615=CARTESIAN_POINT('Origin',(-10.5,33.9411254969543,26.1629509039023));
#47616=CARTESIAN_POINT('',(-14.,34.2946788875476,25.809397513309));
#47617=CARTESIAN_POINT('',(-14.,34.2946788875476,25.809397513309));
#47618=CARTESIAN_POINT('Origin',(-14.,33.9411254969543,26.1629509039023));
#47619=CARTESIAN_POINT('Origin',(-10.5,33.9411254969543,26.1629509039023));
#47620=CARTESIAN_POINT('Origin',(-10.5,33.9411254969543,26.1629509039023));
#47621=CARTESIAN_POINT('Origin',(-10.,28.2842712474619,28.2842712474619));
#47622=CARTESIAN_POINT('',(-10.,26.1629509039023,33.9411254969543));
#47623=CARTESIAN_POINT('',(-10.,32.1733585439879,27.9307178568686));
#47624=CARTESIAN_POINT('',(-10.,22.4152849636136,30.1934595566656));
#47625=CARTESIAN_POINT('',(-10.,23.4052344572747,31.1834090503267));
#47626=CARTESIAN_POINT('',(-10.,28.4256926036992,24.1830519165799));
#47627=CARTESIAN_POINT('Origin',(-10.5,32.1733585439879,27.9307178568686));
#47628=CARTESIAN_POINT('',(-10.5,26.5165042944955,34.2946788875475));
#47629=CARTESIAN_POINT('',(-10.5,32.5269119345812,28.2842712474619));
#47630=CARTESIAN_POINT('Origin',(-10.5,26.1629509039023,33.9411254969543));
#47631=CARTESIAN_POINT('Origin',(-14.,34.6482322781408,26.1629509039023));
#47632=CARTESIAN_POINT('',(-14.,33.2888210834329,27.5223620986102));
#47633=CARTESIAN_POINT('Ctrl Pts',(-14.025428935758,34.2946788875476,26.5165042944955));
#47634=CARTESIAN_POINT('Ctrl Pts',(-14.0048893955981,33.9495862335655,26.8615969484775));
#47635=CARTESIAN_POINT('Ctrl Pts',(-14.,33.6061320240592,27.2050511579839));
#47636=CARTESIAN_POINT('Ctrl Pts',(-14.,33.2888210834329,27.5223620986102));
#47637=CARTESIAN_POINT('',(-14.,27.5223620986102,33.2888210834329));
#47638=CARTESIAN_POINT('',(-14.,35.5269119345812,25.2842712474619));
#47639=CARTESIAN_POINT('',(-14.025428935758,26.5165042944955,34.2946788875476));
#47640=CARTESIAN_POINT('Ctrl Pts',(-14.,27.5223620986102,33.2888210834329));
#47641=CARTESIAN_POINT('Ctrl Pts',(-14.,27.2050511579839,33.6061320240592));
#47642=CARTESIAN_POINT('Ctrl Pts',(-14.0048893955981,26.8615969484775,33.9495862335655));
#47643=CARTESIAN_POINT('Ctrl Pts',(-14.025428935758,26.5165042944955,34.2946788875476));
#47644=CARTESIAN_POINT('',(-14.,26.5165042944955,34.2946788875475));
#47645=CARTESIAN_POINT('Origin',(-10.5,26.1629509039023,33.9411254969543));
#47646=CARTESIAN_POINT('',(-10.5,25.809397513309,34.2946788875475));
#47647=CARTESIAN_POINT('Origin',(-10.5,26.1629509039023,33.9411254969543));
#47648=CARTESIAN_POINT('Origin',(-10.5,26.1629509039023,33.9411254969543));
#47649=CARTESIAN_POINT('Origin',(-14.,26.1629509039023,17.6776695296637));
#47650=CARTESIAN_POINT('',(-14.,18.2027957955108,9.71751442127219));
#47651=CARTESIAN_POINT('',(-14.,30.1934595566656,21.708178182427));
#47652=CARTESIAN_POINT('Origin',(-14.,26.1629509039023,33.9411254969543));
#47653=CARTESIAN_POINT('',(-14.,26.0760286821578,34.4335120598975));
#47654=CARTESIAN_POINT('Ctrl Pts',(-14.,26.0760286821577,34.4335120598975));
#47655=CARTESIAN_POINT('Ctrl Pts',(-14.,26.110383159214,34.439576740978));
#47656=CARTESIAN_POINT('Ctrl Pts',(-14.0019573651892,26.1453834686123,34.4420465318245));
#47657=CARTESIAN_POINT('Ctrl Pts',(-14.0094015207423,26.2380233090203,34.4388040888907));
#47658=CARTESIAN_POINT('Ctrl Pts',(-14.0161612500453,26.2948454509909,34.4268763441738));
#47659=CARTESIAN_POINT('Ctrl Pts',(-14.0245143380439,26.3913434645052,34.3882911628533));
#47660=CARTESIAN_POINT('Ctrl Pts',(-14.0268044276371,26.4315414345032,34.3653919660536));
#47661=CARTESIAN_POINT('Ctrl Pts',(-14.0268044276371,26.4682048340719,34.3371305955528));
#47662=CARTESIAN_POINT('Ctrl Pts',(-14.0268044276371,26.4852460502184,34.3239946581065));
#47663=CARTESIAN_POINT('Ctrl Pts',(-14.0263298822064,26.501367149334,34.3098160327091));
#47664=CARTESIAN_POINT('Ctrl Pts',(-14.025428935758,26.5165042944956,34.2946788875475));
#47665=CARTESIAN_POINT('',(-14.,25.809397513309,34.2946788875475));
#47666=CARTESIAN_POINT('Origin',(-14.,26.1629509039023,33.9411254969543));
#47667=CARTESIAN_POINT('',(-14.,25.809397513309,34.2946788875475));
#47668=CARTESIAN_POINT('Origin',(-10.5,23.4052344572747,31.1834090503267));
#47669=CARTESIAN_POINT('',(-10.5,21.708178182427,30.1934595566656));
#47670=CARTESIAN_POINT('',(-10.5,23.0516810666815,31.53696244092));
#47671=CARTESIAN_POINT('Origin',(-10.5,22.0617315730203,29.8399061660723));
#47672=CARTESIAN_POINT('Origin',(-5.04640452079103,22.0617315730203,27.4913185063573));
#47673=CARTESIAN_POINT('',(-6.14644660940673,21.8117315730203,29.7970129472589));
#47674=CARTESIAN_POINT('Origin',(-6.5,22.0617315730203,29.5470129472589));
#47675=CARTESIAN_POINT('',(-6.35355339059327,21.8117315730203,30.0899061660723));
#47676=CARTESIAN_POINT('Origin',(-6.70710678118654,22.0617315730203,29.8399061660723));
#47677=CARTESIAN_POINT('',(-4.69285113019776,21.8117315730203,27.7413185063573));
#47678=CARTESIAN_POINT('Origin',(-6.5,20.9177083067616,28.4029896810001));
#47679=CARTESIAN_POINT('',(-6.14644660940673,18.4276695296637,26.4129509039023));
#47680=CARTESIAN_POINT('Origin',(-6.5,18.6776695296637,26.1629509039023));
#47681=CARTESIAN_POINT('Origin',(-6.5,22.0617315730203,29.5470129472589));
#47682=CARTESIAN_POINT('',(-6.14644660940673,20.6677083067616,28.6529896810001));
#47683=CARTESIAN_POINT('Origin',(-6.5,18.6776695296637,26.1629509039023));
#47684=CARTESIAN_POINT('Origin',(-6.5,18.6776695296637,26.1629509039023));
#47685=CARTESIAN_POINT('Origin',(-5.52973785412436,20.0498274154182,26.1629509039023));
#47686=CARTESIAN_POINT('',(-6.35355339059327,18.1347763108502,26.4129509039023));
#47687=CARTESIAN_POINT('Origin',(-6.70710678118654,18.3847763108502,26.1629509039023));
#47688=CARTESIAN_POINT('',(-5.17618446353109,19.7998274154182,26.4129509039023));
#47689=CARTESIAN_POINT('Origin',(-6.5,22.0617315730203,29.5470129472589));
#47690=CARTESIAN_POINT('Origin',(-6.25,21.1424927574778,29.2742207411231));
#47691=CARTESIAN_POINT('',(-6.35355339059327,21.617277208194,29.895451801246));
#47692=CARTESIAN_POINT('Origin',(-14.,30.5470129472589,22.0617315730203));
#47693=CARTESIAN_POINT('',(-14.,30.1934595566656,22.4152849636136));
#47694=CARTESIAN_POINT('',(-14.,22.4152849636136,30.1934595566656));
#47695=CARTESIAN_POINT('Origin',(-14.,29.8399061660723,22.0617315730203));
#47696=CARTESIAN_POINT('Origin',(-14.,22.0617315730203,29.8399061660723));
#47697=CARTESIAN_POINT('',(-6.70710678118655,21.708178182427,30.1934595566656));
#47698=CARTESIAN_POINT('Origin',(-6.70710678118655,22.0617315730203,29.8399061660723));
#47699=CARTESIAN_POINT('',(-14.,21.708178182427,30.1934595566656));
#47700=CARTESIAN_POINT('Origin',(-6.70710678118655,22.0617315730203,29.8399061660723));
#47701=CARTESIAN_POINT('Origin',(-6.70710678118655,22.0617315730203,29.8399061660723));
#47702=CARTESIAN_POINT('Origin',(-6.70710678118655,21.867277208194,29.645451801246));
#47703=CARTESIAN_POINT('',(-6.70710678118655,18.031222920257,26.5165042944955));
#47704=CARTESIAN_POINT('',(-6.70710678118655,21.5137238176007,29.9990051918393));
#47705=CARTESIAN_POINT('Origin',(-6.70710678118655,18.3847763108502,26.1629509039023));
#47706=CARTESIAN_POINT('Origin',(-14.,22.0617315730203,30.5470129472589));
#47707=CARTESIAN_POINT('',(-14.,18.031222920257,26.5165042944955));
#47708=CARTESIAN_POINT('',(-14.,11.9095454429505,20.3948268171891));
#47709=CARTESIAN_POINT('',(-14.,18.031222920257,26.5165042944955));
#47710=CARTESIAN_POINT('Origin',(-6.70710678118655,18.3847763108502,26.1629509039023));
#47711=CARTESIAN_POINT('Origin',(-6.70710678118655,18.3847763108502,26.1629509039023));
#47712=CARTESIAN_POINT('Origin',(-14.,18.3847763108502,26.1629509039023));
#47713=CARTESIAN_POINT('Origin',(-14.,18.3847763108502,26.1629509039023));
#47714=CARTESIAN_POINT('Origin',(-10.5,22.9506403026729,-30.4359216769115));
#47715=CARTESIAN_POINT('',(-10.1464466094067,22.2962265447905,-30.2815079190291));
#47716=CARTESIAN_POINT('',(-10.0449101394378,22.4152849636136,-30.1934595566656));
#47717=CARTESIAN_POINT('Ctrl Pts',(-10.1464466094067,22.2962265447905,-30.2815079190291));
#47718=CARTESIAN_POINT('Ctrl Pts',(-10.1423338164079,22.3000255842635,-30.279490590864));
#47719=CARTESIAN_POINT('Ctrl Pts',(-10.1382848886043,22.3038572286173,-30.2773930503804));
#47720=CARTESIAN_POINT('Ctrl Pts',(-10.1022519938418,22.3387765065044,-30.2576611364803));
#47721=CARTESIAN_POINT('Ctrl Pts',(-10.0750196076115,22.3713854144018,-30.2344766097183));
#47722=CARTESIAN_POINT('Ctrl Pts',(-10.0513757505718,22.4054361818559,-30.2031024097759));
#47723=CARTESIAN_POINT('Ctrl Pts',(-10.0480783085823,22.4103623448515,-30.1983821754277));
#47724=CARTESIAN_POINT('Ctrl Pts',(-10.0449101394378,22.4152849636135,-30.1934595566656));
#47725=CARTESIAN_POINT('',(-10.1464466094067,25.9129509039023,-33.8982322781408));
#47726=CARTESIAN_POINT('',(-10.1464466094067,22.7006403026729,-30.6859216769115));
#47727=CARTESIAN_POINT('',(-10.,26.1629509039022,-33.6482322781408));
#47728=CARTESIAN_POINT('Origin',(-10.5,26.1629509039022,-33.6482322781408));
#47729=CARTESIAN_POINT('',(-10.,22.5617315730203,-30.0470129472589));
#47730=CARTESIAN_POINT('',(-10.,22.9506403026729,-30.4359216769115));
#47731=CARTESIAN_POINT('Origin',(-10.5,22.5617315730203,-30.0470129472589));
#47732=CARTESIAN_POINT('Origin',(-9.05473785412436,26.1629509039023,-31.6043229502591));
#47733=CARTESIAN_POINT('',(-10.4571067811865,26.2923604264535,-34.4240884100988));
#47734=CARTESIAN_POINT('',(-10.3535533905933,26.4129509039023,-34.1911254969543));
#47735=CARTESIAN_POINT('Origin',(-10.7071067811865,26.1629509039023,-33.9411254969543));
#47736=CARTESIAN_POINT('',(-10.1464466094067,26.4129509039023,-33.8982322781408));
#47737=CARTESIAN_POINT('',(-8.70118446353109,26.4129509039023,-31.8543229502591));
#47738=CARTESIAN_POINT('Origin',(-10.5,26.1629509039023,-33.6482322781408));
#47739=CARTESIAN_POINT('',(-10.4829629131445,25.9129509039023,-34.3741381988465));
#47740=CARTESIAN_POINT('',(-8.70118446353109,25.9129509039023,-31.8543229502591));
#47741=CARTESIAN_POINT('Origin',(-10.7071067811865,26.1629509039023,-33.9411254969543));
#47742=CARTESIAN_POINT('Origin',(-10.5,26.1629509039023,-33.6482322781408));
#47743=CARTESIAN_POINT('Origin',(-10.5,26.1629509039022,-33.6482322781408));
#47744=CARTESIAN_POINT('Origin',(-10.,28.2842712474619,-28.2842712474619));
#47745=CARTESIAN_POINT('',(-10.,33.6482322781408,-26.1629509039023));
#47746=CARTESIAN_POINT('',(-10.,28.8449314192417,-30.9662517628014));
#47747=CARTESIAN_POINT('',(-10.,30.0470129472588,-22.5617315730203));
#47748=CARTESIAN_POINT('',(-10.,31.5319371877506,-24.046655813512));
#47749=CARTESIAN_POINT('',(-10.,24.1830519165799,-28.4256926036992));
#47750=CARTESIAN_POINT('Origin',(-10.5,28.8449314192417,-30.9662517628014));
#47751=CARTESIAN_POINT('',(-10.1464466094067,34.0446788875475,-26.2665042944955));
#47752=CARTESIAN_POINT('',(-10.1464466094067,29.0949314192417,-31.2162517628014));
#47753=CARTESIAN_POINT('',(-10.0927098751134,34.0583901847326,-26.1629509039023));
#47754=CARTESIAN_POINT('Origin',(-10.5,33.7946788875475,-26.0165042944955));
#47755=CARTESIAN_POINT('Origin',(-10.5,33.6482322781408,-26.1629509039023));
#47756=CARTESIAN_POINT('Origin',(-10.25,28.1074945521653,-32.3501352392846));
#47757=CARTESIAN_POINT('',(-10.3535533905933,34.1911254969543,-26.4129509039023));
#47758=CARTESIAN_POINT('',(-10.3535533905933,27.1200576850888,-33.4840187157677));
#47759=CARTESIAN_POINT('',(-9.35,33.481506089183,-25.703331496131));
#47760=CARTESIAN_POINT('Origin',(-10.7071067811865,26.8700576850888,-33.2340187157677));
#47761=CARTESIAN_POINT('',(-10.7071067811865,26.5165042944955,-34.2946788875476));
#47762=CARTESIAN_POINT('Origin',(-10.7071067811865,26.1629509039022,-33.9411254969543));
#47763=CARTESIAN_POINT('',(-10.7071067811865,34.2946788875475,-26.5165042944955));
#47764=CARTESIAN_POINT('',(-10.7071067811865,27.2236110756821,-33.587572106361));
#47765=CARTESIAN_POINT('Origin',(-10.7071067811865,33.9411254969543,-26.1629509039023));
#47766=CARTESIAN_POINT('Origin',(-14.,26.1629509039022,-33.9411254969543));
#47767=CARTESIAN_POINT('',(-10.5,25.809397513309,-34.2946788875476));
#47768=CARTESIAN_POINT('Origin',(-10.,26.1629509039022,-33.9411254969543));
#47769=CARTESIAN_POINT('',(-14.,25.809397513309,-34.2946788875476));
#47770=CARTESIAN_POINT('',(-14.,25.809397513309,-34.2946788875476));
#47771=CARTESIAN_POINT('',(-14.,26.5165042944955,-34.2946788875476));
#47772=CARTESIAN_POINT('Origin',(-14.,26.1629509039022,-33.9411254969543));
#47773=CARTESIAN_POINT('',(-14.,26.5165042944955,-34.2946788875476));
#47774=CARTESIAN_POINT('Origin',(-6.70710678118654,25.4558441227157,-19.0918830920368));
#47775=CARTESIAN_POINT('',(-6.35355339059327,25.9129509039023,-18.1347763108502));
#47776=CARTESIAN_POINT('',(-6.70710678118654,25.809397513309,-18.031222920257));
#47777=CARTESIAN_POINT('Origin',(-6.70710678118654,26.1629509039023,-18.3847763108502));
#47778=CARTESIAN_POINT('',(-6.70710678118654,18.031222920257,-25.809397513309));
#47779=CARTESIAN_POINT('',(-6.70710678118654,25.1022907321224,-18.7383297014435));
#47780=CARTESIAN_POINT('',(-6.35355339059327,18.1347763108502,-25.9129509039023));
#47781=CARTESIAN_POINT('Origin',(-6.70710678118654,18.3847763108502,-26.1629509039023));
#47782=CARTESIAN_POINT('',(-6.35355339059327,25.2058441227157,-18.8418830920368));
#47783=CARTESIAN_POINT('Origin',(-6.70710678118655,18.3847763108502,-26.1629509039023));
#47784=CARTESIAN_POINT('',(-6.35355339059327,18.1347763108502,-26.4129509039023));
#47785=CARTESIAN_POINT('',(-6.70710678118654,18.031222920257,-26.5165042944955));
#47786=CARTESIAN_POINT('Origin',(-6.70710678118654,18.3847763108502,-26.1629509039023));
#47787=CARTESIAN_POINT('Origin',(-6.70710678118655,18.3847763108502,-26.1629509039023));
#47788=CARTESIAN_POINT('Origin',(-6.70710678118655,18.3847763108502,-26.1629509039023));
#47789=CARTESIAN_POINT('Origin',(-6.70710678118654,26.1629509039023,-18.3847763108502));
#47790=CARTESIAN_POINT('',(-6.35355339059327,26.4129509039023,-18.1347763108502));
#47791=CARTESIAN_POINT('',(-6.70710678118655,26.5165042944955,-18.031222920257));
#47792=CARTESIAN_POINT('Origin',(-6.70710678118655,26.1629509039023,-18.3847763108502));
#47793=CARTESIAN_POINT('Origin',(-6.70710678118654,26.1629509039023,-18.3847763108502));
#47794=CARTESIAN_POINT('Origin',(-6.70710678118654,26.1629509039023,-18.3847763108502));
#47795=CARTESIAN_POINT('Origin',(-14.,26.1629509039023,-18.3847763108502));
#47796=CARTESIAN_POINT('',(-14.,26.5165042944955,-18.031222920257));
#47797=CARTESIAN_POINT('',(-14.,26.5165042944955,-18.031222920257));
#47798=CARTESIAN_POINT('',(-14.,25.809397513309,-18.031222920257));
#47799=CARTESIAN_POINT('Origin',(-14.,26.1629509039023,-18.3847763108502));
#47800=CARTESIAN_POINT('',(-14.,25.809397513309,-18.031222920257));
#47801=CARTESIAN_POINT('Origin',(-6.70710678118655,29.645451801246,-21.867277208194));
#47802=CARTESIAN_POINT('',(-6.35355339059327,30.0899061660723,-21.8117315730203));
#47803=CARTESIAN_POINT('',(-6.35355339059327,29.895451801246,-21.617277208194));
#47804=CARTESIAN_POINT('',(-6.70710678118655,30.1934595566656,-21.708178182427));
#47805=CARTESIAN_POINT('Origin',(-6.70710678118655,29.8399061660723,-22.0617315730203));
#47806=CARTESIAN_POINT('',(-6.70710678118655,29.9990051918393,-21.5137238176007));
#47807=CARTESIAN_POINT('Origin',(-5.52973785412436,26.1629509039023,-20.0498274154182));
#47808=CARTESIAN_POINT('',(-6.14644660940673,25.9129509039023,-18.4276695296637));
#47809=CARTESIAN_POINT('',(-5.17618446353109,25.9129509039023,-19.7998274154182));
#47810=CARTESIAN_POINT('',(-6.14644660940673,26.4129509039023,-18.4276695296637));
#47811=CARTESIAN_POINT('Origin',(-6.5,26.1629509039023,-18.6776695296637));
#47812=CARTESIAN_POINT('',(-5.17618446353109,26.4129509039023,-19.7998274154182));
#47813=CARTESIAN_POINT('Origin',(-6.25,24.2184072556392,-19.97576656852));
#47814=CARTESIAN_POINT('',(-6.14644660940673,18.4276695296637,-25.9129509039023));
#47815=CARTESIAN_POINT('',(-4.69285113019775,20.4833639705652,-25.9129509039023));
#47816=CARTESIAN_POINT('',(-6.14644660940673,23.2309703885628,-21.1096500450032));
#47817=CARTESIAN_POINT('Origin',(-5.04640452079103,20.7333639705652,-26.1629509039023));
#47818=CARTESIAN_POINT('',(-6.14644660940673,18.4276695296637,-26.4129509039023));
#47819=CARTESIAN_POINT('',(-4.69285113019775,20.4833639705652,-26.4129509039023));
#47820=CARTESIAN_POINT('Origin',(-6.5,18.6776695296637,-26.1629509039023));
#47821=CARTESIAN_POINT('Origin',(-6.5,19.8216927959224,-27.306974170161));
#47822=CARTESIAN_POINT('',(-6.14644660940673,21.8117315730203,-29.7970129472589));
#47823=CARTESIAN_POINT('',(-6.,22.0617315730203,-29.5470129472589));
#47824=CARTESIAN_POINT('Origin',(-6.5,22.0617315730203,-29.5470129472589));
#47825=CARTESIAN_POINT('',(-6.,18.6776695296637,-26.1629509039023));
#47826=CARTESIAN_POINT('',(-6.,19.8216927959224,-27.306974170161));
#47827=CARTESIAN_POINT('Origin',(-6.5,18.6776695296637,-26.1629509039023));
#47828=CARTESIAN_POINT('',(-6.14644660940673,19.5716927959224,-27.556974170161));
#47829=CARTESIAN_POINT('Origin',(-6.5,22.0617315730203,-29.5470129472589));
#47830=CARTESIAN_POINT('',(-6.14644660940673,22.3117315730203,-29.7970129472589));
#47831=CARTESIAN_POINT('Origin',(-6.5,22.0617315730203,-29.5470129472589));
#47832=CARTESIAN_POINT('Origin',(-6.5,22.0617315730203,-29.5470129472589));
#47833=CARTESIAN_POINT('Origin',(-6.5,18.6776695296637,-26.1629509039023));
#47834=CARTESIAN_POINT('Origin',(-6.5,18.6776695296637,-26.1629509039023));
#47835=CARTESIAN_POINT('Origin',(-5.25473785412437,22.0617315730203,-27.7859463318517));
#47836=CARTESIAN_POINT('',(-6.40272606668219,21.8703898568377,-30.2095499766867));
#47837=CARTESIAN_POINT('',(-6.35355339059327,22.3117315730203,-30.0899061660723));
#47838=CARTESIAN_POINT('Origin',(-6.70710678118655,22.0617315730203,-29.8399061660723));
#47839=CARTESIAN_POINT('',(-4.9011844635311,22.3117315730203,-28.0359463318517));
#47840=CARTESIAN_POINT('',(-6.35355339059327,21.8117315730203,-30.0899061660723));
#47841=CARTESIAN_POINT('',(-4.90118446353109,21.8117315730203,-28.0359463318517));
#47842=CARTESIAN_POINT('Origin',(-6.70710678118654,22.0617315730203,-29.8399061660723));
#47843=CARTESIAN_POINT('Origin',(-6.5,23.4809703885628,-21.3596500450032));
#47844=CARTESIAN_POINT('',(-6.,26.1629509039023,-18.6776695296637));
#47845=CARTESIAN_POINT('',(-6.,23.4809703885628,-21.3596500450032));
#47846=CARTESIAN_POINT('Origin',(-6.5,26.1629509039023,-18.6776695296637));
#47847=CARTESIAN_POINT('Origin',(-6.,24.1123412384613,-24.1123412384613));
#47848=CARTESIAN_POINT('',(-6.,29.5470129472589,-22.0617315730203));
#47849=CARTESIAN_POINT('',(-6.,24.7437120883597,-26.8650324319194));
#47850=CARTESIAN_POINT('',(-6.,28.4029896810001,-20.9177083067616));
#47851=CARTESIAN_POINT('Origin',(-6.5,24.7437120883597,-26.8650324319194));
#47852=CARTESIAN_POINT('',(-6.14644660940673,29.7970129472589,-22.3117315730203));
#47853=CARTESIAN_POINT('',(-6.14644660940673,24.9937120883597,-27.1150324319194));
#47854=CARTESIAN_POINT('Origin',(-6.5,29.5470129472589,-22.0617315730203));
#47855=CARTESIAN_POINT('Origin',(-6.25,24.0062752212833,-28.2489159084026));
#47856=CARTESIAN_POINT('',(-6.35355339059327,30.0899061660723,-22.3117315730203));
#47857=CARTESIAN_POINT('',(-6.35355339059327,23.0188383542068,-29.3827993848858));
#47858=CARTESIAN_POINT('',(-4.69285113019775,27.7413185063573,-22.3117315730203));
#47859=CARTESIAN_POINT('Origin',(-6.60355339059327,21.9885082683169,-29.766682861369));
#47860=CARTESIAN_POINT('',(-6.70710678118654,21.708178182427,-30.1934595566656));
#47861=CARTESIAN_POINT('Origin',(-6.70710678118654,22.0617315730203,-29.8399061660723));
#47862=CARTESIAN_POINT('Origin',(-6.70710678118654,22.0617315730203,-29.8399061660723));
#47863=CARTESIAN_POINT('Origin',(-6.70710678118654,18.5792306756765,-26.3574052687286));
#47864=CARTESIAN_POINT('',(-6.70710678118654,18.2256772850833,-26.7109586593218));
#47865=CARTESIAN_POINT('',(-6.35355339059327,18.3292306756765,-26.6074052687286));
#47866=CARTESIAN_POINT('Origin',(-6.25,18.9504617357995,-27.0821897194448));
#47867=CARTESIAN_POINT('Origin',(-14.,18.3847763108502,-26.1629509039023));
#47868=CARTESIAN_POINT('',(-14.,18.031222920257,-25.809397513309));
#47869=CARTESIAN_POINT('',(-14.,18.031222920257,-25.809397513309));
#47870=CARTESIAN_POINT('',(-14.,18.031222920257,-26.5165042944955));
#47871=CARTESIAN_POINT('Origin',(-14.,18.3847763108502,-26.1629509039023));
#47872=CARTESIAN_POINT('',(-14.,18.031222920257,-26.5165042944955));
#47873=CARTESIAN_POINT('Origin',(-14.,26.1629509039023,-17.6776695296637));
#47874=CARTESIAN_POINT('',(-14.,27.0416305603426,-16.7989898732233));
#47875=CARTESIAN_POINT('Origin',(-14.,22.0617315730203,-29.8399061660723));
#47876=CARTESIAN_POINT('',(-6.70710678118654,22.4152849636135,-30.1934595566656));
#47877=CARTESIAN_POINT('Origin',(-6.70710678118654,22.0617315730203,-29.8399061660723));
#47878=CARTESIAN_POINT('',(-10.5,21.708178182427,-30.1934595566656));
#47879=CARTESIAN_POINT('',(-14.,21.708178182427,-30.1934595566656));
#47880=CARTESIAN_POINT('Origin',(-10.,22.0617315730203,-29.8399061660723));
#47881=CARTESIAN_POINT('',(-14.,22.4152849636135,-30.1934595566656));
#47882=CARTESIAN_POINT('Origin',(-6.70710678118654,22.0617315730203,-29.8399061660723));
#47883=CARTESIAN_POINT('Origin',(-6.70710678118654,22.0617315730203,-29.8399061660723));
#47884=CARTESIAN_POINT('Origin',(-6.70710678118654,22.7688383542068,-29.1327993848858));
#47885=CARTESIAN_POINT('',(-6.70710678118654,30.1934595566656,-22.4152849636136));
#47886=CARTESIAN_POINT('',(-6.70710678118654,23.1223917448001,-29.486352775479));
#47887=CARTESIAN_POINT('Origin',(-6.70710678118654,29.8399061660723,-22.0617315730203));
#47888=CARTESIAN_POINT('Origin',(-14.,22.0617315730203,-30.5470129472589));
#47889=CARTESIAN_POINT('',(-10.0449101394378,30.1934595566656,-22.4152849636136));
#47890=CARTESIAN_POINT('Origin',(-10.5,30.0470129472588,-22.5617315730203));
#47891=CARTESIAN_POINT('',(-14.,30.1934595566656,-22.4152849636136));
#47892=CARTESIAN_POINT('Origin',(-14.,17.6776695296637,-26.1629509039023));
#47893=CARTESIAN_POINT('',(-14.,9.7175144212722,-18.2027957955108));
#47894=CARTESIAN_POINT('',(-10.5,20.8596500450031,-29.3449314192417));
#47895=CARTESIAN_POINT('Origin',(-10.25,21.0364267402998,-29.1681547239451));
#47896=CARTESIAN_POINT('Origin',(-10.7071067811865,30.6884343034962,-22.9102597104441));
#47897=CARTESIAN_POINT('',(-10.3535533905933,34.2946788875475,-26.0165042944955));
#47898=CARTESIAN_POINT('',(-10.7071067811865,34.2946788875475,-25.809397513309));
#47899=CARTESIAN_POINT('Origin',(-10.7071067811865,33.9411254969543,-26.1629509039023));
#47900=CARTESIAN_POINT('',(-10.7071067811865,30.1934595566656,-21.708178182427));
#47901=CARTESIAN_POINT('',(-10.7071067811865,31.0419876940894,-22.5567063198509));
#47902=CARTESIAN_POINT('',(-10.3535533905933,30.3399061660723,-22.0617315730203));
#47903=CARTESIAN_POINT('Origin',(-10.7071067811865,29.8399061660723,-22.0617315730203));
#47904=CARTESIAN_POINT('',(-10.3535533905933,30.9384343034962,-22.6602597104441));
#47905=CARTESIAN_POINT('Origin',(-14.,30.5470129472588,-22.0617315730203));
#47906=CARTESIAN_POINT('',(-14.,30.1934595566656,-21.708178182427));
#47907=CARTESIAN_POINT('',(-14.,34.2946788875475,-25.809397513309));
#47908=CARTESIAN_POINT('',(-14.,34.2946788875475,-25.809397513309));
#47909=CARTESIAN_POINT('',(-14.,20.3948268171891,-11.9095454429505));
#47910=CARTESIAN_POINT('Origin',(-9.70355339059327,33.231506089183,-25.453331496131));
#47911=CARTESIAN_POINT('',(-10.1464466094067,34.1263048569333,-26.1410234826947));
#47912=CARTESIAN_POINT('Origin',(-10.,33.4411254969543,-25.6629509039023));
#47913=CARTESIAN_POINT('Ctrl Pts',(-10.1464466094067,34.1263048569333,-26.1410234826947));
#47914=CARTESIAN_POINT('Ctrl Pts',(-10.1267754433189,34.1045114392619,-26.1470492948923));
#47915=CARTESIAN_POINT('Ctrl Pts',(-10.1087254771823,34.0818363093199,-26.1545897832218));
#47916=CARTESIAN_POINT('Ctrl Pts',(-10.0927098751134,34.0583901847326,-26.1629509039023));
#47917=CARTESIAN_POINT('Origin',(-10.7071067811865,33.9411254969543,-26.1629509039023));
#47918=CARTESIAN_POINT('Origin',(-10.7071067811865,33.9411254969543,-26.1629509039023));
#47919=CARTESIAN_POINT('Origin',(-10.7071067811865,33.9411254969543,-26.1629509039023));
#47920=CARTESIAN_POINT('Origin',(-10.5,31.5319371877506,-24.046655813512));
#47921=CARTESIAN_POINT('',(-10.1464466094067,30.2815079190291,-22.2962265447905));
#47922=CARTESIAN_POINT('',(-10.1464466094067,31.7819371877506,-23.796655813512));
#47923=CARTESIAN_POINT('Ctrl Pts',(-10.0449101394378,30.1934595566656,-22.4152849636136));
#47924=CARTESIAN_POINT('Ctrl Pts',(-10.0480783085823,30.1983821754277,-22.4103623448515));
#47925=CARTESIAN_POINT('Ctrl Pts',(-10.0513757505718,30.2031024097759,-22.4054361818559));
#47926=CARTESIAN_POINT('Ctrl Pts',(-10.0750196076115,30.2344766097183,-22.3713854144018));
#47927=CARTESIAN_POINT('Ctrl Pts',(-10.1022519938418,30.2576611364803,-22.3387765065044));
#47928=CARTESIAN_POINT('Ctrl Pts',(-10.1382848886043,30.2773930503804,-22.3038572286173));
#47929=CARTESIAN_POINT('Ctrl Pts',(-10.142333816408,30.279490590864,-22.3000255842635));
#47930=CARTESIAN_POINT('Ctrl Pts',(-10.1464466094067,30.2815079190291,-22.2962265447905));
#47931=CARTESIAN_POINT('Origin',(-6.5,26.1629509039023,-18.6776695296637));
#47932=CARTESIAN_POINT('Origin',(-6.5,26.1629509039023,-18.6776695296637));
#47933=CARTESIAN_POINT('Origin',(-14.,33.9411254969543,-26.1629509039023));
#47934=CARTESIAN_POINT('',(-14.025428935758,34.2946788875476,-26.5165042944955));
#47935=CARTESIAN_POINT('',(-14.,34.2946788875475,-26.5165042944955));
#47936=CARTESIAN_POINT('',(-14.,34.4335120598975,-26.0760286821578));
#47937=CARTESIAN_POINT('Ctrl Pts',(-14.,34.4335120598975,-26.0760286821577));
#47938=CARTESIAN_POINT('Ctrl Pts',(-14.,34.439576740978,-26.110383159214));
#47939=CARTESIAN_POINT('Ctrl Pts',(-14.0019573651892,34.4420465318245,-26.1453834686123));
#47940=CARTESIAN_POINT('Ctrl Pts',(-14.0094015207423,34.4388040888907,-26.2380233090204));
#47941=CARTESIAN_POINT('Ctrl Pts',(-14.0161612500454,34.4268763441737,-26.294845450991));
#47942=CARTESIAN_POINT('Ctrl Pts',(-14.0245143380439,34.3882911628533,-26.3913434645052));
#47943=CARTESIAN_POINT('Ctrl Pts',(-14.026804427637,34.3653919660536,-26.4315414345033));
#47944=CARTESIAN_POINT('Ctrl Pts',(-14.026804427637,34.3371305955527,-26.4682048340719));
#47945=CARTESIAN_POINT('Ctrl Pts',(-14.026804427637,34.3239946581065,-26.4852460502184));
#47946=CARTESIAN_POINT('Ctrl Pts',(-14.0263298822064,34.3098160327091,-26.501367149334));
#47947=CARTESIAN_POINT('Ctrl Pts',(-14.025428935758,34.2946788875475,-26.5165042944956));
#47948=CARTESIAN_POINT('Origin',(-14.,33.9411254969543,-26.1629509039023));
#47949=CARTESIAN_POINT('Origin',(-10.25,31.3601857456234,-23.2284577619781));
#47950=CARTESIAN_POINT('Origin',(-10.,29.8399061660723,-22.0617315730203));
#47951=CARTESIAN_POINT('Origin',(-5.04640452079103,27.4913185063573,-22.0617315730203));
#47952=CARTESIAN_POINT('',(-6.14644660940673,29.7970129472589,-21.8117315730203));
#47953=CARTESIAN_POINT('Origin',(-6.5,29.5470129472589,-22.0617315730203));
#47954=CARTESIAN_POINT('Origin',(-6.70710678118654,29.8399061660723,-22.0617315730203));
#47955=CARTESIAN_POINT('',(-4.69285113019775,27.7413185063573,-21.8117315730203));
#47956=CARTESIAN_POINT('Origin',(-6.70710678118654,29.8399061660723,-22.0617315730203));
#47957=CARTESIAN_POINT('Origin',(-6.70710678118654,29.8399061660723,-22.0617315730203));
#47958=CARTESIAN_POINT('Origin',(-14.,29.8399061660723,-22.0617315730203));
#47959=CARTESIAN_POINT('Origin',(-6.5,28.4029896810001,-20.9177083067616));
#47960=CARTESIAN_POINT('Origin',(-6.5,29.5470129472589,-22.0617315730203));
#47961=CARTESIAN_POINT('',(-6.14644660940673,28.6529896810001,-20.6677083067616));
#47962=CARTESIAN_POINT('Origin',(-6.5,29.5470129472589,-22.0617315730203));
#47963=CARTESIAN_POINT('Origin',(-6.25,29.2742207411231,-21.1424927574778));
#47964=CARTESIAN_POINT('Origin',(-76.,0.,0.));
#47965=CARTESIAN_POINT('',(-76.,-44.,-5.38844591624836E-15));
#47966=CARTESIAN_POINT('',(-76.,-5.38844591624836E-15,-44.));
#47967=CARTESIAN_POINT('Origin',(-76.,0.,0.));
#47968=CARTESIAN_POINT('',(-75.5,-5.32721357629099E-15,-43.5));
#47969=CARTESIAN_POINT('Origin',(-76.,-5.32721357629099E-15,-43.5));
#47970=CARTESIAN_POINT('Origin',(-75.5,0.,0.));
#47971=CARTESIAN_POINT('Origin',(-76.,0.,0.));
#47972=CARTESIAN_POINT('Origin',(-75.,0.,0.));
#47973=CARTESIAN_POINT('',(-81.9928932188135,-44.,-5.38844591624836E-15));
#47974=CARTESIAN_POINT('',(-75.,-44.,-5.38844591624836E-15));
#47975=CARTESIAN_POINT('',(-81.9928932188135,-28.792835000627,-33.2711985450881));
#47976=CARTESIAN_POINT('Origin',(-81.9928932188135,0.,0.));
#47977=CARTESIAN_POINT('',(-76.5,-28.7928350006269,-33.2711985450881));
#47978=CARTESIAN_POINT('',(-75.,-28.7928350006269,-33.2711985450881));
#47979=CARTESIAN_POINT('',(-76.5,-17.7850525803124,-40.2453960685632));
#47980=CARTESIAN_POINT('Origin',(-76.5,0.,0.));
#47981=CARTESIAN_POINT('',(-81.9928932188135,-17.7850525803124,-40.2453960685632));
#47982=CARTESIAN_POINT('',(-75.,-17.7850525803124,-40.2453960685632));
#47983=CARTESIAN_POINT('',(-81.9928932188135,33.2711985450881,-28.792835000627));
#47984=CARTESIAN_POINT('Origin',(-81.9928932188135,0.,0.));
#47985=CARTESIAN_POINT('',(-76.5,33.2711985450881,-28.792835000627));
#47986=CARTESIAN_POINT('',(-75.,33.2711985450881,-28.792835000627));
#47987=CARTESIAN_POINT('',(-76.5,40.2453960685632,-17.7850525803124));
#47988=CARTESIAN_POINT('Origin',(-76.5,0.,0.));
#47989=CARTESIAN_POINT('',(-81.9928932188135,40.2453960685632,-17.7850525803124));
#47990=CARTESIAN_POINT('',(-75.,40.2453960685632,-17.7850525803124));
#47991=CARTESIAN_POINT('',(-81.9928932188135,28.7928350006269,33.2711985450881));
#47992=CARTESIAN_POINT('Origin',(-81.9928932188135,0.,0.));
#47993=CARTESIAN_POINT('',(-76.5,28.7928350006269,33.2711985450881));
#47994=CARTESIAN_POINT('',(-75.,28.7928350006269,33.2711985450881));
#47995=CARTESIAN_POINT('',(-76.5,17.7850525803124,40.2453960685632));
#47996=CARTESIAN_POINT('Origin',(-76.5,0.,0.));
#47997=CARTESIAN_POINT('',(-81.9928932188135,17.7850525803124,40.2453960685632));
#47998=CARTESIAN_POINT('',(-75.,17.7850525803124,40.2453960685632));
#47999=CARTESIAN_POINT('',(-81.9928932188135,-33.2711985450881,28.7928350006269));
#48000=CARTESIAN_POINT('Origin',(-81.9928932188135,0.,0.));
#48001=CARTESIAN_POINT('',(-76.5,-33.2711985450881,28.7928350006269));
#48002=CARTESIAN_POINT('',(-75.,-33.2711985450881,28.7928350006269));
#48003=CARTESIAN_POINT('',(-76.5,-40.2453960685632,17.7850525803123));
#48004=CARTESIAN_POINT('Origin',(-76.5,0.,0.));
#48005=CARTESIAN_POINT('',(-81.9928932188135,-40.2453960685632,17.7850525803123));
#48006=CARTESIAN_POINT('',(-75.,-40.2453960685632,17.7850525803123));
#48007=CARTESIAN_POINT('Origin',(-81.9928932188135,0.,0.));
#48008=CARTESIAN_POINT('Origin',(-75.5,44.5,0.));
#48009=CARTESIAN_POINT('',(-75.5,-42.4,-5.19250242838478E-15));
#48010=CARTESIAN_POINT('Origin',(-75.5,0.,0.));
#48011=CARTESIAN_POINT('Origin',(-82.5,27.2681929349507,18.7607836329628));
#48012=CARTESIAN_POINT('',(-82.8535533905933,18.1725024134732,39.3532030423759));
#48013=CARTESIAN_POINT('',(-82.5,18.1497255644298,39.7527038317633));
#48014=CARTESIAN_POINT('Ctrl Pts',(-82.8535533905933,18.1725024134732,39.3532030423759));
#48015=CARTESIAN_POINT('Ctrl Pts',(-82.8366099658527,18.1852779971399,39.3659662456744));
#48016=CARTESIAN_POINT('Ctrl Pts',(-82.8190446071419,18.1949775258609,39.3808339631167));
#48017=CARTESIAN_POINT('Ctrl Pts',(-82.7677366682921,18.2164972638614,39.4274108400557));
#48018=CARTESIAN_POINT('Ctrl Pts',(-82.7337459048348,18.2211084931905,39.4627255203892));
#48019=CARTESIAN_POINT('Ctrl Pts',(-82.6671016739128,18.2188694611548,39.5371512535174));
#48020=CARTESIAN_POINT('Ctrl Pts',(-82.6344780878158,18.211893370137,39.5762852200451));
#48021=CARTESIAN_POINT('Ctrl Pts',(-82.5669046106341,18.1882818091273,39.661496926548));
#48022=CARTESIAN_POINT('Ctrl Pts',(-82.5323527761039,18.1704694163667,39.7076676112556));
#48023=CARTESIAN_POINT('Ctrl Pts',(-82.5,18.1497255644298,39.7527038317633));
#48024=CARTESIAN_POINT('',(-82.5,24.4987646471392,25.9685365994627));
#48025=CARTESIAN_POINT('',(-82.5,27.7223340063745,18.9699627123327));
#48026=CARTESIAN_POINT('',(-83.,24.0446235757154,25.7593575200928));
#48027=CARTESIAN_POINT('Origin',(-82.5,24.0446235757154,25.7593575200928));
#48028=CARTESIAN_POINT('',(-83.,17.9060450480377,39.0866015158896));
#48029=CARTESIAN_POINT('',(-83.,27.2681929349507,18.7607836329628));
#48030=CARTESIAN_POINT('Ctrl Pts',(-83.,17.9060450480377,39.0866015158896));
#48031=CARTESIAN_POINT('Ctrl Pts',(-83.,17.9068391651052,39.0873972685336));
#48032=CARTESIAN_POINT('Ctrl Pts',(-82.9999966660379,17.9076332865639,39.0881930147409));
#48033=CARTESIAN_POINT('Ctrl Pts',(-82.9996048777198,17.9542929979794,39.1349475530888));
#48034=CARTESIAN_POINT('Ctrl Pts',(-82.9880998337802,17.9999192181754,39.1806291884362));
#48035=CARTESIAN_POINT('Ctrl Pts',(-82.9422519329555,18.0884603751996,39.2692142985112));
#48036=CARTESIAN_POINT('Ctrl Pts',(-82.9069781960815,18.1305308491385,39.3112695307757));
#48037=CARTESIAN_POINT('Ctrl Pts',(-82.8587400616057,18.1685480689101,39.3492524644103));
#48038=CARTESIAN_POINT('Ctrl Pts',(-82.8561621144247,18.1705353985348,39.3512379336024));
#48039=CARTESIAN_POINT('Ctrl Pts',(-82.8535533905933,18.1725024134732,39.3532030423759));
#48040=CARTESIAN_POINT('Origin',(-82.5,27.2236110756821,27.2236110756821));
#48041=CARTESIAN_POINT('',(-82.5,29.9484575042249,28.4786855519015));
#48042=CARTESIAN_POINT('',(-83.,30.4025985756487,28.6878646312713));
#48043=CARTESIAN_POINT('Origin',(-82.5,30.4025985756487,28.6878646312713));
#48044=CARTESIAN_POINT('Origin',(-83.,27.2236110756821,27.2236110756821));
#48045=CARTESIAN_POINT('Origin',(-82.5,27.2236110756821,27.2236110756821));
#48046=CARTESIAN_POINT('Origin',(-82.5,36.9730332048023,14.4230336013604));
#48047=CARTESIAN_POINT('',(-82.5,28.5407738489008,31.5348562042458));
#48048=CARTESIAN_POINT('',(-83.,28.9949149203246,31.7440352836156));
#48049=CARTESIAN_POINT('Origin',(-82.5,28.9949149203246,31.7440352836156));
#48050=CARTESIAN_POINT('',(-83.,36.9730332048023,14.4230336013604));
#48051=CARTESIAN_POINT('',(-82.5,36.5188921333785,14.2138545219905));
#48052=CARTESIAN_POINT('Origin',(-82.5,28.9949149203246,31.7440352836156));
#48053=CARTESIAN_POINT('',(-82.8535533905933,29.2333555023034,32.0050833421521));
#48054=CARTESIAN_POINT('Origin',(-82.5,28.9949149203246,31.7440352836156));
#48055=CARTESIAN_POINT('Origin',(-82.5,28.9949149203246,31.7440352836156));
#48056=CARTESIAN_POINT('Origin',(-81.9928932188135,28.4656436938016,32.8931167434394));
#48057=CARTESIAN_POINT('',(-82.3464466094067,28.6970028856031,33.1604609492284));
#48058=CARTESIAN_POINT('',(-81.9928932188135,28.0115026223778,32.6839376640695));
#48059=CARTESIAN_POINT('Origin',(-81.9928932188135,28.4656436938016,32.8931167434394));
#48060=CARTESIAN_POINT('',(-81.9928932188135,27.9656436938016,32.8931167434394));
#48061=CARTESIAN_POINT('Origin',(-81.9928932188135,28.4656436938016,32.8931167434394));
#48062=CARTESIAN_POINT('',(-82.0504431038337,27.9740691453425,32.9641271232539));
#48063=CARTESIAN_POINT('Origin',(-81.9928932188135,28.4656436938016,32.8931167434394));
#48064=CARTESIAN_POINT('Origin',(-81.9928932188135,28.4656436938016,32.8931167434394));
#48065=CARTESIAN_POINT('Origin',(-81.9928932188135,28.4656436938016,32.8931167434394));
#48066=CARTESIAN_POINT('Ctrl Pts',(-82.3464466094067,28.6970028856031,33.1604609492284));
#48067=CARTESIAN_POINT('Ctrl Pts',(-82.5198916952181,28.8750299889571,32.777021537783));
#48068=CARTESIAN_POINT('Ctrl Pts',(-82.6890302423685,29.0538136387275,32.3919001753921));
#48069=CARTESIAN_POINT('Ctrl Pts',(-82.8535533905932,29.2333555023034,32.0050833421521));
#48070=CARTESIAN_POINT('Ctrl Pts',(-82.4107979354011,28.6107539071896,33.1499982741659));
#48071=CARTESIAN_POINT('Ctrl Pts',(-82.5847771257014,28.7890085398853,32.7663377509294));
#48072=CARTESIAN_POINT('Ctrl Pts',(-82.7544490809092,28.9680220426012,32.3809740568209));
#48073=CARTESIAN_POINT('Ctrl Pts',(-82.9195064441822,29.1478143532338,31.9938921294479));
#48074=CARTESIAN_POINT('Ctrl Pts',(-82.4878723202377,28.4047764122382,33.0901740387693));
#48075=CARTESIAN_POINT('Ctrl Pts',(-82.6627581651749,28.583033090945,32.7062483470394));
#48076=CARTESIAN_POINT('Ctrl Pts',(-82.8333405871198,28.7620735816751,32.3205905916121));
#48077=CARTESIAN_POINT('Ctrl Pts',(-82.9993073418929,28.9419061790346,31.9331823972077));
#48078=CARTESIAN_POINT('Ctrl Pts',(-82.402697304057,28.1204642389912,32.9204852331458));
#48079=CARTESIAN_POINT('Ctrl Pts',(-82.5777878858747,28.2977526404933,32.536956679965));
#48080=CARTESIAN_POINT('Ctrl Pts',(-82.7485753212377,28.4758222195063,32.1517086466974));
#48081=CARTESIAN_POINT('Ctrl Pts',(-82.9147495721166,28.6546921362081,31.764723584709));
#48082=CARTESIAN_POINT('Ctrl Pts',(-82.1928732504717,28.0005687726945,32.769842915114));
#48083=CARTESIAN_POINT('Ctrl Pts',(-82.3671797925051,28.17683463364,32.3873378092548));
#48084=CARTESIAN_POINT('Ctrl Pts',(-82.537183228921,28.3538706019485,32.0031656241164));
#48085=CARTESIAN_POINT('Ctrl Pts',(-82.7025711378507,28.5316782401504,31.6173102173229));
#48086=CARTESIAN_POINT('Ctrl Pts',(-82.0428577478797,28.002868743917,32.702682362758));
#48087=CARTESIAN_POINT('Ctrl Pts',(-82.2165175283878,28.178677124377,32.3209949026089));
#48088=CARTESIAN_POINT('Ctrl Pts',(-82.3858725432196,28.355232305031,31.9376749996291));
#48089=CARTESIAN_POINT('Ctrl Pts',(-82.5506111984385,28.5325481277584,31.5527147674639));
#48090=CARTESIAN_POINT('Ctrl Pts',(-81.9928932188135,28.0115026223778,32.6839376640695));
#48091=CARTESIAN_POINT('Ctrl Pts',(-82.1663383046248,28.1871793984968,32.3025322215592));
#48092=CARTESIAN_POINT('Ctrl Pts',(-82.3354768517752,28.3636014212964,31.9195088011564));
#48093=CARTESIAN_POINT('Ctrl Pts',(-82.5,28.5407738489008,31.5348562042457));
#48094=CARTESIAN_POINT('Ctrl Pts',(-82.3464466094067,28.6970028856031,33.1604609492284));
#48095=CARTESIAN_POINT('Ctrl Pts',(-82.5198916952181,28.8750299889571,32.777021537783));
#48096=CARTESIAN_POINT('Ctrl Pts',(-82.6890302423685,29.0538136387275,32.3919001753921));
#48097=CARTESIAN_POINT('Ctrl Pts',(-82.8535533905932,29.2333555023034,32.0050833421521));
#48098=CARTESIAN_POINT('Ctrl Pts',(-82.5,28.5407738489008,31.5348562042457));
#48099=CARTESIAN_POINT('Ctrl Pts',(-82.3354768517752,28.3636014212964,31.9195088011564));
#48100=CARTESIAN_POINT('Ctrl Pts',(-82.1663383046248,28.1871793984968,32.3025322215592));
#48101=CARTESIAN_POINT('Ctrl Pts',(-81.9928932188135,28.0115026223778,32.6839376640695));
#48102=CARTESIAN_POINT('Origin',(-83.,43.2,0.));
#48103=CARTESIAN_POINT('',(-83.,39.0866015158896,-17.9060450480377));
#48104=CARTESIAN_POINT('Origin',(-83.,0.,0.));
#48105=CARTESIAN_POINT('',(-83.,25.7593575200928,-24.0446235757154));
#48106=CARTESIAN_POINT('',(-83.,44.7879994647011,-15.2799597870972));
#48107=CARTESIAN_POINT('',(-83.,28.6878646312713,-30.4025985756487));
#48108=CARTESIAN_POINT('Origin',(-83.,27.2236110756821,-27.2236110756821));
#48109=CARTESIAN_POINT('',(-83.,31.7440352836156,-28.9949149203246));
#48110=CARTESIAN_POINT('',(-83.,40.4502494330987,-24.9848000569488));
#48111=CARTESIAN_POINT('',(-83.,-17.9060450480377,-39.0866015158896));
#48112=CARTESIAN_POINT('Origin',(-83.,0.,0.));
#48113=CARTESIAN_POINT('',(-83.,-24.0446235757154,-25.7593575200928));
#48114=CARTESIAN_POINT('',(-83.,-19.7071756188355,-35.1762326125546));
#48115=CARTESIAN_POINT('',(-83.,-30.4025985756487,-28.6878646312713));
#48116=CARTESIAN_POINT('Origin',(-83.,-27.2236110756821,-27.2236110756821));
#48117=CARTESIAN_POINT('',(-83.,-28.9949149203246,-31.7440352836156));
#48118=CARTESIAN_POINT('',(-83.,-29.4120158886871,-30.8384825809522));
#48119=CARTESIAN_POINT('',(-83.,-39.0866015158896,17.9060450480377));
#48120=CARTESIAN_POINT('Origin',(-83.,0.,0.));
#48121=CARTESIAN_POINT('',(-83.,-25.7593575200928,24.0446235757154));
#48122=CARTESIAN_POINT('',(-83.,-9.14901678081629,31.695408766689));
#48123=CARTESIAN_POINT('',(-83.,-28.6878646312713,30.4025985756487));
#48124=CARTESIAN_POINT('Origin',(-83.,-27.2236110756821,27.2236110756821));
#48125=CARTESIAN_POINT('',(-83.,-31.7440352836156,28.9949149203246));
#48126=CARTESIAN_POINT('',(-83.,-4.81126674921393,41.4002490365406));
#48127=CARTESIAN_POINT('Origin',(-83.,0.,0.));
#48128=CARTESIAN_POINT('',(-83.,-9.49971599022433E-16,-7.75710678118654));
#48129=CARTESIAN_POINT('Origin',(-83.,0.,0.));
#48130=CARTESIAN_POINT('Origin',(-82.5,0.,0.));
#48131=CARTESIAN_POINT('',(-82.8535533905933,39.4080313955299,-18.0532959647562));
#48132=CARTESIAN_POINT('Origin',(-82.8535533905933,4.44089209850063E-15,
-2.77555756156289E-15));
#48133=CARTESIAN_POINT('Origin',(-82.5,39.0866015158896,-17.9060450480377));
#48134=CARTESIAN_POINT('Origin',(-82.6,0.,0.));
#48135=CARTESIAN_POINT('',(-82.3464466129164,40.1114460228581,-17.7258580223676));
#48136=CARTESIAN_POINT('Origin',(-82.3464466094067,0.,-3.33066907387547E-15));
#48137=CARTESIAN_POINT('Ctrl Pts',(-82.8535533905933,39.4080313955299,-18.0532959647562));
#48138=CARTESIAN_POINT('Ctrl Pts',(-82.6854396980163,39.6430704046442,-17.9438814038579));
#48139=CARTESIAN_POINT('Ctrl Pts',(-82.5163877136628,39.8775346219,-17.8347386981006));
#48140=CARTESIAN_POINT('Ctrl Pts',(-82.3464466129164,40.1114460228581,-17.7258580223676));
#48141=CARTESIAN_POINT('Origin',(-81.9928932188135,0.,0.));
#48142=CARTESIAN_POINT('Origin',(-81.9928932188135,39.7880620223296,-17.5829497100815));
#48143=CARTESIAN_POINT('Origin',(-75.,28.4656436938016,32.8931167434394));
#48144=CARTESIAN_POINT('',(-77.,28.0115026223778,32.6839376640695));
#48145=CARTESIAN_POINT('',(-75.,28.0115026223778,32.6839376640695));
#48146=CARTESIAN_POINT('',(-77.,28.0856877263144,33.2181297628261));
#48147=CARTESIAN_POINT('Origin',(-77.,28.4656436938016,32.8931167434394));
#48148=CARTESIAN_POINT('Ctrl Pts',(-76.5,28.7928350006269,33.2711985450881));
#48149=CARTESIAN_POINT('Ctrl Pts',(-76.5009112946168,28.7921419638462,33.2717982978638));
#48150=CARTESIAN_POINT('Ctrl Pts',(-76.501822590879,28.7914472767631,33.2723961461826));
#48151=CARTESIAN_POINT('Ctrl Pts',(-76.5561204584075,28.749957410408,33.3079042591946));
#48152=CARTESIAN_POINT('Ctrl Pts',(-76.6098195625403,28.7032660033557,33.3364800964725));
#48153=CARTESIAN_POINT('Ctrl Pts',(-76.7122026008175,28.602334790547,33.3770567140054));
#48154=CARTESIAN_POINT('Ctrl Pts',(-76.7616726361357,28.5476297045157,33.3897295300249));
#48155=CARTESIAN_POINT('Ctrl Pts',(-76.850087254088,28.4352133445064,33.3951790166874));
#48156=CARTESIAN_POINT('Ctrl Pts',(-76.889996425565,28.3771217427946,33.3890059164672));
#48157=CARTESIAN_POINT('Ctrl Pts',(-76.9474081328341,28.27413553634,33.3573297979247));
#48158=CARTESIAN_POINT('Ctrl Pts',(-76.9678406878702,28.2296235623677,33.3368297278635));
#48159=CARTESIAN_POINT('Ctrl Pts',(-76.9935652964058,28.1501559864102,33.2835955472113));
#48160=CARTESIAN_POINT('Ctrl Pts',(-77.,28.1158074516949,33.253341181184));
#48161=CARTESIAN_POINT('Ctrl Pts',(-77.,28.0856877263144,33.2181297628261));
#48162=CARTESIAN_POINT('Origin',(-82.5,-9.14901678081629,31.695408766689));
#48163=CARTESIAN_POINT('',(-82.8535533905933,-39.3532030423759,18.1725024134732));
#48164=CARTESIAN_POINT('',(-82.5,-39.7527038317633,18.1497255644298));
#48165=CARTESIAN_POINT('Ctrl Pts',(-82.8535533905933,-39.3532030423759,
18.1725024134732));
#48166=CARTESIAN_POINT('Ctrl Pts',(-82.8366099658527,-39.3659662456744,
18.1852779971399));
#48167=CARTESIAN_POINT('Ctrl Pts',(-82.8190446071419,-39.3808339631167,
18.1949775258609));
#48168=CARTESIAN_POINT('Ctrl Pts',(-82.7677366682921,-39.4274108400557,
18.2164972638614));
#48169=CARTESIAN_POINT('Ctrl Pts',(-82.7337459048348,-39.4627255203892,
18.2211084931905));
#48170=CARTESIAN_POINT('Ctrl Pts',(-82.6671016739128,-39.5371512535175,
18.2188694611548));
#48171=CARTESIAN_POINT('Ctrl Pts',(-82.6344780878157,-39.5762852200451,
18.211893370137));
#48172=CARTESIAN_POINT('Ctrl Pts',(-82.5669046106341,-39.661496926548,18.1882818091273));
#48173=CARTESIAN_POINT('Ctrl Pts',(-82.5323527761039,-39.7076676112556,
18.1704694163667));
#48174=CARTESIAN_POINT('Ctrl Pts',(-82.5,-39.7527038317633,18.1497255644297));
#48175=CARTESIAN_POINT('',(-82.5,-25.9685365994627,24.4987646471392));
#48176=CARTESIAN_POINT('',(-82.5,-9.35819586018618,32.1495498381128));
#48177=CARTESIAN_POINT('Origin',(-82.5,-25.7593575200928,24.0446235757154));
#48178=CARTESIAN_POINT('Ctrl Pts',(-83.,-39.0866015158896,17.9060450480377));
#48179=CARTESIAN_POINT('Ctrl Pts',(-83.,-39.0873972740994,17.9068391706596));
#48180=CARTESIAN_POINT('Ctrl Pts',(-82.9999966659913,-39.0881930258708,
17.9076332976816));
#48181=CARTESIAN_POINT('Ctrl Pts',(-82.9996059304676,-39.1348216015621,
17.9541673017709));
#48182=CARTESIAN_POINT('Ctrl Pts',(-82.9881628075444,-39.1803794345047,
17.9996697609635));
#48183=CARTESIAN_POINT('Ctrl Pts',(-82.9424916603154,-39.2688855146336,
18.0881315731075));
#48184=CARTESIAN_POINT('Ctrl Pts',(-82.9072680988186,-39.3109720341272,
18.130233190386));
#48185=CARTESIAN_POINT('Ctrl Pts',(-82.8589631266987,-39.3490805827825,
18.1683760263469));
#48186=CARTESIAN_POINT('Ctrl Pts',(-82.8562750094044,-39.3511528916702,
18.1704502741115));
#48187=CARTESIAN_POINT('Ctrl Pts',(-82.8535533905933,-39.3532030423759,
18.1725024134732));
#48188=CARTESIAN_POINT('Origin',(-82.5,-27.2236110756821,27.2236110756821));
#48189=CARTESIAN_POINT('',(-82.5,-28.4786855519014,29.9484575042249));
#48190=CARTESIAN_POINT('Origin',(-82.5,-28.6878646312713,30.4025985756487));
#48191=CARTESIAN_POINT('Origin',(-82.5,-27.2236110756821,27.2236110756821));
#48192=CARTESIAN_POINT('Origin',(-82.5,-4.81126674921393,41.4002490365406));
#48193=CARTESIAN_POINT('',(-82.861919052854,-33.0775140978602,28.0008882573809));
#48194=CARTESIAN_POINT('Ctrl Pts',(-82.861919052854,-33.0775140978601,28.0008882573809));
#48195=CARTESIAN_POINT('Ctrl Pts',(-82.9506866114062,-32.7352615883927,
28.2610595985261));
#48196=CARTESIAN_POINT('Ctrl Pts',(-82.9991927191309,-32.2707133550685,
28.6098467819186));
#48197=CARTESIAN_POINT('Ctrl Pts',(-82.9999966796634,-31.7526069532298,
28.9886497095682));
#48198=CARTESIAN_POINT('Ctrl Pts',(-83.,-31.7483212454185,28.991782520556));
#48199=CARTESIAN_POINT('Ctrl Pts',(-83.,-31.7440352836157,28.9949149203247));
#48200=CARTESIAN_POINT('',(-82.5,-32.6839376640695,28.0115026223778));
#48201=CARTESIAN_POINT('',(-82.5,-4.60208766984403,40.9461079651168));
#48202=CARTESIAN_POINT('Origin',(-82.5,-32.8931167434394,28.4656436938016));
#48203=CARTESIAN_POINT('Origin',(-82.5,0.,0.));
#48204=CARTESIAN_POINT('',(-82.8535533905933,-29.2333555023034,-32.005083342152));
#48205=CARTESIAN_POINT('Origin',(-82.5,-28.9949149203246,-31.7440352836156));
#48206=CARTESIAN_POINT('Origin',(-82.8535533905933,0.,-1.11022302462516E-15));
#48207=CARTESIAN_POINT('Origin',(-82.5,0.,0.));
#48208=CARTESIAN_POINT('',(-82.8535533905844,-33.0858623853674,28.0042879552233));
#48209=CARTESIAN_POINT('Ctrl Pts',(-82.861919052854,-33.0775140978602,28.0008882573809));
#48210=CARTESIAN_POINT('Ctrl Pts',(-82.8591705016505,-33.0803421425098,
28.0020103183848));
#48211=CARTESIAN_POINT('Ctrl Pts',(-82.8563818305258,-33.0831248304814,
28.003144256925));
#48212=CARTESIAN_POINT('Ctrl Pts',(-82.8535533905865,-33.0858623853687,
28.0042879552254));
#48213=CARTESIAN_POINT('Origin',(-82.8535533905933,-1.66533453693773E-15,
0.));
#48214=CARTESIAN_POINT('Origin',(-83.,17.8050341073026,40.5010508850245));
#48215=CARTESIAN_POINT('',(-82.3464466094067,18.0515020953342,39.9659532237599));
#48216=CARTESIAN_POINT('Ctrl Pts',(-82.3464466094067,18.0515020953342,39.9659532237599));
#48217=CARTESIAN_POINT('Ctrl Pts',(-82.4235381014816,18.1006999631463,39.8591415269723));
#48218=CARTESIAN_POINT('Ctrl Pts',(-82.5,18.1497255644298,39.7527038317633));
#48219=CARTESIAN_POINT('',(-82.3223113642133,18.0370907815053,39.9972411016995));
#48220=CARTESIAN_POINT('Ctrl Pts',(-82.3223113642133,18.0370907815053,39.9972411016995));
#48221=CARTESIAN_POINT('Ctrl Pts',(-82.3305312270325,18.0416817288895,39.9872738632445));
#48222=CARTESIAN_POINT('Ctrl Pts',(-82.3386105716178,18.0465013314245,39.9768101999294));
#48223=CARTESIAN_POINT('Ctrl Pts',(-82.3464466094067,18.0515020953342,39.9659532237599));
#48224=CARTESIAN_POINT('',(-76.8294181454841,18.0370907815289,39.9972411016484));
#48225=CARTESIAN_POINT('',(-75.,18.0370907815053,39.9972411016995));
#48226=CARTESIAN_POINT('',(-77.,18.2783610671109,39.4734279826357));
#48227=CARTESIAN_POINT('Ctrl Pts',(-76.8294181454571,18.0370907815373,39.9972411016301));
#48228=CARTESIAN_POINT('Ctrl Pts',(-76.8802846591861,18.065500682451,39.9355614017345));
#48229=CARTESIAN_POINT('Ctrl Pts',(-76.9231860633659,18.1032378673816,39.8536315756326));
#48230=CARTESIAN_POINT('Ctrl Pts',(-76.9817250649226,18.1795903983193,39.6878653799385));
#48231=CARTESIAN_POINT('Ctrl Pts',(-77.,18.233218835034,39.5714346365688));
#48232=CARTESIAN_POINT('Ctrl Pts',(-77.,18.2783610671109,39.4734279826357));
#48233=CARTESIAN_POINT('',(-77.,24.4987646471392,25.9685365994627));
#48234=CARTESIAN_POINT('',(-77.,24.4987646471392,25.9685365994627));
#48235=CARTESIAN_POINT('',(-83.,24.4987646471392,25.9685365994627));
#48236=CARTESIAN_POINT('Origin',(-82.6,0.,0.));
#48237=CARTESIAN_POINT('',(-82.3464466094067,-33.3916700985745,28.4276364302343));
#48238=CARTESIAN_POINT('Ctrl Pts',(-82.3464466094069,-33.3916700985742,
28.4276364302344));
#48239=CARTESIAN_POINT('Ctrl Pts',(-82.3466452959177,-33.391648652821,28.427355119475));
#48240=CARTESIAN_POINT('Ctrl Pts',(-82.346844018298,-33.3916269832502,28.4270740141655));
#48241=CARTESIAN_POINT('Ctrl Pts',(-82.3957553456065,-33.3862395754527,
28.3579486596923));
#48242=CARTESIAN_POINT('Ctrl Pts',(-82.4545593255999,-33.36620626683,28.29064286912));
#48243=CARTESIAN_POINT('Ctrl Pts',(-82.5782395151542,-33.3038745068911,
28.1728689595436));
#48244=CARTESIAN_POINT('Ctrl Pts',(-82.64311889955,-33.2615715101842,28.1224065803701));
#48245=CARTESIAN_POINT('Ctrl Pts',(-82.7513471853223,-33.1789245718431,
28.0525292204883));
#48246=CARTESIAN_POINT('Ctrl Pts',(-82.8029335885286,-33.1348556429589,
28.0247564052626));
#48247=CARTESIAN_POINT('Ctrl Pts',(-82.8535533905865,-33.0858623853687,
28.0042879552254));
#48248=CARTESIAN_POINT('Origin',(-82.3464466094067,-3.33066907387547E-15,
0.));
#48249=CARTESIAN_POINT('Origin',(-75.,-32.8931167434394,28.4656436938016));
#48250=CARTESIAN_POINT('',(-77.,-32.6839376640695,28.0115026223778));
#48251=CARTESIAN_POINT('',(-75.,-32.6839376640695,28.0115026223778));
#48252=CARTESIAN_POINT('',(-77.,-33.2181297628261,28.0856877263144));
#48253=CARTESIAN_POINT('Origin',(-77.,-32.8931167434394,28.4656436938016));
#48254=CARTESIAN_POINT('Ctrl Pts',(-76.5,-33.2711985450881,28.7928350006269));
#48255=CARTESIAN_POINT('Ctrl Pts',(-76.500911294616,-33.2717982978633,28.7921419638468));
#48256=CARTESIAN_POINT('Ctrl Pts',(-76.5018225908806,-33.2723961461827,
28.791447276763));
#48257=CARTESIAN_POINT('Ctrl Pts',(-76.5561204584061,-33.3079042592076,
28.7499574103928));
#48258=CARTESIAN_POINT('Ctrl Pts',(-76.6098195625592,-33.3364800964826,
28.7032660033393));
#48259=CARTESIAN_POINT('Ctrl Pts',(-76.7122026008526,-33.3770567140169,
28.6023347905102));
#48260=CARTESIAN_POINT('Ctrl Pts',(-76.761672636178,-33.3897295300342,28.5476297044676));
#48261=CARTESIAN_POINT('Ctrl Pts',(-76.8500872541283,-33.3951790166836,
28.4352133444499));
#48262=CARTESIAN_POINT('Ctrl Pts',(-76.889996425598,-33.3890059164574,28.3771217427426));
#48263=CARTESIAN_POINT('Ctrl Pts',(-76.9474081328553,-33.3573297979066,
28.2741355362964));
#48264=CARTESIAN_POINT('Ctrl Pts',(-76.9678406878865,-33.336829727842,28.2296235623278));
#48265=CARTESIAN_POINT('Ctrl Pts',(-76.9935652964101,-33.2835955471917,
28.1501559863878));
#48266=CARTESIAN_POINT('Ctrl Pts',(-77.,-33.2533411811723,28.1158074516849));
#48267=CARTESIAN_POINT('Ctrl Pts',(-77.,-33.2181297628261,28.0856877263144));
#48268=CARTESIAN_POINT('Ctrl Pts',(-81.9928932188135,-33.2711985450881,
28.7928350006269));
#48269=CARTESIAN_POINT('Ctrl Pts',(-81.9939470017665,-33.2718920740956,
28.7920336019004));
#48270=CARTESIAN_POINT('Ctrl Pts',(-81.9950007872636,-33.2725830567574,
28.7912299961877));
#48271=CARTESIAN_POINT('Ctrl Pts',(-82.0576631913743,-33.3135201817406,
28.7433131970572));
#48272=CARTESIAN_POINT('Ctrl Pts',(-82.1197538127841,-33.3453729171763,
28.6882973488404));
#48273=CARTESIAN_POINT('Ctrl Pts',(-82.2343773913435,-33.3855972358229,
28.5708455441907));
#48274=CARTESIAN_POINT('Ctrl Pts',(-82.2882331858636,-33.3956551578982,
28.5081013386358));
#48275=CARTESIAN_POINT('Ctrl Pts',(-82.3395113735642,-33.3923414225311,
28.4373899351447));
#48276=CARTESIAN_POINT('Ctrl Pts',(-82.3429958929941,-33.3920425607612,
28.4325221351122));
#48277=CARTESIAN_POINT('Ctrl Pts',(-82.3464466094069,-33.3916700985742,
28.4276364302344));
#48278=CARTESIAN_POINT('Ctrl Pts',(-82.5,-28.5407738489008,-31.5348562042457));
#48279=CARTESIAN_POINT('Ctrl Pts',(-82.3354767269923,-28.3636012869196,
-31.9195090928971));
#48280=CARTESIAN_POINT('Ctrl Pts',(-82.1663384008616,-28.1871794959658,
-32.3025320099479));
#48281=CARTESIAN_POINT('Ctrl Pts',(-81.9928932185014,-28.0115026220617,
-32.6839376647557));
#48282=CARTESIAN_POINT('Ctrl Pts',(-82.601222396877,-28.5243224066161,-31.570573330682));
#48283=CARTESIAN_POINT('Ctrl Pts',(-82.4362685881547,-28.3468680421775,
-31.9558433587761));
#48284=CARTESIAN_POINT('Ctrl Pts',(-82.266696368842,-28.17016995578,-32.3394554481576));
#48285=CARTESIAN_POINT('Ctrl Pts',(-82.0928222766332,-27.9942348651397,
-32.7214270621338));
#48286=CARTESIAN_POINT('Ctrl Pts',(-82.8034223550171,-28.5581838001894,
-31.6726547394673));
#48287=CARTESIAN_POINT('Ctrl Pts',(-82.6376066813012,-28.3799605743899,
-32.0590647631586));
#48288=CARTESIAN_POINT('Ctrl Pts',(-82.4671755612215,-28.202520651421,-32.4437642807502));
#48289=CARTESIAN_POINT('Ctrl Pts',(-82.2924428677096,-28.0258606823619,
-32.8267719987384));
#48290=CARTESIAN_POINT('Ctrl Pts',(-82.9826254704188,-28.7876553692672,
-31.8549987460867));
#48291=CARTESIAN_POINT('Ctrl Pts',(-82.8163920970618,-28.6082163213685,
-32.2423197945722));
#48292=CARTESIAN_POINT('Ctrl Pts',(-82.6455413605155,-28.4295675026153,
-32.6278870365822));
#48293=CARTESIAN_POINT('Ctrl Pts',(-82.4703908997593,-28.2517145084275,
-33.0117234332617));
#48294=CARTESIAN_POINT('Ctrl Pts',(-82.9669916294052,-29.0496559660236,
-31.9689903150268));
#48295=CARTESIAN_POINT('Ctrl Pts',(-82.801451982201,-28.8697784920648,-32.3562635518781));
#48296=CARTESIAN_POINT('Ctrl Pts',(-82.6312976029413,-28.6906846360163,
-32.7417993726423));
#48297=CARTESIAN_POINT('Ctrl Pts',(-82.4568372372109,-28.5123652574907,
-33.1256165828682));
#48298=CARTESIAN_POINT('Ctrl Pts',(-82.8865299173878,-29.1905849277686,
-31.9994877358));
#48299=CARTESIAN_POINT('Ctrl Pts',(-82.7217411730814,-29.0109209132906,
-32.3864371172518));
#48300=CARTESIAN_POINT('Ctrl Pts',(-82.5523328602259,-28.832016226968,-32.771679559501));
#48301=CARTESIAN_POINT('Ctrl Pts',(-82.3786222720913,-28.6538783960759,
-33.1552296123872));
#48302=CARTESIAN_POINT('Ctrl Pts',(-82.8535533905933,-29.2333555023034,
-32.005083342152));
#48303=CARTESIAN_POINT('Ctrl Pts',(-82.6890301175855,-29.0538135025535,
-32.3919004687743));
#48304=CARTESIAN_POINT('Ctrl Pts',(-82.5198917914549,-28.87503008773,-32.7770213250434));
#48305=CARTESIAN_POINT('Ctrl Pts',(-82.3464466090947,-28.6970028852828,
-33.1604609499183));
#48306=CARTESIAN_POINT('',(-81.9928932185014,-28.0115026220617,-32.6839376647557));
#48307=CARTESIAN_POINT('',(-82.3464466090947,-28.6970028851807,-33.1604609498003));
#48308=CARTESIAN_POINT('Origin',(-81.9928932185014,-28.4656436934856,-32.8931167441256));
#48309=CARTESIAN_POINT('Ctrl Pts',(-82.3464466090947,-28.6970028852828,
-33.1604609499183));
#48310=CARTESIAN_POINT('Ctrl Pts',(-82.5198917914549,-28.87503008773,-32.7770213250434));
#48311=CARTESIAN_POINT('Ctrl Pts',(-82.6890301175855,-29.0538135025535,
-32.3919004687743));
#48312=CARTESIAN_POINT('Ctrl Pts',(-82.8535533905933,-29.2333555023034,
-32.005083342152));
#48313=CARTESIAN_POINT('',(-82.5,-28.5407738489008,-31.5348562042457));
#48314=CARTESIAN_POINT('Origin',(-82.5,-28.9949149203246,-31.7440352836156));
#48315=CARTESIAN_POINT('Ctrl Pts',(-82.5,-28.5407738489008,-31.5348562042457));
#48316=CARTESIAN_POINT('Ctrl Pts',(-82.3354767269923,-28.3636012869196,
-31.9195090928971));
#48317=CARTESIAN_POINT('Ctrl Pts',(-82.1663384008616,-28.1871794959658,
-32.3025320099479));
#48318=CARTESIAN_POINT('Ctrl Pts',(-81.9928932185014,-28.0115026220617,
-32.6839376647557));
#48319=CARTESIAN_POINT('Origin',(-82.5,-28.9949149203246,-31.7440352836156));
#48320=CARTESIAN_POINT('Origin',(-82.5,-28.9949149203246,-31.7440352836156));
#48321=CARTESIAN_POINT('Origin',(-75.,-28.4656436938016,-32.8931167434394));
#48322=CARTESIAN_POINT('',(-77.,-28.0856877263144,-33.2181297628261));
#48323=CARTESIAN_POINT('Ctrl Pts',(-76.5,-28.7928350006269,-33.2711985450881));
#48324=CARTESIAN_POINT('Ctrl Pts',(-76.5009112946178,-28.7921419638454,
-33.2717982978645));
#48325=CARTESIAN_POINT('Ctrl Pts',(-76.501822590878,-28.791447276762,-33.2723961461835));
#48326=CARTESIAN_POINT('Ctrl Pts',(-76.5561204584386,-28.7499574104089,
-33.3079042591934));
#48327=CARTESIAN_POINT('Ctrl Pts',(-76.6098195625684,-28.7032660033313,
-33.3364800964874));
#48328=CARTESIAN_POINT('Ctrl Pts',(-76.7122026008691,-28.602334790493,-33.3770567140222));
#48329=CARTESIAN_POINT('Ctrl Pts',(-76.7616726361978,-28.5476297044451,
-33.3897295300385));
#48330=CARTESIAN_POINT('Ctrl Pts',(-76.8500872541471,-28.4352133444235,
-33.3951790166818));
#48331=CARTESIAN_POINT('Ctrl Pts',(-76.8899964256134,-28.3771217427184,
-33.3890059164528));
#48332=CARTESIAN_POINT('Ctrl Pts',(-76.9474081328652,-28.2741355362761,
-33.3573297978981));
#48333=CARTESIAN_POINT('Ctrl Pts',(-76.9678406878941,-28.2296235623091,
-33.3368297278319));
#48334=CARTESIAN_POINT('Ctrl Pts',(-76.9935652964121,-28.1501559863774,
-33.2835955471825));
#48335=CARTESIAN_POINT('Ctrl Pts',(-77.,-28.1158074516803,-33.2533411811668));
#48336=CARTESIAN_POINT('Ctrl Pts',(-77.,-28.0856877263144,-33.2181297628261));
#48337=CARTESIAN_POINT('',(-81.9928932188135,-27.9656436938016,-32.8931167438896));
#48338=CARTESIAN_POINT('Origin',(-81.9928932188135,-28.4656436938016,-32.8931167434394));
#48339=CARTESIAN_POINT('Origin',(-81.9928932188135,-28.4656436938016,-32.8931167434394));
#48340=CARTESIAN_POINT('',(-77.,-28.0115026223778,-32.6839376640695));
#48341=CARTESIAN_POINT('',(-75.,-28.0115026223778,-32.6839376640695));
#48342=CARTESIAN_POINT('Origin',(-77.,-28.4656436938016,-32.8931167434394));
#48343=CARTESIAN_POINT('Origin',(-81.9928932188135,-28.4656436932813,-32.8931167438896));
#48344=CARTESIAN_POINT('Origin',(-81.9928932188135,-28.4656436932813,-32.8931167438896));
#48345=CARTESIAN_POINT('',(-82.050443104264,-27.9740691449652,-32.9641271243453));
#48346=CARTESIAN_POINT('Origin',(-81.9928932188135,-28.4656436932813,-32.8931167438896));
#48347=CARTESIAN_POINT('Origin',(-83.,-40.5010508850245,17.8050341073026));
#48348=CARTESIAN_POINT('',(-82.3464466094067,-39.9659532237599,18.0515020953342));
#48349=CARTESIAN_POINT('Ctrl Pts',(-82.3464466094067,-39.9659532237599,
18.0515020953342));
#48350=CARTESIAN_POINT('Ctrl Pts',(-82.4235381014816,-39.8591415269723,
18.1006999631463));
#48351=CARTESIAN_POINT('Ctrl Pts',(-82.5,-39.7527038317633,18.1497255644298));
#48352=CARTESIAN_POINT('',(-82.3223113642133,-39.9972411016995,18.0370907815053));
#48353=CARTESIAN_POINT('Ctrl Pts',(-82.3223113642133,-39.9972411016995,
18.0370907815053));
#48354=CARTESIAN_POINT('Ctrl Pts',(-82.3305312270325,-39.9872738632445,
18.0416817288895));
#48355=CARTESIAN_POINT('Ctrl Pts',(-82.3386105716178,-39.9768101999294,
18.0465013314245));
#48356=CARTESIAN_POINT('Ctrl Pts',(-82.3464466094067,-39.9659532237599,
18.0515020953341));
#48357=CARTESIAN_POINT('',(-76.8294181454841,-39.9972411016484,18.0370907815288));
#48358=CARTESIAN_POINT('',(-75.,-39.9972411016995,18.0370907815053));
#48359=CARTESIAN_POINT('',(-77.,-39.4734279826357,18.2783610671109));
#48360=CARTESIAN_POINT('Ctrl Pts',(-76.8294181454571,-39.9972411016301,
18.0370907815373));
#48361=CARTESIAN_POINT('Ctrl Pts',(-76.8802846591861,-39.9355614017345,
18.065500682451));
#48362=CARTESIAN_POINT('Ctrl Pts',(-76.9231860633659,-39.8536315756326,
18.1032378673816));
#48363=CARTESIAN_POINT('Ctrl Pts',(-76.9817250649226,-39.6878653799385,
18.1795903983192));
#48364=CARTESIAN_POINT('Ctrl Pts',(-77.,-39.5714346365688,18.233218835034));
#48365=CARTESIAN_POINT('Ctrl Pts',(-77.,-39.4734279826357,18.2783610671109));
#48366=CARTESIAN_POINT('',(-77.,-25.9685365994627,24.4987646471392));
#48367=CARTESIAN_POINT('',(-77.,-25.9685365994627,24.4987646471392));
#48368=CARTESIAN_POINT('',(-83.,-25.9685365994627,24.4987646471392));
#48369=CARTESIAN_POINT('Origin',(-82.6,0.,0.));
#48370=CARTESIAN_POINT('Origin',(-82.3464466094067,0.,1.11022302462516E-15));
#48371=CARTESIAN_POINT('Origin',(-81.9928932188135,0.,0.));
#48372=CARTESIAN_POINT('Ctrl Pts',(-81.9928932188135,-40.2453960685632,
17.7850525803124));
#48373=CARTESIAN_POINT('Ctrl Pts',(-81.9939472381724,-40.2449675863739,
17.7860221830357));
#48374=CARTESIAN_POINT('Ctrl Pts',(-81.9950012600764,-40.2445360196401,
17.7869904254498));
#48375=CARTESIAN_POINT('Ctrl Pts',(-82.0547007770009,-40.2199175482614,
17.8417542131912));
#48376=CARTESIAN_POINT('Ctrl Pts',(-82.1137599900357,-40.186017191161,17.891710645152));
#48377=CARTESIAN_POINT('Ctrl Pts',(-82.2236189798636,-40.1028545535996,
17.9756182289286));
#48378=CARTESIAN_POINT('Ctrl Pts',(-82.2755452949045,-40.0539486860789,
18.0109710556312));
#48379=CARTESIAN_POINT('Ctrl Pts',(-82.3223113642133,-39.9972411016995,
18.0370907815053));
#48380=CARTESIAN_POINT('Origin',(-75.,-39.7880620223296,17.5829497100815));
#48381=CARTESIAN_POINT('Ctrl Pts',(-76.829418145442,-39.9972411016484,18.0370907815288));
#48382=CARTESIAN_POINT('Ctrl Pts',(-76.7894304995805,-40.0457293076422,
18.0147569321475));
#48383=CARTESIAN_POINT('Ctrl Pts',(-76.7456834207506,-40.088484052965,17.9856744463975));
#48384=CARTESIAN_POINT('Ctrl Pts',(-76.6365588529939,-40.1769760907868,
17.9049698494587));
#48385=CARTESIAN_POINT('Ctrl Pts',(-76.5686581389593,-40.2173075134492,
17.8481334281707));
#48386=CARTESIAN_POINT('Ctrl Pts',(-76.5009411428971,-40.2450128585448,
17.7859180752662));
#48387=CARTESIAN_POINT('Ctrl Pts',(-76.5004705713342,-40.2452047709046,
17.7854854634878));
#48388=CARTESIAN_POINT('Ctrl Pts',(-76.5,-40.2453960685632,17.7850525803123));
#48389=CARTESIAN_POINT('Origin',(-83.,-28.4786855519014,29.9484575042249));
#48390=CARTESIAN_POINT('',(-77.,-28.4786855519014,29.9484575042249));
#48391=CARTESIAN_POINT('',(-83.,-28.4786855519014,29.9484575042249));
#48392=CARTESIAN_POINT('',(-77.,-43.0111998374632,23.2547269643883));
#48393=CARTESIAN_POINT('Origin',(-81.9928932188135,0.,0.));
#48394=CARTESIAN_POINT('Ctrl Pts',(-81.9928932188135,17.7850525803123,40.2453960685632));
#48395=CARTESIAN_POINT('Ctrl Pts',(-81.9939472381728,17.786022183036,40.2449675863738));
#48396=CARTESIAN_POINT('Ctrl Pts',(-81.9950012600754,17.7869904254506,40.2445360196398));
#48397=CARTESIAN_POINT('Ctrl Pts',(-82.0547007770136,17.84175421318,40.2199175482663));
#48398=CARTESIAN_POINT('Ctrl Pts',(-82.1137599900355,17.8917106451519,40.1860171911611));
#48399=CARTESIAN_POINT('Ctrl Pts',(-82.2236189798635,17.9756182289286,40.1028545535997));
#48400=CARTESIAN_POINT('Ctrl Pts',(-82.2755452949045,18.0109710556312,40.0539486860789));
#48401=CARTESIAN_POINT('Ctrl Pts',(-82.3223113642133,18.0370907815053,39.9972411016995));
#48402=CARTESIAN_POINT('Origin',(-75.,17.5829497100815,39.7880620223296));
#48403=CARTESIAN_POINT('Ctrl Pts',(-76.829418145442,18.0370907815289,39.9972411016484));
#48404=CARTESIAN_POINT('Ctrl Pts',(-76.7894304995805,18.0147569321475,40.0457293076422));
#48405=CARTESIAN_POINT('Ctrl Pts',(-76.7456834207506,17.9856744463976,40.088484052965));
#48406=CARTESIAN_POINT('Ctrl Pts',(-76.6365588529938,17.9049698494586,40.176976090787));
#48407=CARTESIAN_POINT('Ctrl Pts',(-76.5686581389664,17.8481334281635,40.2173075134524));
#48408=CARTESIAN_POINT('Ctrl Pts',(-76.5009411428974,17.7859180752668,40.2450128585445));
#48409=CARTESIAN_POINT('Ctrl Pts',(-76.5004705713336,17.7854854634873,40.2452047709049));
#48410=CARTESIAN_POINT('Ctrl Pts',(-76.5,17.7850525803123,40.2453960685632));
#48411=CARTESIAN_POINT('Origin',(-83.,29.9484575042249,28.4786855519015));
#48412=CARTESIAN_POINT('',(-77.,29.9484575042249,28.4786855519015));
#48413=CARTESIAN_POINT('',(-83.,29.9484575042249,28.4786855519015));
#48414=CARTESIAN_POINT('',(-77.,23.2547269643883,43.0111998374633));
#48415=CARTESIAN_POINT('Ctrl Pts',(-81.9928932223231,39.9972410968818,-18.0370907837244));
#48416=CARTESIAN_POINT('Ctrl Pts',(-82.1628343230695,39.7639623455707,-18.1445398507793));
#48417=CARTESIAN_POINT('Ctrl Pts',(-82.331886307423,39.530149144004,-18.2522350876248));
#48418=CARTESIAN_POINT('Ctrl Pts',(-82.5,39.2957805952595,-18.3601861194615));
#48419=CARTESIAN_POINT('Ctrl Pts',(-82.1335529082636,40.0817756848435,-17.9981538357199));
#48420=CARTESIAN_POINT('Ctrl Pts',(-82.303363849546,39.8479876918321,-18.1058233857611));
#48421=CARTESIAN_POINT('Ctrl Pts',(-82.4723016542503,39.6136883508133,-18.2137706610956));
#48422=CARTESIAN_POINT('Ctrl Pts',(-82.6402844586922,39.3787952697101,-18.321949249316));
#48423=CARTESIAN_POINT('Ctrl Pts',(-82.2718712658937,40.1264553236608,-17.87639229832));
#48424=CARTESIAN_POINT('Ctrl Pts',(-82.4415798928791,39.8923864524203,-17.9847127214014));
#48425=CARTESIAN_POINT('Ctrl Pts',(-82.6104201587052,39.6578020933961,-18.0933094953168));
#48426=CARTESIAN_POINT('Ctrl Pts',(-82.7782997031823,39.422614172472,-18.2021497484197));
#48427=CARTESIAN_POINT('Ctrl Pts',(-82.3464466129164,40.1114460228581,-17.7258580223676));
#48428=CARTESIAN_POINT('Ctrl Pts',(-82.5163877136628,39.8775346219,-17.8347386981006));
#48429=CARTESIAN_POINT('Ctrl Pts',(-82.6854396980163,39.6430704046442,-17.9438814038579));
#48430=CARTESIAN_POINT('Ctrl Pts',(-82.8535533905933,39.4080313955299,-18.0532959647562));
#48431=CARTESIAN_POINT('',(-82.5,39.2957805952595,-18.3601861194615));
#48432=CARTESIAN_POINT('Origin',(-82.5,39.0866015158896,-17.9060450480377));
#48433=CARTESIAN_POINT('',(-81.9928932223231,39.9972410992906,-18.0370907826149));
#48434=CARTESIAN_POINT('Origin',(-81.9928932223231,39.7880620175119,-17.5829497123006));
#48435=CARTESIAN_POINT('Ctrl Pts',(-81.9928932223231,39.9972410968818,-18.0370907837244));
#48436=CARTESIAN_POINT('Ctrl Pts',(-82.1628343230695,39.7639623455707,-18.1445398507793));
#48437=CARTESIAN_POINT('Ctrl Pts',(-82.331886307423,39.530149144004,-18.2522350876248));
#48438=CARTESIAN_POINT('Ctrl Pts',(-82.5,39.2957805952595,-18.3601861194615));
#48439=CARTESIAN_POINT('Origin',(-82.5,39.0866015158896,-17.9060450480377));
#48440=CARTESIAN_POINT('Origin',(-82.5,39.0866015158896,-17.9060450480377));
#48441=CARTESIAN_POINT('Origin',(-81.9928932223231,39.7880620223296,-17.5829497100815));
#48442=CARTESIAN_POINT('Origin',(-81.9928932223231,39.7880620223296,-17.5829497100815));
#48443=CARTESIAN_POINT('Origin',(-82.5,44.7879994647011,-15.2799597870972));
#48444=CARTESIAN_POINT('',(-82.5,25.9685365994627,-24.4987646471392));
#48445=CARTESIAN_POINT('',(-82.5,44.997178544071,-15.734100858521));
#48446=CARTESIAN_POINT('Origin',(-82.5,25.7593575200928,-24.0446235757154));
#48447=CARTESIAN_POINT('Origin',(-83.,40.5010508850245,-17.8050341073026));
#48448=CARTESIAN_POINT('',(-76.8294181454841,39.9972411016484,-18.0370907815289));
#48449=CARTESIAN_POINT('',(-75.,39.9972411016995,-18.0370907815054));
#48450=CARTESIAN_POINT('',(-77.,39.4734279826357,-18.2783610671109));
#48451=CARTESIAN_POINT('Ctrl Pts',(-76.8294181454571,39.99724110163,-18.0370907815373));
#48452=CARTESIAN_POINT('Ctrl Pts',(-76.8802846591861,39.9355614017345,-18.065500682451));
#48453=CARTESIAN_POINT('Ctrl Pts',(-76.9231860633659,39.8536315756326,-18.1032378673816));
#48454=CARTESIAN_POINT('Ctrl Pts',(-76.9817250649226,39.6878653799385,-18.1795903983193));
#48455=CARTESIAN_POINT('Ctrl Pts',(-77.,39.5714346365688,-18.233218835034));
#48456=CARTESIAN_POINT('Ctrl Pts',(-77.,39.4734279826357,-18.2783610671109));
#48457=CARTESIAN_POINT('',(-77.,25.9685365994627,-24.4987646471392));
#48458=CARTESIAN_POINT('',(-77.,25.9685365994627,-24.4987646471392));
#48459=CARTESIAN_POINT('',(-83.,25.9685365994627,-24.4987646471392));
#48460=CARTESIAN_POINT('Origin',(-75.,39.7880620223296,-17.5829497100815));
#48461=CARTESIAN_POINT('Ctrl Pts',(-76.829418145442,39.9972411016484,-18.0370907815289));
#48462=CARTESIAN_POINT('Ctrl Pts',(-76.7894304995805,40.0457293076422,-18.0147569321475));
#48463=CARTESIAN_POINT('Ctrl Pts',(-76.7456834207506,40.088484052965,-17.9856744463975));
#48464=CARTESIAN_POINT('Ctrl Pts',(-76.6365588529939,40.1769760907868,-17.9049698494588));
#48465=CARTESIAN_POINT('Ctrl Pts',(-76.5686581389598,40.2173075134493,-17.8481334281704));
#48466=CARTESIAN_POINT('Ctrl Pts',(-76.5009411428979,40.2450128585444,-17.785918075267));
#48467=CARTESIAN_POINT('Ctrl Pts',(-76.5004705713334,40.245204770905,-17.7854854634871));
#48468=CARTESIAN_POINT('Ctrl Pts',(-76.5,40.2453960685632,-17.7850525803124));
#48469=CARTESIAN_POINT('Origin',(-75.,-17.5829497100816,-39.7880620223296));
#48470=CARTESIAN_POINT('',(-81.9928932188135,-18.0370907815054,-39.9972411016994));
#48471=CARTESIAN_POINT('Origin',(-81.9928932188135,-17.5829497100816,-39.7880620223296));
#48472=CARTESIAN_POINT('',(-76.8294181454841,-18.0370907815289,-39.9972411016484));
#48473=CARTESIAN_POINT('Ctrl Pts',(-76.829418145442,-18.0370907815289,-39.9972411016484));
#48474=CARTESIAN_POINT('Ctrl Pts',(-76.7894304995805,-18.0147569321475,
-40.0457293076422));
#48475=CARTESIAN_POINT('Ctrl Pts',(-76.7456834207506,-17.9856744463976,
-40.088484052965));
#48476=CARTESIAN_POINT('Ctrl Pts',(-76.6365588529926,-17.9049698494578,
-40.1769760907878));
#48477=CARTESIAN_POINT('Ctrl Pts',(-76.5686581390476,-17.8481334280872,
-40.2173075134863));
#48478=CARTESIAN_POINT('Ctrl Pts',(-76.5009411428928,-17.7859180752669,
-40.2450128585444));
#48479=CARTESIAN_POINT('Ctrl Pts',(-76.5004705713346,-17.7854854634883,
-40.2452047709044));
#48480=CARTESIAN_POINT('Ctrl Pts',(-76.5,-17.7850525803124,-40.2453960685632));
#48481=CARTESIAN_POINT('',(-75.,-18.0370907815054,-39.9972411016994));
#48482=CARTESIAN_POINT('Ctrl Pts',(-81.9928932188135,-18.0370907815054,
-39.9972411016994));
#48483=CARTESIAN_POINT('Ctrl Pts',(-82.162834320742,-18.1445398492965,-39.7639623487899));
#48484=CARTESIAN_POINT('Ctrl Pts',(-82.3318863062657,-18.2522350868817,
-39.5301491456174));
#48485=CARTESIAN_POINT('Ctrl Pts',(-82.5,-18.3601861194615,-39.2957805952595));
#48486=CARTESIAN_POINT('Ctrl Pts',(-82.1335529047565,-17.9981538334961,
-40.0817756896715));
#48487=CARTESIAN_POINT('Ctrl Pts',(-82.3033638472202,-18.105823384275,-39.8479876950582));
#48488=CARTESIAN_POINT('Ctrl Pts',(-82.4723016530939,-18.2137706603509,
-39.6136883524303));
#48489=CARTESIAN_POINT('Ctrl Pts',(-82.6402844586922,-18.321949249316,-39.3787952697101));
#48490=CARTESIAN_POINT('Ctrl Pts',(-82.2718712623887,-17.8763922960829,
-40.1264553284945));
#48491=CARTESIAN_POINT('Ctrl Pts',(-82.4415798905547,-17.9847127199064,
-39.8923864556503));
#48492=CARTESIAN_POINT('Ctrl Pts',(-82.6104201575495,-18.0933094945676,
-39.6578020950152));
#48493=CARTESIAN_POINT('Ctrl Pts',(-82.7782997031823,-18.2021497484197,
-39.422614172472));
#48494=CARTESIAN_POINT('Ctrl Pts',(-82.3464466094067,-17.725858020119,-40.1114460276889));
#48495=CARTESIAN_POINT('Ctrl Pts',(-82.5163877113353,-17.834738696598,-39.8775346251281));
#48496=CARTESIAN_POINT('Ctrl Pts',(-82.6854396968589,-17.9438814031046,
-39.6430704062622));
#48497=CARTESIAN_POINT('Ctrl Pts',(-82.8535533905932,-18.0532959647562,
-39.4080313955299));
#48498=CARTESIAN_POINT('',(-82.5,-18.3601861194615,-39.2957805952595));
#48499=CARTESIAN_POINT('',(-82.8535533905932,-18.0532959647562,-39.4080313955299));
#48500=CARTESIAN_POINT('Origin',(-82.5,-17.9060450480377,-39.0866015158896));
#48501=CARTESIAN_POINT('',(-82.3464466094067,-17.725858020119,-40.1114460276889));
#48502=CARTESIAN_POINT('Ctrl Pts',(-82.8535533905932,-18.0532959647562,
-39.4080313955299));
#48503=CARTESIAN_POINT('Ctrl Pts',(-82.6854396968589,-17.9438814031046,
-39.6430704062622));
#48504=CARTESIAN_POINT('Ctrl Pts',(-82.5163877113353,-17.834738696598,-39.8775346251281));
#48505=CARTESIAN_POINT('Ctrl Pts',(-82.3464466094067,-17.725858020119,-40.1114460276889));
#48506=CARTESIAN_POINT('Origin',(-81.9928932188135,-17.5829497100816,-39.7880620223296));
#48507=CARTESIAN_POINT('Ctrl Pts',(-81.9928932188135,-18.0370907815054,
-39.9972411016994));
#48508=CARTESIAN_POINT('Ctrl Pts',(-82.162834320742,-18.1445398492965,-39.7639623487899));
#48509=CARTESIAN_POINT('Ctrl Pts',(-82.3318863062657,-18.2522350868817,
-39.5301491456174));
#48510=CARTESIAN_POINT('Ctrl Pts',(-82.5,-18.3601861194615,-39.2957805952595));
#48511=CARTESIAN_POINT('Origin',(-82.5,-17.9060450480377,-39.0866015158896));
#48512=CARTESIAN_POINT('Origin',(-82.5,-17.9060450480377,-39.0866015158896));
#48513=CARTESIAN_POINT('Origin',(-82.5,-17.9060450480377,-39.0866015158896));
#48514=CARTESIAN_POINT('Origin',(-81.9928932188135,-17.5829497100816,-39.7880620223295));
#48515=CARTESIAN_POINT('Origin',(-81.9928932188135,-17.5829497100816,-39.7880620223295));
#48516=CARTESIAN_POINT('Origin',(-81.9928932188135,0.,0.));
#48517=CARTESIAN_POINT('',(-82.3464466094067,33.1604609492284,-28.6970028856031));
#48518=CARTESIAN_POINT('Origin',(-82.3464466094067,2.22044604925031E-15,
0.));
#48519=CARTESIAN_POINT('Origin',(-81.9928932188135,32.8931167434394,-28.4656436938016));
#48520=CARTESIAN_POINT('Origin',(-82.6,0.,0.));
#48521=CARTESIAN_POINT('',(-82.8535533905933,32.005083342152,-29.2333555023034));
#48522=CARTESIAN_POINT('Origin',(-82.8535533905933,2.22044604925031E-15,
0.));
#48523=CARTESIAN_POINT('Ctrl Pts',(-82.3464466094067,33.1604609492285,-28.6970028856031));
#48524=CARTESIAN_POINT('Ctrl Pts',(-82.519891807541,32.777021289468,-28.8750301042473));
#48525=CARTESIAN_POINT('Ctrl Pts',(-82.6890303136401,32.3919000078227,-29.0538137165052));
#48526=CARTESIAN_POINT('Ctrl Pts',(-82.8535533905933,32.005083342152,-29.2333555023034));
#48527=CARTESIAN_POINT('Origin',(-76.5,0.,0.));
#48528=CARTESIAN_POINT('',(-77.,-18.2783610671109,-39.4734279826357));
#48529=CARTESIAN_POINT('Origin',(-77.,0.,0.));
#48530=CARTESIAN_POINT('Ctrl Pts',(-76.8294181454571,-18.0370907815373,
-39.99724110163));
#48531=CARTESIAN_POINT('Ctrl Pts',(-76.8802846591861,-18.065500682451,-39.9355614017345));
#48532=CARTESIAN_POINT('Ctrl Pts',(-76.9231860633659,-18.1032378673816,
-39.8536315756326));
#48533=CARTESIAN_POINT('Ctrl Pts',(-76.9817250649226,-18.1795903983193,
-39.6878653799385));
#48534=CARTESIAN_POINT('Ctrl Pts',(-77.,-18.233218835034,-39.5714346365688));
#48535=CARTESIAN_POINT('Ctrl Pts',(-77.,-18.2783610671109,-39.4734279826356));
#48536=CARTESIAN_POINT('Origin',(-77.,-23.8767458057638,-34.489868218463));
#48537=CARTESIAN_POINT('',(-77.,-29.9484575042249,-28.4786855519014));
#48538=CARTESIAN_POINT('',(-77.,-23.2547269643883,-43.0111998374633));
#48539=CARTESIAN_POINT('',(-77.,-24.4987646471392,-25.9685365994627));
#48540=CARTESIAN_POINT('Origin',(-77.,-27.2236110756821,-27.2236110756821));
#48541=CARTESIAN_POINT('',(-77.,-24.4987646471392,-25.9685365994627));
#48542=CARTESIAN_POINT('',(-77.,-27.2236110756821,-25.4736110756821));
#48543=CARTESIAN_POINT('Origin',(-77.,-27.2236110756821,-27.2236110756821));
#48544=CARTESIAN_POINT('Origin',(-81.9928932188135,32.8931167434394,-28.4656436938016));
#48545=CARTESIAN_POINT('',(-81.9928932188135,32.6839376640695,-28.0115026223778));
#48546=CARTESIAN_POINT('Origin',(-81.9928932188135,32.8931167434394,-28.4656436938016));
#48547=CARTESIAN_POINT('Origin',(-81.9928932188135,32.8931167434394,-28.4656436938016));
#48548=CARTESIAN_POINT('Ctrl Pts',(-82.5,31.5348562042457,-28.5407738489008));
#48549=CARTESIAN_POINT('Ctrl Pts',(-82.3354769230468,31.9195086345245,-28.3636014980477));
#48550=CARTESIAN_POINT('Ctrl Pts',(-82.1663384169477,32.3025319745614,-28.187179512265));
#48551=CARTESIAN_POINT('Ctrl Pts',(-81.9928932188134,32.6839376640695,-28.0115026223778));
#48552=CARTESIAN_POINT('Ctrl Pts',(-82.601222396877,31.5705733306819,-28.5243224066161));
#48553=CARTESIAN_POINT('Ctrl Pts',(-82.4362687847223,31.9558428996681,-28.3468682536414));
#48554=CARTESIAN_POINT('Ctrl Pts',(-82.2666963849679,32.3394554127185,-28.1701699721031));
#48555=CARTESIAN_POINT('Ctrl Pts',(-82.092822276946,32.7214270614466,-27.9942348654562));
#48556=CARTESIAN_POINT('Ctrl Pts',(-82.8034223550171,31.6726547394673,-28.5581838001894));
#48557=CARTESIAN_POINT('Ctrl Pts',(-82.6376068788958,32.0590643026922,-28.3799607867701));
#48558=CARTESIAN_POINT('Ctrl Pts',(-82.4671755774271,32.4437642452149,-28.2025206678114));
#48559=CARTESIAN_POINT('Ctrl Pts',(-82.292442868024,32.8267719980494,-28.0258606826798));
#48560=CARTESIAN_POINT('Ctrl Pts',(-82.9826254704188,31.8549987460867,-28.7876553692672));
#48561=CARTESIAN_POINT('Ctrl Pts',(-82.8163922951542,32.2423193330201,-28.6082165351974));
#48562=CARTESIAN_POINT('Ctrl Pts',(-82.6455413767597,32.62788700097,-28.4295675191164));
#48563=CARTESIAN_POINT('Ctrl Pts',(-82.4703909000744,33.0117234325711,-28.2517145087475));
#48564=CARTESIAN_POINT('Ctrl Pts',(-82.9669916294051,31.9689903150268,-29.0496559660236));
#48565=CARTESIAN_POINT('Ctrl Pts',(-82.8014521794668,32.356263090383,-28.8697787064162));
#48566=CARTESIAN_POINT('Ctrl Pts',(-82.6312976191216,32.7417993370319,-28.6906846525606));
#48567=CARTESIAN_POINT('Ctrl Pts',(-82.4568372375248,33.1256165821777,-28.5123652578115));
#48568=CARTESIAN_POINT('Ctrl Pts',(-82.8865299173878,31.9994877358,-29.1905849277686));
#48569=CARTESIAN_POINT('Ctrl Pts',(-82.7217413694523,32.3864366561427,-29.0109211273876));
#48570=CARTESIAN_POINT('Ctrl Pts',(-82.5523328763366,32.7716795239154,-28.8320162434955));
#48571=CARTESIAN_POINT('Ctrl Pts',(-82.3786222724039,33.1552296116972,-28.6538783963964));
#48572=CARTESIAN_POINT('Ctrl Pts',(-82.8535533905933,32.005083342152,-29.2333555023034));
#48573=CARTESIAN_POINT('Ctrl Pts',(-82.6890303136401,32.3919000078227,-29.0538137165052));
#48574=CARTESIAN_POINT('Ctrl Pts',(-82.519891807541,32.777021289468,-28.8750301042473));
#48575=CARTESIAN_POINT('Ctrl Pts',(-82.3464466094067,33.1604609492285,-28.6970028856031));
#48576=CARTESIAN_POINT('',(-82.5,31.5348562042457,-28.5407738489008));
#48577=CARTESIAN_POINT('Origin',(-82.5,31.7440352836156,-28.9949149203246));
#48578=CARTESIAN_POINT('Ctrl Pts',(-82.5,31.5348562042457,-28.5407738489008));
#48579=CARTESIAN_POINT('Ctrl Pts',(-82.3354769230468,31.9195086345245,-28.3636014980477));
#48580=CARTESIAN_POINT('Ctrl Pts',(-82.1663384169477,32.3025319745614,-28.187179512265));
#48581=CARTESIAN_POINT('Ctrl Pts',(-81.9928932188134,32.6839376640695,-28.0115026223778));
#48582=CARTESIAN_POINT('Origin',(-75.,32.8931167434394,-28.4656436938016));
#48583=CARTESIAN_POINT('',(-77.,33.2181297628261,-28.0856877263144));
#48584=CARTESIAN_POINT('Ctrl Pts',(-76.5,33.2711985450881,-28.792835000627));
#48585=CARTESIAN_POINT('Ctrl Pts',(-76.500911294617,33.2717982978639,-28.7921419638461));
#48586=CARTESIAN_POINT('Ctrl Pts',(-76.5018225908797,33.272396146182,-28.7914472767637));
#48587=CARTESIAN_POINT('Ctrl Pts',(-76.5561204583968,33.3079042592016,-28.7499574103998));
#48588=CARTESIAN_POINT('Ctrl Pts',(-76.6098195625408,33.3364800964727,-28.7032660033553));
#48589=CARTESIAN_POINT('Ctrl Pts',(-76.712202600818,33.3770567140056,-28.6023347905465));
#48590=CARTESIAN_POINT('Ctrl Pts',(-76.7616726361363,33.389729530025,-28.5476297045151));
#48591=CARTESIAN_POINT('Ctrl Pts',(-76.8500872540886,33.3951790166874,-28.4352133445057));
#48592=CARTESIAN_POINT('Ctrl Pts',(-76.8899964255655,33.3890059164671,-28.377121742794));
#48593=CARTESIAN_POINT('Ctrl Pts',(-76.9474081328343,33.3573297979245,-28.2741355363395));
#48594=CARTESIAN_POINT('Ctrl Pts',(-76.9678406878704,33.3368297278632,-28.2296235623672));
#48595=CARTESIAN_POINT('Ctrl Pts',(-76.9935652964059,33.283595547211,-28.1501559864099));
#48596=CARTESIAN_POINT('Ctrl Pts',(-77.,33.2533411811838,-28.1158074516948));
#48597=CARTESIAN_POINT('Ctrl Pts',(-77.,33.2181297628261,-28.0856877263145));
#48598=CARTESIAN_POINT('',(-77.,32.6839376640695,-28.0115026223778));
#48599=CARTESIAN_POINT('',(-75.,32.6839376640695,-28.0115026223778));
#48600=CARTESIAN_POINT('Origin',(-77.,32.8931167434394,-28.4656436938016));
#48601=CARTESIAN_POINT('Origin',(-82.5,0.,0.));
#48602=CARTESIAN_POINT('Origin',(-82.5,31.7440352836156,-28.9949149203246));
#48603=CARTESIAN_POINT('Origin',(-82.5,-19.7071756188355,-35.1762326125546));
#48604=CARTESIAN_POINT('',(-82.5,-24.4987646471392,-25.9685365994627));
#48605=CARTESIAN_POINT('',(-82.5,-20.1613166902593,-35.3854116919245));
#48606=CARTESIAN_POINT('Origin',(-82.5,-24.0446235757154,-25.7593575200928));
#48607=CARTESIAN_POINT('Origin',(-82.5,-27.2236110756821,-27.2236110756821));
#48608=CARTESIAN_POINT('',(-82.5,-29.9484575042249,-28.4786855519014));
#48609=CARTESIAN_POINT('Origin',(-82.5,-30.4025985756487,-28.6878646312713));
#48610=CARTESIAN_POINT('Origin',(-82.5,-27.2236110756821,-27.2236110756821));
#48611=CARTESIAN_POINT('Origin',(-82.5,-29.4120158886871,-30.8384825809522));
#48612=CARTESIAN_POINT('',(-82.5,-28.9578748172633,-30.6293035015823));
#48613=CARTESIAN_POINT('Origin',(-82.5,31.7440352836156,-28.9949149203246));
#48614=CARTESIAN_POINT('Origin',(-82.5,31.7440352836156,-28.9949149203246));
#48615=CARTESIAN_POINT('Origin',(-83.,-17.8050341073026,-40.5010508850245));
#48616=CARTESIAN_POINT('',(-83.,-24.4987646471392,-25.9685365994627));
#48617=CARTESIAN_POINT('Origin',(-83.,28.4786855519014,-29.9484575042249));
#48618=CARTESIAN_POINT('',(-82.5,28.4786855519014,-29.9484575042249));
#48619=CARTESIAN_POINT('',(-82.5,40.2410703537288,-24.530658985525));
#48620=CARTESIAN_POINT('',(-77.,28.4786855519014,-29.9484575042249));
#48621=CARTESIAN_POINT('',(-83.,28.4786855519014,-29.9484575042249));
#48622=CARTESIAN_POINT('',(-77.,43.0111998374633,-23.2547269643883));
#48623=CARTESIAN_POINT('Origin',(-82.5,40.4502494330987,-24.9848000569488));
#48624=CARTESIAN_POINT('Origin',(-82.5,28.6878646312713,-30.4025985756487));
#48625=CARTESIAN_POINT('Origin',(-82.5,27.2236110756821,-27.2236110756821));
#48626=CARTESIAN_POINT('Origin',(-82.5,27.2236110756821,-27.2236110756821));
#48627=CARTESIAN_POINT('Origin',(-83.,27.2236110756821,-27.2236110756821));
#48628=CARTESIAN_POINT('Origin',(-77.,27.2236110756821,-27.2236110756821));
#48629=CARTESIAN_POINT('Origin',(-76.5,-27.2236110756821,-27.2236110756821));
#48630=CARTESIAN_POINT('',(-76.5,-27.2236110756821,-25.9736110756821));
#48631=CARTESIAN_POINT('Origin',(-76.5,-27.2236110756821,-25.4736110756821));
#48632=CARTESIAN_POINT('Origin',(-76.5,-27.2236110756821,-27.2236110756821));
#48633=CARTESIAN_POINT('Origin',(-83.,-27.2236110756821,-27.2236110756821));
#48634=CARTESIAN_POINT('',(-67.5,-27.2236110756821,-25.9736110756821));
#48635=CARTESIAN_POINT('',(-83.,-27.2236110756821,-25.9736110756821));
#48636=CARTESIAN_POINT('',(-67.5,-27.2236110756821,-28.4736110756821));
#48637=CARTESIAN_POINT('Origin',(-67.5,-27.2236110756821,-27.2236110756821));
#48638=CARTESIAN_POINT('Origin',(-67.5,-27.2236110756821,-27.2236110756821));
#48639=CARTESIAN_POINT('Origin',(-10.5,-26.1629509039023,-33.9411254969543));
#48640=CARTESIAN_POINT('',(-10.5,-25.809397513309,-34.2946788875476));
#48641=CARTESIAN_POINT('',(-10.,-26.1629509039023,-33.9411254969543));
#48642=CARTESIAN_POINT('Origin',(-10.5,-26.1629509039023,-33.9411254969543));
#48643=CARTESIAN_POINT('',(-10.5,-26.5165042944955,-34.2946788875476));
#48644=CARTESIAN_POINT('Origin',(-10.5,-26.1629509039023,-33.9411254969543));
#48645=CARTESIAN_POINT('Origin',(-10.5,-26.1629509039023,-33.9411254969543));
#48646=CARTESIAN_POINT('Origin',(-10.5,-23.4052344572747,-31.1834090503267));
#48647=CARTESIAN_POINT('',(-10.5,-21.708178182427,-30.1934595566656));
#48648=CARTESIAN_POINT('',(-10.,-22.4152849636136,-30.1934595566656));
#48649=CARTESIAN_POINT('Origin',(-10.5,-22.0617315730203,-29.8399061660723));
#48650=CARTESIAN_POINT('',(-10.,-23.4052344572747,-31.1834090503267));
#48651=CARTESIAN_POINT('',(-10.5,-23.0516810666815,-31.53696244092));
#48652=CARTESIAN_POINT('Origin',(-14.,-22.0617315730203,-30.5470129472589));
#48653=CARTESIAN_POINT('',(-6.70710678118655,-21.708178182427,-30.1934595566656));
#48654=CARTESIAN_POINT('',(-14.,-21.708178182427,-30.1934595566656));
#48655=CARTESIAN_POINT('',(-14.,-25.809397513309,-34.2946788875476));
#48656=CARTESIAN_POINT('',(-14.,-25.809397513309,-34.2946788875476));
#48657=CARTESIAN_POINT('',(-14.,-18.031222920257,-26.5165042944955));
#48658=CARTESIAN_POINT('',(-14.,-5.90954544295051,-14.3948268171891));
#48659=CARTESIAN_POINT('',(-6.70710678118654,-18.031222920257,-26.5165042944955));
#48660=CARTESIAN_POINT('',(-14.,-18.031222920257,-26.5165042944955));
#48661=CARTESIAN_POINT('',(-6.70710678118654,-21.5137238176007,-29.9990051918393));
#48662=CARTESIAN_POINT('Origin',(-14.,-26.1629509039023,-33.9411254969543));
#48663=CARTESIAN_POINT('',(-14.,-26.5165042944955,-34.2946788875476));
#48664=CARTESIAN_POINT('',(-14.,-26.5165042944955,-34.2946788875476));
#48665=CARTESIAN_POINT('Origin',(-14.,-26.1629509039023,-33.9411254969543));
#48666=CARTESIAN_POINT('Origin',(-6.5,-20.9177083067616,-28.4029896810001));
#48667=CARTESIAN_POINT('',(-6.01703708685547,-22.0617315730203,-29.7300256491511));
#48668=CARTESIAN_POINT('',(-6.14644660940673,-21.8117315730203,-29.7970129472589));
#48669=CARTESIAN_POINT('Origin',(-6.5,-22.0617315730203,-29.5470129472589));
#48670=CARTESIAN_POINT('',(-6.14644660940673,-18.4276695296637,-26.4129509039022));
#48671=CARTESIAN_POINT('',(-6.14644660940673,-20.6677083067616,-28.6529896810001));
#48672=CARTESIAN_POINT('',(-6.01703708685546,-18.4946568277715,-26.1629509039023));
#48673=CARTESIAN_POINT('Origin',(-6.5,-18.6776695296637,-26.1629509039023));
#48674=CARTESIAN_POINT('',(-6.,-18.6776695296637,-26.1629509039023));
#48675=CARTESIAN_POINT('Origin',(-6.5,-18.6776695296637,-26.1629509039023));
#48676=CARTESIAN_POINT('',(-6.,-22.0617315730203,-29.5470129472589));
#48677=CARTESIAN_POINT('',(-6.,-20.9177083067616,-28.4029896810001));
#48678=CARTESIAN_POINT('Origin',(-6.5,-22.0617315730203,-29.5470129472589));
#48679=CARTESIAN_POINT('Origin',(-5.80473785412436,-19.6609186857656,-26.1629509039022));
#48680=CARTESIAN_POINT('',(-6.35355339059327,-18.1347763108502,-26.4129509039023));
#48681=CARTESIAN_POINT('',(-5.45118446353109,-19.4109186857656,-26.4129509039022));
#48682=CARTESIAN_POINT('',(-6.35355339059327,-18.1347763108502,-25.9129509039023));
#48683=CARTESIAN_POINT('Origin',(-6.70710678118655,-18.3847763108502,-26.1629509039023));
#48684=CARTESIAN_POINT('',(-6.14644660940673,-18.4276695296637,-25.9129509039023));
#48685=CARTESIAN_POINT('',(-5.45118446353109,-19.4109186857656,-25.9129509039023));
#48686=CARTESIAN_POINT('Origin',(-6.5,-18.6776695296637,-26.1629509039022));
#48687=CARTESIAN_POINT('Origin',(-6.25,-21.1424927574778,-29.2742207411231));
#48688=CARTESIAN_POINT('',(-6.35355339059327,-21.8117315730203,-30.0899061660723));
#48689=CARTESIAN_POINT('',(-5.93451779686442,-21.8117315730203,-29.4973003463039));
#48690=CARTESIAN_POINT('',(-6.35355339059327,-21.617277208194,-29.895451801246));
#48691=CARTESIAN_POINT('Origin',(-6.2880711874577,-22.0617315730203,-29.2473003463039));
#48692=CARTESIAN_POINT('',(-6.14644660940672,-22.3117315730203,-29.7970129472588));
#48693=CARTESIAN_POINT('Origin',(-6.5,-22.0617315730203,-29.5470129472589));
#48694=CARTESIAN_POINT('',(-6.35355339059327,-22.3117315730203,-30.0899061660723));
#48695=CARTESIAN_POINT('',(-5.93451779686442,-22.3117315730203,-29.4973003463039));
#48696=CARTESIAN_POINT('Origin',(-6.70710678118654,-22.0617315730203,-29.8399061660723));
#48697=CARTESIAN_POINT('Origin',(-6.70710678118654,-21.867277208194,-29.645451801246));
#48698=CARTESIAN_POINT('Origin',(-6.70710678118654,-22.0617315730203,-29.8399061660723));
#48699=CARTESIAN_POINT('Origin',(-6.70710678118654,-18.3847763108502,-26.1629509039023));
#48700=CARTESIAN_POINT('Origin',(-6.25,-19.97576656852,-24.2184072556392));
#48701=CARTESIAN_POINT('',(-6.35355339059327,-25.9129509039023,-18.1347763108502));
#48702=CARTESIAN_POINT('',(-6.35355339059327,-18.8418830920368,-25.2058441227157));
#48703=CARTESIAN_POINT('',(-6.14644660940673,-25.9129509039023,-18.4276695296637));
#48704=CARTESIAN_POINT('',(-4.69285113019775,-25.9129509039023,-20.4833639705652));
#48705=CARTESIAN_POINT('',(-6.14644660940673,-21.1096500450032,-23.2309703885628));
#48706=CARTESIAN_POINT('Origin',(-6.25,-28.2489159084026,-24.0062752212833));
#48707=CARTESIAN_POINT('',(-6.14644660940672,-30.0250855260513,-22.0836589942278));
#48708=CARTESIAN_POINT('',(-6.14644660940672,-27.1150324319194,-24.9937120883597));
#48709=CARTESIAN_POINT('',(-6.35355339059327,-30.1934595566656,-22.208178182427));
#48710=CARTESIAN_POINT('Origin',(-6.,-29.3399061660723,-22.5617315730203));
#48711=CARTESIAN_POINT('',(-6.35355339059327,-29.3827993848858,-23.0188383542068));
#48712=CARTESIAN_POINT('Origin',(-6.5,-26.8650324319194,-24.7437120883597));
#48713=CARTESIAN_POINT('',(-6.,-29.5470129472589,-22.0617315730203));
#48714=CARTESIAN_POINT('',(-6.,-26.8650324319194,-24.7437120883597));
#48715=CARTESIAN_POINT('',(-6.09270987511341,-29.9571708538506,-22.0617315730203));
#48716=CARTESIAN_POINT('Origin',(-6.5,-29.5470129472589,-22.0617315730203));
#48717=CARTESIAN_POINT('Ctrl Pts',(-6.09270987511341,-29.9571708538506,
-22.0617315730203));
#48718=CARTESIAN_POINT('Ctrl Pts',(-6.10696729553699,-29.9780430792037,
-22.0691748156934));
#48719=CARTESIAN_POINT('Ctrl Pts',(-6.12280773614487,-29.9982570735517,
-22.0759673093509));
#48720=CARTESIAN_POINT('Ctrl Pts',(-6.14208599488146,-30.0202233077774,
-22.0822967086671));
#48721=CARTESIAN_POINT('Ctrl Pts',(-6.14425676103634,-30.0226594227913,
-22.0829881842228));
#48722=CARTESIAN_POINT('Ctrl Pts',(-6.14644660940672,-30.0250855260513,
-22.0836589942278));
#48723=CARTESIAN_POINT('Origin',(-76.5,0.,0.));
#48724=CARTESIAN_POINT('Origin',(-77.,0.,0.));
#48725=CARTESIAN_POINT('Origin',(-77.,23.8767458057638,34.489868218463));
#48726=CARTESIAN_POINT('Origin',(-77.,27.2236110756821,27.2236110756821));
#48727=CARTESIAN_POINT('',(-77.,27.2236110756821,28.9736110756821));
#48728=CARTESIAN_POINT('Origin',(-77.,27.2236110756821,27.2236110756821));
#48729=CARTESIAN_POINT('Origin',(-76.5,27.2236110756821,27.2236110756821));
#48730=CARTESIAN_POINT('',(-76.5,27.2236110756821,28.4736110756821));
#48731=CARTESIAN_POINT('Origin',(-76.5,27.2236110756821,28.9736110756821));
#48732=CARTESIAN_POINT('Origin',(-76.5,27.2236110756821,27.2236110756821));
#48733=CARTESIAN_POINT('Origin',(-83.,27.2236110756821,27.2236110756821));
#48734=CARTESIAN_POINT('',(-67.5,27.2236110756821,28.4736110756821));
#48735=CARTESIAN_POINT('',(-83.,27.2236110756821,28.4736110756821));
#48736=CARTESIAN_POINT('',(-67.5,27.2236110756821,25.9736110756821));
#48737=CARTESIAN_POINT('Origin',(-67.5,27.2236110756821,27.2236110756821));
#48738=CARTESIAN_POINT('Origin',(-67.5,27.2236110756821,27.2236110756821));
#48739=CARTESIAN_POINT('Origin',(-14.,-18.3847763108502,-26.1629509039023));
#48740=CARTESIAN_POINT('',(-6.70710678118654,-18.031222920257,-25.809397513309));
#48741=CARTESIAN_POINT('Origin',(-6.70710678118654,-18.3847763108502,-26.1629509039023));
#48742=CARTESIAN_POINT('',(-14.,-18.031222920257,-25.809397513309));
#48743=CARTESIAN_POINT('Origin',(-14.,-18.3847763108502,-26.1629509039023));
#48744=CARTESIAN_POINT('',(-14.,-18.031222920257,-25.809397513309));
#48745=CARTESIAN_POINT('Origin',(-6.70710678118654,-18.3847763108502,-26.1629509039023));
#48746=CARTESIAN_POINT('Origin',(-6.70710678118654,-18.3847763108502,-26.1629509039023));
#48747=CARTESIAN_POINT('Origin',(-14.,-22.0617315730203,-29.8399061660723));
#48748=CARTESIAN_POINT('',(-6.70710678118655,-22.4152849636136,-30.1934595566656));
#48749=CARTESIAN_POINT('Origin',(-6.70710678118655,-22.0617315730203,-29.8399061660723));
#48750=CARTESIAN_POINT('',(-14.,-22.4152849636136,-30.1934595566656));
#48751=CARTESIAN_POINT('Origin',(-6.70710678118655,-22.0617315730203,-29.8399061660723));
#48752=CARTESIAN_POINT('Origin',(-6.70710678118655,-22.0617315730203,-29.8399061660723));
#48753=CARTESIAN_POINT('Origin',(-6.70710678118654,-19.0918830920368,-25.4558441227157));
#48754=CARTESIAN_POINT('',(-6.70710678118654,-25.809397513309,-18.031222920257));
#48755=CARTESIAN_POINT('',(-6.70710678118654,-18.7383297014435,-25.1022907321224));
#48756=CARTESIAN_POINT('Origin',(-6.70710678118655,-26.1629509039023,-18.3847763108502));
#48757=CARTESIAN_POINT('Origin',(-6.70710678118654,-26.1629509039023,-18.3847763108502));
#48758=CARTESIAN_POINT('',(-6.35355339059327,-26.4129509039023,-18.1347763108502));
#48759=CARTESIAN_POINT('',(-6.70710678118655,-26.5165042944955,-18.031222920257));
#48760=CARTESIAN_POINT('Origin',(-6.70710678118655,-26.1629509039023,-18.3847763108502));
#48761=CARTESIAN_POINT('Origin',(-6.70710678118654,-26.1629509039023,-18.3847763108502));
#48762=CARTESIAN_POINT('Origin',(-6.70710678118654,-26.1629509039023,-18.3847763108502));
#48763=CARTESIAN_POINT('Origin',(-14.,-26.1629509039023,-18.3847763108502));
#48764=CARTESIAN_POINT('',(-14.,-25.809397513309,-18.031222920257));
#48765=CARTESIAN_POINT('',(-14.,-25.809397513309,-18.031222920257));
#48766=CARTESIAN_POINT('',(-14.,-26.5165042944955,-18.031222920257));
#48767=CARTESIAN_POINT('Origin',(-14.,-26.1629509039023,-18.3847763108502));
#48768=CARTESIAN_POINT('',(-14.,-26.5165042944955,-18.031222920257));
#48769=CARTESIAN_POINT('Origin',(-14.,-17.6776695296637,-26.1629509039023));
#48770=CARTESIAN_POINT('',(-14.,-16.7989898732233,-27.0416305603426));
#48771=CARTESIAN_POINT('Origin',(-6.5,-21.3596500450032,-23.4809703885628));
#48772=CARTESIAN_POINT('',(-6.,-26.1629509039023,-18.6776695296637));
#48773=CARTESIAN_POINT('Origin',(-6.5,-26.1629509039023,-18.6776695296637));
#48774=CARTESIAN_POINT('',(-6.,-21.3596500450032,-23.4809703885628));
#48775=CARTESIAN_POINT('Origin',(-5.04640452079102,-26.1629509039023,-20.7333639705652));
#48776=CARTESIAN_POINT('',(-6.14644660940673,-26.4129509039023,-18.4276695296637));
#48777=CARTESIAN_POINT('',(-4.69285113019775,-26.4129509039023,-20.4833639705652));
#48778=CARTESIAN_POINT('Origin',(-6.5,-26.1629509039023,-18.6776695296637));
#48779=CARTESIAN_POINT('Origin',(-6.5,-26.1629509039023,-18.6776695296637));
#48780=CARTESIAN_POINT('Origin',(-6.5,-26.1629509039023,-18.6776695296637));
#48781=CARTESIAN_POINT('Origin',(-6.,-24.1123412384613,-24.1123412384613));
#48782=CARTESIAN_POINT('',(-6.,-27.306974170161,-19.8216927959224));
#48783=CARTESIAN_POINT('Origin',(-6.5,-27.306974170161,-19.8216927959224));
#48784=CARTESIAN_POINT('',(-6.14644660940673,-29.9434595566656,-21.958178182427));
#48785=CARTESIAN_POINT('',(-6.14644660940673,-27.556974170161,-19.5716927959224));
#48786=CARTESIAN_POINT('Origin',(-6.5,-29.6934595566656,-22.208178182427));
#48787=CARTESIAN_POINT('Origin',(-6.25,-27.0821897194448,-18.9504617357995));
#48788=CARTESIAN_POINT('',(-6.35355339059327,-30.0899061660723,-21.8117315730203));
#48789=CARTESIAN_POINT('',(-6.35355339059327,-26.6074052687286,-18.3292306756765));
#48790=CARTESIAN_POINT('',(-10.25,-32.8451099861151,-19.0565277529775));
#48791=CARTESIAN_POINT('Origin',(-73.,0.,0.));
#48792=CARTESIAN_POINT('',(-73.,-44.,5.38844591624836E-15));
#48793=CARTESIAN_POINT('',(-73.,-5.38844591624836E-15,44.));
#48794=CARTESIAN_POINT('Origin',(-73.,0.,0.));
#48795=CARTESIAN_POINT('',(-73.5,-5.32721357629099E-15,43.5));
#48796=CARTESIAN_POINT('Origin',(-73.,-5.32721357629099E-15,43.5));
#48797=CARTESIAN_POINT('Origin',(-73.5,0.,0.));
#48798=CARTESIAN_POINT('Origin',(-73.,0.,0.));
#48799=CARTESIAN_POINT('Origin',(-75.,0.,0.));
#48800=CARTESIAN_POINT('',(-68.0071067811866,-44.,-5.38844591624836E-15));
#48801=CARTESIAN_POINT('',(-68.0071067811866,-5.38844591624836E-15,44.));
#48802=CARTESIAN_POINT('Origin',(-68.0071067811866,0.,0.));
#48803=CARTESIAN_POINT('',(-75.,-44.,-5.38844591624836E-15));
#48804=CARTESIAN_POINT('Origin',(-68.0071067811866,0.,0.));
#48805=CARTESIAN_POINT('Origin',(-73.5,42.4,0.));
#48806=CARTESIAN_POINT('',(-73.5,-42.4,-5.19250242838478E-15));
#48807=CARTESIAN_POINT('Origin',(-73.5,0.,0.));
#48808=CARTESIAN_POINT('Origin',(-68.0071067811866,0.,0.));
#48809=CARTESIAN_POINT('',(-67.6535533905933,-5.37051137910276E-15,43.8535533905933));
#48810=CARTESIAN_POINT('',(-67.6535533905933,-43.8535533905933,-5.37051137910276E-15));
#48811=CARTESIAN_POINT('Origin',(-67.6535533905933,0.,-6.71313922387845E-15));
#48812=CARTESIAN_POINT('Origin',(-67.6535533905933,0.,-6.71313922387845E-15));
#48813=CARTESIAN_POINT('Origin',(-68.0071067811866,-5.32721357629099E-15,
43.5));
#48814=CARTESIAN_POINT('Origin',(-67.4,0.,0.));
#48815=CARTESIAN_POINT('',(-67.1464466094067,-43.3464466094067,-5.30840870946216E-15));
#48816=CARTESIAN_POINT('',(-67.1464466094067,-5.30840870946216E-15,43.3464466094067));
#48817=CARTESIAN_POINT('Origin',(-67.1464466094067,0.,-6.6355108868277E-15));
#48818=CARTESIAN_POINT('',(-67.4,-43.6,-5.33946004428246E-15));
#48819=CARTESIAN_POINT('Origin',(-67.1464466094067,0.,-6.6355108868277E-15));
#48820=CARTESIAN_POINT('Origin',(-76.5,0.,0.));
#48821=CARTESIAN_POINT('Origin',(-77.,0.,0.));
#48822=CARTESIAN_POINT('Origin',(-77.,-34.489868218463,23.8767458057638));
#48823=CARTESIAN_POINT('Origin',(-77.,-27.2236110756821,27.2236110756821));
#48824=CARTESIAN_POINT('',(-77.,-27.2236110756821,28.9736110756821));
#48825=CARTESIAN_POINT('Origin',(-77.,-27.2236110756821,27.2236110756821));
#48826=CARTESIAN_POINT('Origin',(-76.5,0.,0.));
#48827=CARTESIAN_POINT('Origin',(-77.,0.,0.));
#48828=CARTESIAN_POINT('Origin',(-77.,34.489868218463,-23.8767458057638));
#48829=CARTESIAN_POINT('',(-77.,27.2236110756821,-25.4736110756821));
#48830=CARTESIAN_POINT('Origin',(-77.,27.2236110756821,-27.2236110756821));
#48831=CARTESIAN_POINT('Origin',(-10.6035533905933,-32.5951099861151,-19.3065277529775));
#48832=CARTESIAN_POINT('',(-6.70710678118655,-30.1934595566656,-22.4152849636136));
#48833=CARTESIAN_POINT('Origin',(-6.70710678118655,-29.8399061660723,-22.0617315730203));
#48834=CARTESIAN_POINT('Origin',(-6.70710678118655,-29.8399061660723,-22.0617315730203));
#48835=CARTESIAN_POINT('Origin',(-6.70710678118655,-29.1327993848858,-22.7688383542068));
#48836=CARTESIAN_POINT('',(-6.70710678118655,-29.486352775479,-23.1223917448001));
#48837=CARTESIAN_POINT('Origin',(-14.,-30.5470129472589,-22.0617315730203));
#48838=CARTESIAN_POINT('',(-10.,-30.1934595566656,-22.4152849636136));
#48839=CARTESIAN_POINT('',(-14.,-30.1934595566656,-22.4152849636136));
#48840=CARTESIAN_POINT('',(-10.,-28.4256926036992,-24.1830519165799));
#48841=CARTESIAN_POINT('Origin',(-6.70710678118655,-26.3574052687286,-18.5792306756765));
#48842=CARTESIAN_POINT('',(-6.70710678118655,-30.1934595566656,-21.708178182427));
#48843=CARTESIAN_POINT('',(-6.70710678118655,-26.7109586593218,-18.2256772850833));
#48844=CARTESIAN_POINT('Origin',(-6.70710678118655,-29.8399061660723,-22.0617315730203));
#48845=CARTESIAN_POINT('Origin',(-6.70710678118655,-29.8399061660723,-22.0617315730203));
#48846=CARTESIAN_POINT('Origin',(-6.70710678118655,-29.8399061660723,-22.0617315730203));
#48847=CARTESIAN_POINT('Origin',(-14.,-26.1629509039023,-17.6776695296637));
#48848=CARTESIAN_POINT('',(-14.,-34.2946788875476,-25.809397513309));
#48849=CARTESIAN_POINT('',(-14.,-12.2027957955108,-3.7175144212722));
#48850=CARTESIAN_POINT('',(-10.5,-34.2946788875476,-25.809397513309));
#48851=CARTESIAN_POINT('',(-14.,-34.2946788875476,-25.809397513309));
#48852=CARTESIAN_POINT('',(-10.5,-30.1934595566656,-21.708178182427));
#48853=CARTESIAN_POINT('',(-10.5,-29.3449314192417,-20.8596500450031));
#48854=CARTESIAN_POINT('',(-14.,-30.1934595566656,-21.708178182427));
#48855=CARTESIAN_POINT('Origin',(-14.,-29.8399061660723,-22.0617315730203));
#48856=CARTESIAN_POINT('Origin',(-10.5,-29.8399061660723,-22.0617315730203));
#48857=CARTESIAN_POINT('Origin',(-76.5,27.2236110756821,-27.2236110756821));
#48858=CARTESIAN_POINT('',(-76.5,27.2236110756821,-25.9736110756821));
#48859=CARTESIAN_POINT('Origin',(-76.5,27.2236110756821,-25.4736110756821));
#48860=CARTESIAN_POINT('Origin',(-76.5,27.2236110756821,-27.2236110756821));
#48861=CARTESIAN_POINT('Origin',(-83.,27.2236110756821,-27.2236110756821));
#48862=CARTESIAN_POINT('',(-67.5,27.2236110756821,-25.9736110756821));
#48863=CARTESIAN_POINT('',(-83.,27.2236110756821,-25.9736110756821));
#48864=CARTESIAN_POINT('',(-67.5,27.2236110756821,-28.4736110756821));
#48865=CARTESIAN_POINT('Origin',(-67.5,27.2236110756821,-27.2236110756821));
#48866=CARTESIAN_POINT('Origin',(-67.5,27.2236110756821,-27.2236110756821));
#48867=CARTESIAN_POINT('Origin',(-76.5,-27.2236110756821,27.2236110756821));
#48868=CARTESIAN_POINT('',(-76.5,-27.2236110756821,28.4736110756821));
#48869=CARTESIAN_POINT('Origin',(-76.5,-27.2236110756821,28.9736110756821));
#48870=CARTESIAN_POINT('Origin',(-76.5,-27.2236110756821,27.2236110756821));
#48871=CARTESIAN_POINT('Origin',(-83.,-27.2236110756821,27.2236110756821));
#48872=CARTESIAN_POINT('',(-67.5,-27.2236110756821,28.4736110756821));
#48873=CARTESIAN_POINT('',(-83.,-27.2236110756821,28.4736110756821));
#48874=CARTESIAN_POINT('',(-67.5,-27.2236110756821,25.9736110756821));
#48875=CARTESIAN_POINT('Origin',(-67.5,-27.2236110756821,27.2236110756821));
#48876=CARTESIAN_POINT('Origin',(-67.5,-27.2236110756821,27.2236110756821));
#48877=CARTESIAN_POINT('Origin',(-67.5,-12.5,21.650635094611));
#48878=CARTESIAN_POINT('',(-67.,-12.5,18.150635094611));
#48879=CARTESIAN_POINT('Origin',(-67.,-12.5,21.650635094611));
#48880=CARTESIAN_POINT('',(-67.5,-12.5,18.650635094611));
#48881=CARTESIAN_POINT('Origin',(-67.5,-12.5,18.150635094611));
#48882=CARTESIAN_POINT('',(-67.5,-12.5,24.650635094611));
#48883=CARTESIAN_POINT('Origin',(-67.5,-12.5,21.650635094611));
#48884=CARTESIAN_POINT('Origin',(-67.5,-12.5,21.650635094611));
#48885=CARTESIAN_POINT('Origin',(-67.,7.05,0.));
#48886=CARTESIAN_POINT('',(-67.,-5.26511090665038E-15,42.9928932188134));
#48887=CARTESIAN_POINT('Origin',(-67.,0.,0.));
#48888=CARTESIAN_POINT('',(-67.,-12.5,-25.150635094611));
#48889=CARTESIAN_POINT('Origin',(-67.,-12.5,-21.650635094611));
#48890=CARTESIAN_POINT('',(-67.,27.2236110756821,25.4736110756821));
#48891=CARTESIAN_POINT('Origin',(-67.,27.2236110756821,27.2236110756821));
#48892=CARTESIAN_POINT('',(-67.,25.,-3.5));
#48893=CARTESIAN_POINT('Origin',(-67.,25.,0.));
#48894=CARTESIAN_POINT('',(-67.,27.2236110756821,-28.9736110756821));
#48895=CARTESIAN_POINT('Origin',(-67.,27.2236110756821,-27.2236110756821));
#48896=CARTESIAN_POINT('',(-67.,12.,-16.2846096908265));
#48897=CARTESIAN_POINT('Origin',(-67.,12.,-20.7846096908265));
#48898=CARTESIAN_POINT('',(-67.,-24.,4.5));
#48899=CARTESIAN_POINT('Origin',(-67.,-24.,2.93915231795365E-15));
#48900=CARTESIAN_POINT('',(-67.,12.,25.2846096908265));
#48901=CARTESIAN_POINT('Origin',(-67.,12.,20.7846096908265));
#48902=CARTESIAN_POINT('',(-67.,-9.24608333356252E-16,7.55));
#48903=CARTESIAN_POINT('Origin',(-67.,0.,0.));
#48904=CARTESIAN_POINT('',(-67.,-27.2236110756821,25.4736110756821));
#48905=CARTESIAN_POINT('Origin',(-67.,-27.2236110756821,27.2236110756821));
#48906=CARTESIAN_POINT('',(-67.,-27.2236110756821,-28.9736110756821));
#48907=CARTESIAN_POINT('Origin',(-67.,-27.2236110756821,-27.2236110756821));
#48908=CARTESIAN_POINT('Origin',(-80.,-12.5,21.650635094611));
#48909=CARTESIAN_POINT('',(-80.,-12.5,24.650635094611));
#48910=CARTESIAN_POINT('Origin',(-80.,-12.5,21.650635094611));
#48911=CARTESIAN_POINT('',(-80.,-12.5,24.650635094611));
#48912=CARTESIAN_POINT('Origin',(-67.5,-12.5,-21.650635094611));
#48913=CARTESIAN_POINT('',(-67.5,-12.5,-24.650635094611));
#48914=CARTESIAN_POINT('Origin',(-67.5,-12.5,-25.150635094611));
#48915=CARTESIAN_POINT('',(-67.5,-12.5,-18.650635094611));
#48916=CARTESIAN_POINT('Origin',(-67.5,-12.5,-21.650635094611));
#48917=CARTESIAN_POINT('Origin',(-67.5,-12.5,-21.650635094611));
#48918=CARTESIAN_POINT('Origin',(-80.,-12.5,-21.650635094611));
#48919=CARTESIAN_POINT('',(-80.,-12.5,-18.650635094611));
#48920=CARTESIAN_POINT('Origin',(-80.,-12.5,-21.650635094611));
#48921=CARTESIAN_POINT('',(-80.,-12.5,-18.650635094611));
#48922=CARTESIAN_POINT('Origin',(-67.5,0.,0.));
#48923=CARTESIAN_POINT('Origin',(-67.5,-5.26511090665038E-15,42.9928932188134));
#48924=CARTESIAN_POINT('Origin',(-67.5,27.2236110756821,27.2236110756821));
#48925=CARTESIAN_POINT('Origin',(-67.5,27.2236110756821,25.4736110756821));
#48926=CARTESIAN_POINT('Origin',(-67.5,-27.2236110756821,-27.2236110756821));
#48927=CARTESIAN_POINT('Origin',(-67.5,-27.2236110756821,-28.9736110756821));
#48928=CARTESIAN_POINT('Origin',(-67.5,25.,0.));
#48929=CARTESIAN_POINT('',(-67.5,25.,-3.));
#48930=CARTESIAN_POINT('Origin',(-67.5,25.,-3.5));
#48931=CARTESIAN_POINT('',(-67.5,25.,3.));
#48932=CARTESIAN_POINT('Origin',(-67.5,25.,0.));
#48933=CARTESIAN_POINT('Origin',(-67.5,25.,0.));
#48934=CARTESIAN_POINT('Origin',(-80.,25.,0.));
#48935=CARTESIAN_POINT('',(-80.,25.,3.));
#48936=CARTESIAN_POINT('Origin',(-80.,25.,0.));
#48937=CARTESIAN_POINT('',(-80.,25.,3.));
#48938=CARTESIAN_POINT('Origin',(-67.5,-27.2236110756821,27.2236110756821));
#48939=CARTESIAN_POINT('Origin',(-67.5,-27.2236110756821,25.4736110756821));
#48940=CARTESIAN_POINT('Origin',(-67.5,27.2236110756821,-27.2236110756821));
#48941=CARTESIAN_POINT('Origin',(-67.5,27.2236110756821,-28.9736110756821));
#48942=CARTESIAN_POINT('Origin',(-16.,25.,0.));
#48943=CARTESIAN_POINT('',(-16.,25.,3.));
#48944=CARTESIAN_POINT('Origin',(-16.,25.,0.));
#48945=CARTESIAN_POINT('',(-15.5,25.,3.5));
#48946=CARTESIAN_POINT('Origin',(-16.,25.,3.5));
#48947=CARTESIAN_POINT('Origin',(-15.5,25.,0.));
#48948=CARTESIAN_POINT('Origin',(-80.,25.,0.));
#48949=CARTESIAN_POINT('',(-19.5,25.,3.));
#48950=CARTESIAN_POINT('Origin',(-19.5,25.,0.));
#48951=CARTESIAN_POINT('',(-80.,25.,3.));
#48952=CARTESIAN_POINT('Origin',(-15.5,25.,0.));
#48953=CARTESIAN_POINT('',(-15.5,25.,5.));
#48954=CARTESIAN_POINT('Origin',(-15.5,25.,0.));
#48955=CARTESIAN_POINT('Origin',(-16.,-12.5,21.650635094611));
#48956=CARTESIAN_POINT('',(-16.,-12.5,24.650635094611));
#48957=CARTESIAN_POINT('Origin',(-16.,-12.5,21.650635094611));
#48958=CARTESIAN_POINT('',(-15.5,-12.5,25.150635094611));
#48959=CARTESIAN_POINT('Origin',(-16.,-12.5,25.150635094611));
#48960=CARTESIAN_POINT('Origin',(-15.5,-12.5,21.650635094611));
#48961=CARTESIAN_POINT('Origin',(-80.,-12.5,21.650635094611));
#48962=CARTESIAN_POINT('',(-19.5,-12.5,24.650635094611));
#48963=CARTESIAN_POINT('Origin',(-19.5,-12.5,21.650635094611));
#48964=CARTESIAN_POINT('',(-80.,-12.5,24.650635094611));
#48965=CARTESIAN_POINT('Origin',(-15.5,-12.5,21.650635094611));
#48966=CARTESIAN_POINT('',(-15.5,-12.5,26.650635094611));
#48967=CARTESIAN_POINT('Origin',(-15.5,-12.5,21.650635094611));
#48968=CARTESIAN_POINT('Origin',(-16.,-12.5,-21.650635094611));
#48969=CARTESIAN_POINT('',(-16.,-12.5,-18.650635094611));
#48970=CARTESIAN_POINT('Origin',(-16.,-12.5,-21.650635094611));
#48971=CARTESIAN_POINT('',(-15.5,-12.5,-18.150635094611));
#48972=CARTESIAN_POINT('Origin',(-16.,-12.5,-18.150635094611));
#48973=CARTESIAN_POINT('Origin',(-15.5,-12.5,-21.650635094611));
#48974=CARTESIAN_POINT('Origin',(-80.,-12.5,-21.650635094611));
#48975=CARTESIAN_POINT('',(-19.5,-12.5,-18.650635094611));
#48976=CARTESIAN_POINT('Origin',(-19.5,-12.5,-21.650635094611));
#48977=CARTESIAN_POINT('',(-80.,-12.5,-18.650635094611));
#48978=CARTESIAN_POINT('Origin',(-15.5,-12.5,-21.650635094611));
#48979=CARTESIAN_POINT('',(-15.5,-12.5,-16.650635094611));
#48980=CARTESIAN_POINT('Origin',(-15.5,-12.5,-21.650635094611));
#48981=CARTESIAN_POINT('Origin',(-10.5,-32.1733585439879,-27.9307178568686));
#48982=CARTESIAN_POINT('',(-10.,-33.9411254969543,-26.1629509039023));
#48983=CARTESIAN_POINT('',(-10.,-32.1733585439879,-27.9307178568686));
#48984=CARTESIAN_POINT('',(-10.5,-34.2946788875476,-26.5165042944955));
#48985=CARTESIAN_POINT('Origin',(-10.5,-33.9411254969543,-26.1629509039023));
#48986=CARTESIAN_POINT('',(-10.5,-32.5269119345812,-28.2842712474619));
#48987=CARTESIAN_POINT('Origin',(-10.5,-28.9913780286485,-21.2132034355964));
#48988=CARTESIAN_POINT('Origin',(-10.5,-33.9411254969543,-26.1629509039023));
#48989=CARTESIAN_POINT('',(-10.,-28.9913780286485,-21.2132034355964));
#48990=CARTESIAN_POINT('Origin',(-10.5,-33.9411254969543,-26.1629509039023));
#48991=CARTESIAN_POINT('Origin',(-10.5,-33.9411254969543,-26.1629509039023));
#48992=CARTESIAN_POINT('Origin',(-14.,-34.6482322781408,-26.1629509039023));
#48993=CARTESIAN_POINT('',(-14.,-26.2486696528563,-34.5625135291868));
#48994=CARTESIAN_POINT('',(-14.,-29.5269119345812,-31.2842712474619));
#48995=CARTESIAN_POINT('',(-14.025428935758,-34.2946788875476,-26.5165042944955));
#48996=CARTESIAN_POINT('',(-14.,-34.2946788875476,-26.5165042944955));
#48997=CARTESIAN_POINT('',(-14.,-33.2888210834328,-27.5223620986103));
#48998=CARTESIAN_POINT('Ctrl Pts',(-14.025428935758,-34.2946788875476,-26.5165042944955));
#48999=CARTESIAN_POINT('Ctrl Pts',(-14.0048893955981,-33.9495862335655,
-26.8615969484776));
#49000=CARTESIAN_POINT('Ctrl Pts',(-14.,-33.6061320240591,-27.205051157984));
#49001=CARTESIAN_POINT('Ctrl Pts',(-14.,-33.2888210834328,-27.5223620986103));
#49002=CARTESIAN_POINT('',(-14.,-27.5223620986103,-33.2888210834328));
#49003=CARTESIAN_POINT('',(-14.,-29.5269119345812,-31.2842712474619));
#49004=CARTESIAN_POINT('',(-14.1464466094067,-25.5428242561643,-35.2683589258788));
#49005=CARTESIAN_POINT('Ctrl Pts',(-14.,-27.5223620986103,-33.2888210834328));
#49006=CARTESIAN_POINT('Ctrl Pts',(-14.,-27.1477600534413,-33.6634231286018));
#49007=CARTESIAN_POINT('Ctrl Pts',(-14.006470104281,-26.7367117564975,-34.0744714255456));
#49008=CARTESIAN_POINT('Ctrl Pts',(-14.0541139337517,-26.1259981746158,
-34.6851850074273));
#49009=CARTESIAN_POINT('Ctrl Pts',(-14.0762586162872,-25.9236817936235,
-34.8875013884196));
#49010=CARTESIAN_POINT('Ctrl Pts',(-14.1209183378663,-25.6651436792899,
-35.1460395027532));
#49011=CARTESIAN_POINT('Ctrl Pts',(-14.1328725146262,-25.6036027751564,
-35.2075804068867));
#49012=CARTESIAN_POINT('Ctrl Pts',(-14.1464466094065,-25.5428242561655,
-35.2683589258776));
#49013=CARTESIAN_POINT('Ctrl Pts',(-14.1464466094067,-25.5428242561643,
-35.2683589258788));
#49014=CARTESIAN_POINT('Ctrl Pts',(-14.0674931369572,-25.8963413932067,
-34.9148417888364));
#49015=CARTESIAN_POINT('Ctrl Pts',(-14.,-26.2486696528563,-34.5625135291868));
#49016=CARTESIAN_POINT('Origin',(-14.,-33.9411254969543,-26.1629509039023));
#49017=CARTESIAN_POINT('',(-14.,-34.4335120598975,-26.0760286821578));
#49018=CARTESIAN_POINT('Origin',(-14.,-33.9411254969543,-26.1629509039023));
#49019=CARTESIAN_POINT('Ctrl Pts',(-14.0254289357581,-34.2946788875476,
-26.5165042944955));
#49020=CARTESIAN_POINT('Ctrl Pts',(-14.0263293530702,-34.3098071424901,
-26.501376039553));
#49021=CARTESIAN_POINT('Ctrl Pts',(-14.0268044276371,-34.3239877839475,
-26.4852549680463));
#49022=CARTESIAN_POINT('Ctrl Pts',(-14.0268044276371,-34.3371305955528,
-26.4682048340719));
#49023=CARTESIAN_POINT('Ctrl Pts',(-14.0268044276371,-34.3619967163995,
-26.4359460827031));
#49024=CARTESIAN_POINT('Ctrl Pts',(-14.0250516964297,-34.3827322393151,
-26.4009212026149));
#49025=CARTESIAN_POINT('Ctrl Pts',(-14.0179720411043,-34.4215374836554,
-26.3124348467826));
#49026=CARTESIAN_POINT('Ctrl Pts',(-14.0115803121848,-34.4352140696344,
-26.2577402477615));
#49027=CARTESIAN_POINT('Ctrl Pts',(-14.0028573458318,-34.4429028780862,
-26.1599875313315));
#49028=CARTESIAN_POINT('Ctrl Pts',(-14.,-34.4408500788191,-26.1175962104965));
#49029=CARTESIAN_POINT('Ctrl Pts',(-14.,-34.4335120598975,-26.0760286821578));
#49030=CARTESIAN_POINT('Origin',(-19.1928932188134,0.,0.));
#49031=CARTESIAN_POINT('',(-19.1928932188134,-5.38844591624836E-15,44.));
#49032=CARTESIAN_POINT('',(-19.1928932188134,-44.,-5.38844591624836E-15));
#49033=CARTESIAN_POINT('Origin',(-19.1928932188134,0.,0.));
#49034=CARTESIAN_POINT('Origin',(-19.1928932188134,0.,0.));
#49035=CARTESIAN_POINT('',(-19.5464466094067,-5.37051137910276E-15,43.8535533905933));
#49036=CARTESIAN_POINT('Origin',(-19.1928932188134,-5.32721357629099E-15,
43.5));
#49037=CARTESIAN_POINT('',(-19.5464466094067,-43.8535533905933,-5.37051137910276E-15));
#49038=CARTESIAN_POINT('Origin',(-19.5464466094067,0.,-6.71313922387845E-15));
#49039=CARTESIAN_POINT('Origin',(-19.5464466094067,0.,-6.71313922387845E-15));
#49040=CARTESIAN_POINT('Origin',(-19.7,0.,0.));
#49041=CARTESIAN_POINT('',(-19.8535533905933,-43.5464466094067,-5.33290164544511E-15));
#49042=CARTESIAN_POINT('',(-19.7,-43.7,-5.35170651227393E-15));
#49043=CARTESIAN_POINT('',(-19.8535533905933,-5.3329016454451E-15,43.5464466094067));
#49044=CARTESIAN_POINT('Origin',(-19.8535533905933,0.,-6.66612705680638E-15));
#49045=CARTESIAN_POINT('Origin',(-19.8535533905933,0.,-6.66612705680638E-15));
#49046=CARTESIAN_POINT('Origin',(-17.,0.,0.));
#49047=CARTESIAN_POINT('',(-14.8071067811865,-44.,-5.38844591624836E-15));
#49048=CARTESIAN_POINT('',(-14.8071067811865,-5.38844591624836E-15,44.));
#49049=CARTESIAN_POINT('Origin',(-14.8071067811865,0.,0.));
#49050=CARTESIAN_POINT('',(-17.,-44.,-5.38844591624836E-15));
#49051=CARTESIAN_POINT('Origin',(-14.8071067811865,0.,0.));
#49052=CARTESIAN_POINT('Origin',(-19.5,0.,0.));
#49053=CARTESIAN_POINT('',(-20.,-5.28960384263333E-15,43.1928932188135));
#49054=CARTESIAN_POINT('Origin',(-19.5,-5.28960384263333E-15,43.1928932188135));
#49055=CARTESIAN_POINT('Origin',(-20.,0.,0.));
#49056=CARTESIAN_POINT('Origin',(-20.,43.4,0.));
#49057=CARTESIAN_POINT('',(-20.,-12.5,-18.150635094611));
#49058=CARTESIAN_POINT('Origin',(-20.,-12.5,-21.650635094611));
#49059=CARTESIAN_POINT('',(-20.,25.,3.5));
#49060=CARTESIAN_POINT('Origin',(-20.,25.,0.));
#49061=CARTESIAN_POINT('',(-20.,12.,-16.2846096908265));
#49062=CARTESIAN_POINT('Origin',(-20.,12.,-20.7846096908265));
#49063=CARTESIAN_POINT('',(-20.,-24.,4.5));
#49064=CARTESIAN_POINT('Origin',(-20.,-24.,2.93915231795365E-15));
#49065=CARTESIAN_POINT('',(-20.,12.,25.2846096908265));
#49066=CARTESIAN_POINT('Origin',(-20.,12.,20.7846096908265));
#49067=CARTESIAN_POINT('',(-20.,-1.53080849893419E-15,12.5));
#49068=CARTESIAN_POINT('Origin',(-20.,0.,0.));
#49069=CARTESIAN_POINT('',(-20.,-12.5,25.150635094611));
#49070=CARTESIAN_POINT('Origin',(-20.,-12.5,21.650635094611));
#49071=CARTESIAN_POINT('Origin',(-19.5,-12.5,-21.650635094611));
#49072=CARTESIAN_POINT('Origin',(-19.5,-12.5,-18.150635094611));
#49073=CARTESIAN_POINT('Origin',(-19.5,-12.5,21.650635094611));
#49074=CARTESIAN_POINT('Origin',(-19.5,-12.5,25.150635094611));
#49075=CARTESIAN_POINT('Origin',(-19.5,25.,0.));
#49076=CARTESIAN_POINT('Origin',(-19.5,25.,3.5));
#49077=CARTESIAN_POINT('Origin',(-67.5,0.,0.));
#49078=CARTESIAN_POINT('',(-67.5,-8.63375993398884E-16,7.05));
#49079=CARTESIAN_POINT('',(-67.5,-7.05,-8.63375993398884E-16));
#49080=CARTESIAN_POINT('Origin',(-67.5,0.,0.));
#49081=CARTESIAN_POINT('Origin',(-67.5,0.,0.));
#49082=CARTESIAN_POINT('Origin',(-67.5,-9.24608333356252E-16,7.55));
#49083=CARTESIAN_POINT('Origin',(-75.,0.,0.));
#49084=CARTESIAN_POINT('',(-82.2928932188135,-7.05,-8.63375993398884E-16));
#49085=CARTESIAN_POINT('',(-75.,-7.05,-8.63375993398884E-16));
#49086=CARTESIAN_POINT('',(-82.2928932188135,-8.63375993398884E-16,7.05));
#49087=CARTESIAN_POINT('Origin',(-82.2928932188135,0.,0.));
#49088=CARTESIAN_POINT('Origin',(-82.2928932188135,0.,0.));
#49089=CARTESIAN_POINT('Origin',(-82.5,0.,0.));
#49090=CARTESIAN_POINT('',(-82.8535533905933,7.40355339059327,0.));
#49091=CARTESIAN_POINT('',(-82.8535533905933,-9.06673796210658E-16,-7.40355339059327));
#49092=CARTESIAN_POINT('Origin',(-82.8535533905933,0.,-4.53336898105329E-16));
#49093=CARTESIAN_POINT('Origin',(-82.5,-9.49971599022433E-16,-7.75710678118654));
#49094=CARTESIAN_POINT('Origin',(-82.8535533905933,0.,-4.53336898105329E-16));
#49095=CARTESIAN_POINT('Origin',(-82.75,0.,0.));
#49096=CARTESIAN_POINT('',(-82.6464466094067,7.19644660940673,-1.76262106108895E-15));
#49097=CARTESIAN_POINT('',(-82.75,7.3,-8.93992163377568E-16));
#49098=CARTESIAN_POINT('',(-82.6464466094068,-8.81310530544477E-16,7.19644660940673));
#49099=CARTESIAN_POINT('Origin',(-82.6464466094067,0.,-4.40655265272239E-16));
#49100=CARTESIAN_POINT('Origin',(-82.6464466094067,0.,-4.40655265272239E-16));
#49101=CARTESIAN_POINT('Origin',(-82.2928932188135,0.,0.));
#49102=CARTESIAN_POINT('Origin',(-82.2928932188135,-9.24608333356252E-16,
7.55));
#49103=CARTESIAN_POINT('Origin',(-19.5,0.,0.));
#49104=CARTESIAN_POINT('',(-19.5,-1.46957615897682E-15,12.));
#49105=CARTESIAN_POINT('Origin',(-19.5,-1.53080849893419E-15,12.5));
#49106=CARTESIAN_POINT('',(-19.5,-12.,-1.46957615897682E-15));
#49107=CARTESIAN_POINT('Origin',(-19.5,0.,0.));
#49108=CARTESIAN_POINT('Origin',(-19.5,0.,0.));
#49109=CARTESIAN_POINT('Origin',(-17.,0.,0.));
#49110=CARTESIAN_POINT('',(-14.7071067811865,-12.,-1.46957615897682E-15));
#49111=CARTESIAN_POINT('',(-14.7071067811865,-1.46957615897682E-15,-12.));
#49112=CARTESIAN_POINT('Origin',(-14.7071067811865,0.,0.));
#49113=CARTESIAN_POINT('',(-17.,-12.,-1.46957615897682E-15));
#49114=CARTESIAN_POINT('Origin',(-14.7071067811865,0.,0.));
#49115=CARTESIAN_POINT('Origin',(-14.8071067811865,0.,0.));
#49116=CARTESIAN_POINT('',(-14.4535533905933,-5.37051137910276E-15,43.8535533905933));
#49117=CARTESIAN_POINT('',(-14.4535533905933,-43.8535533905933,-5.37051137910276E-15));
#49118=CARTESIAN_POINT('Origin',(-14.4535533905933,0.,-6.71313922387845E-15));
#49119=CARTESIAN_POINT('Origin',(-14.4535533905933,0.,-6.71313922387845E-15));
#49120=CARTESIAN_POINT('Origin',(-14.8071067811865,-5.32721357629099E-15,
43.5));
#49121=CARTESIAN_POINT('Origin',(-14.3,0.,0.));
#49122=CARTESIAN_POINT('',(-14.1464466094067,-43.5464466094067,-5.33290164544511E-15));
#49123=CARTESIAN_POINT('Origin',(-14.1464466094067,0.,4.44089209850063E-15));
#49124=CARTESIAN_POINT('',(-14.3,-43.7,-5.35170651227393E-15));
#49125=CARTESIAN_POINT('',(-14.1464466094067,25.5428242561642,-35.2683589258789));
#49126=CARTESIAN_POINT('Origin',(-14.1464466094067,0.,4.44089209850063E-15));
#49127=CARTESIAN_POINT('',(-14.,26.2486696528562,-34.5625135291869));
#49128=CARTESIAN_POINT('Ctrl Pts',(-14.,26.2486696528562,-34.5625135291869));
#49129=CARTESIAN_POINT('Ctrl Pts',(-14.0674931369565,25.8963413932104,-34.9148417888327));
#49130=CARTESIAN_POINT('Ctrl Pts',(-14.1464466094067,25.5428242561642,-35.2683589258789));
#49131=CARTESIAN_POINT('Origin',(-14.,0.,0.));
#49132=CARTESIAN_POINT('Origin',(-14.5,0.,0.));
#49133=CARTESIAN_POINT('Origin',(-14.,0.,0.));
#49134=CARTESIAN_POINT('Origin',(-14.,0.,0.));
#49135=CARTESIAN_POINT('Origin',(-14.,0.,0.));
#49136=CARTESIAN_POINT('Origin',(-14.,0.,0.));
#49137=CARTESIAN_POINT('Origin',(-14.,0.,0.));
#49138=CARTESIAN_POINT('',(-14.,33.2888210834329,-27.5223620986102));
#49139=CARTESIAN_POINT('Ctrl Pts',(-14.,33.2888210834329,-27.5223620986102));
#49140=CARTESIAN_POINT('Ctrl Pts',(-14.,33.6061320240592,-27.2050511579839));
#49141=CARTESIAN_POINT('Ctrl Pts',(-14.0048893955981,33.9495862335655,-26.8615969484775));
#49142=CARTESIAN_POINT('Ctrl Pts',(-14.025428935758,34.2946788875476,-26.5165042944955));
#49143=CARTESIAN_POINT('',(-14.,27.5223620986102,-33.2888210834329));
#49144=CARTESIAN_POINT('Origin',(-14.,0.,0.));
#49145=CARTESIAN_POINT('Ctrl Pts',(-14.1464466094073,25.5428242561618,-35.2683589258813));
#49146=CARTESIAN_POINT('Ctrl Pts',(-14.1328725146267,25.6036027751539,-35.2075804068892));
#49147=CARTESIAN_POINT('Ctrl Pts',(-14.1209183378665,25.6651436792886,-35.1460395027545));
#49148=CARTESIAN_POINT('Ctrl Pts',(-14.0762586162872,25.9236817936235,-34.8875013884196));
#49149=CARTESIAN_POINT('Ctrl Pts',(-14.0541139337517,26.1259981746158,-34.6851850074273));
#49150=CARTESIAN_POINT('Ctrl Pts',(-14.006470104281,26.7367117564975,-34.0744714255456));
#49151=CARTESIAN_POINT('Ctrl Pts',(-14.,27.1477600534412,-33.6634231286019));
#49152=CARTESIAN_POINT('Ctrl Pts',(-14.,27.5223620986102,-33.2888210834329));
#49153=CARTESIAN_POINT('Origin',(-14.,0.,0.));
#49154=CARTESIAN_POINT('Origin',(-14.5,-12.5,-21.650635094611));
#49155=CARTESIAN_POINT('',(-14.,-12.5,-27.150635094611));
#49156=CARTESIAN_POINT('Origin',(-14.,-12.5,-21.650635094611));
#49157=CARTESIAN_POINT('',(-14.5,-12.5,-26.650635094611));
#49158=CARTESIAN_POINT('Origin',(-14.5,-12.5,-27.150635094611));
#49159=CARTESIAN_POINT('',(-14.5,-12.5,-16.650635094611));
#49160=CARTESIAN_POINT('Origin',(-14.5,-12.5,-21.650635094611));
#49161=CARTESIAN_POINT('Origin',(-14.5,-12.5,-21.650635094611));
#49162=CARTESIAN_POINT('Origin',(-14.,12.,0.));
#49163=CARTESIAN_POINT('',(-14.,31.2842712474619,-29.5269119345812));
#49164=CARTESIAN_POINT('',(-14.,-21.0416305603426,22.7989898732233));
#49165=CARTESIAN_POINT('',(-14.,-12.5,16.150635094611));
#49166=CARTESIAN_POINT('Origin',(-14.,-12.5,21.650635094611));
#49167=CARTESIAN_POINT('',(-14.,-1.55617176460037E-15,12.7071067811865));
#49168=CARTESIAN_POINT('Origin',(-14.,0.,0.));
#49169=CARTESIAN_POINT('',(-14.,25.,-5.5));
#49170=CARTESIAN_POINT('Origin',(-14.,25.,0.));
#49171=CARTESIAN_POINT('Origin',(-15.5,-12.5,-21.650635094611));
#49172=CARTESIAN_POINT('',(-15.5,-12.5,-16.650635094611));
#49173=CARTESIAN_POINT('Origin',(-14.5,-12.5,21.650635094611));
#49174=CARTESIAN_POINT('',(-14.5,-12.5,16.650635094611));
#49175=CARTESIAN_POINT('Origin',(-14.5,-12.5,16.150635094611));
#49176=CARTESIAN_POINT('',(-14.5,-12.5,26.650635094611));
#49177=CARTESIAN_POINT('Origin',(-14.5,-12.5,21.650635094611));
#49178=CARTESIAN_POINT('Origin',(-14.5,-12.5,21.650635094611));
#49179=CARTESIAN_POINT('Origin',(-15.5,-12.5,21.650635094611));
#49180=CARTESIAN_POINT('',(-15.5,-12.5,26.650635094611));
#49181=CARTESIAN_POINT('Origin',(-14.5,25.,0.));
#49182=CARTESIAN_POINT('',(-14.5,25.,-5.));
#49183=CARTESIAN_POINT('Origin',(-14.5,25.,-5.5));
#49184=CARTESIAN_POINT('',(-14.5,25.,5.));
#49185=CARTESIAN_POINT('Origin',(-14.5,25.,0.));
#49186=CARTESIAN_POINT('Origin',(-14.5,25.,0.));
#49187=CARTESIAN_POINT('Origin',(-15.5,25.,0.));
#49188=CARTESIAN_POINT('',(-15.5,25.,5.));
#49189=CARTESIAN_POINT('Origin',(-14.7071067811865,0.,0.));
#49190=CARTESIAN_POINT('',(-14.3535533905933,12.1464466094067,2.46519032881566E-31));
#49191=CARTESIAN_POINT('',(-14.3535533905933,-1.48751069612242E-15,-12.1464466094067));
#49192=CARTESIAN_POINT('Origin',(-14.3535533905933,0.,-7.43755348061208E-16));
#49193=CARTESIAN_POINT('Origin',(-14.7071067811865,-1.53080849893419E-15,
-12.5));
#49194=CARTESIAN_POINT('Origin',(-14.3535533905933,0.,-7.43755348061208E-16));
#49195=CARTESIAN_POINT('Origin',(-14.25,0.,0.));
#49196=CARTESIAN_POINT('',(-14.1464466094067,12.3535533905933,-3.0257479235772E-15));
#49197=CARTESIAN_POINT('',(-14.25,12.25,-1.50019232895551E-15));
#49198=CARTESIAN_POINT('',(-14.1464466094067,-1.5128739617886E-15,12.3535533905933));
#49199=CARTESIAN_POINT('Origin',(-14.1464466094067,0.,-7.56436980894299E-16));
#49200=CARTESIAN_POINT('Origin',(-14.1464466094067,0.,-7.56436980894299E-16));
#49201=CARTESIAN_POINT('Origin',(-14.5,0.,0.));
#49202=CARTESIAN_POINT('Origin',(-14.5,-1.55617176460037E-15,12.7071067811865));
#49203=CARTESIAN_POINT('Origin',(-83.,-29.9484575042249,-28.4786855519014));
#49204=CARTESIAN_POINT('',(-83.,-29.9484575042249,-28.4786855519014));
#49205=CARTESIAN_POINT('Origin',(-83.,-27.2236110756821,-27.2236110756821));
#49206=CARTESIAN_POINT('Origin',(-83.,-27.2236110756821,27.2236110756821));
#49207=CARTESIAN_POINT('Origin',(-83.,27.2236110756821,27.2236110756821));
#49208=CARTESIAN_POINT('Origin',(-80.,25.,0.));
#49209=CARTESIAN_POINT('Origin',(-80.,-12.5,21.650635094611));
#49210=CARTESIAN_POINT('Origin',(-80.,-12.5,-21.650635094611));
#49211=CARTESIAN_POINT('Origin',(-14.,26.1629509039022,-34.6482322781408));
#49212=CARTESIAN_POINT('',(-14.,31.2842712474619,-29.5269119345812));
#49213=CARTESIAN_POINT('Origin',(-14.,12.,0.));
#49214=CARTESIAN_POINT('Origin',(-14.,12.,0.));
#49215=CARTESIAN_POINT('Origin',(-14.,12.,0.));
#49216=CARTESIAN_POINT('Origin',(-10.,-28.2842712474619,-28.2842712474619));
#49217=CARTESIAN_POINT('Origin',(-14.,12.,0.));
#49218=CARTESIAN_POINT('Origin',(-14.,-26.1629509039023,17.6776695296637));
#49219=CARTESIAN_POINT('Origin',(-74.5,0.,0.));
#49220=CARTESIAN_POINT('',(-74.5,-42.4,-5.19250242838478E-15));
#49221=CARTESIAN_POINT('Origin',(-67.5,12.,-20.7846096908265));
#49222=CARTESIAN_POINT('',(-67.5,12.,-16.2846096908265));
#49223=CARTESIAN_POINT('Origin',(-67.5,-24.,2.93915231795365E-15));
#49224=CARTESIAN_POINT('',(-67.5,-24.,4.5));
#49225=CARTESIAN_POINT('Origin',(-67.5,12.,20.7846096908265));
#49226=CARTESIAN_POINT('',(-67.5,12.,25.2846096908265));
#65540=UNCERTAINTY_MEASURE_WITH_UNIT(LENGTH_MEASURE(0.01),#65564,
'DISTANCE_ACCURACY_VALUE',
'Maximum model space distance between geometric entities at asserted c
onnectivities');
#65550=UNCERTAINTY_MEASURE_WITH_UNIT(LENGTH_MEASURE(0.01),#65564,
'DISTANCE_ACCURACY_VALUE',
'Maximum model space distance between geometric entities at asserted c
onnectivities');
#65553=(
GEOMETRIC_REPRESENTATION_CONTEXT(3)
GLOBAL_UNCERTAINTY_ASSIGNED_CONTEXT((#65540))
GLOBAL_UNIT_ASSIGNED_CONTEXT((#65564,#65566,#65567))
REPRESENTATION_CONTEXT('','3D')
);
#65563=(
GEOMETRIC_REPRESENTATION_CONTEXT(3)
GLOBAL_UNCERTAINTY_ASSIGNED_CONTEXT((#65550))
GLOBAL_UNIT_ASSIGNED_CONTEXT((#65564,#65566,#65567))
REPRESENTATION_CONTEXT('','3D')
);
#65564=(
LENGTH_UNIT()
NAMED_UNIT(*)
SI_UNIT(.MILLI.,.METRE.)
);
#65566=(
NAMED_UNIT(*)
PLANE_ANGLE_UNIT()
SI_UNIT($,.RADIAN.)
);
#65567=(
NAMED_UNIT(*)
SI_UNIT($,.STERADIAN.)
SOLID_ANGLE_UNIT()
);
#65570=SHAPE_DEFINITION_REPRESENTATION(#65582,#65615);
#65582=PRODUCT_DEFINITION_SHAPE('',$,#65628);
#65615=SHAPE_REPRESENTATION('',(#20555),#65553);
#65625=PRODUCT_DEFINITION_CONTEXT('part definition',#65663,'design');
#65628=PRODUCT_DEFINITION('2026-10-10-05-45-22-506',
'02_Planet_Cage_Bottom_Disc_and_Notched_Top_Plate',#65640,#65625);
#65640=PRODUCT_DEFINITION_FORMATION('',$,#65667);
#65663=APPLICATION_CONTEXT(
'Core Data for Automotive Mechanical Design Process');
#65664=PRODUCT_CONTEXT('part definition',#65663,'mechanical');
#65667=PRODUCT('2026-10-10-05-45-22-506',
'02_Planet_Cage_Bottom_Disc_and_Notched_Top_Plate',$,(#65664));
#65796=COLOUR_RGB('Off White',0.89,0.88,0.83);
#65797=FILL_AREA_STYLE_COLOUR('',#65796);
#65798=FILL_AREA_STYLE('',(#65797));
#65799=SURFACE_STYLE_FILL_AREA(#65798);
#65800=SURFACE_SIDE_STYLE('',(#65799));
#65801=SURFACE_STYLE_USAGE(.BOTH.,#65800);
#65802=PRESENTATION_STYLE_ASSIGNMENT((#65801));
ENDSEC;
END-ISO-10303-21;
